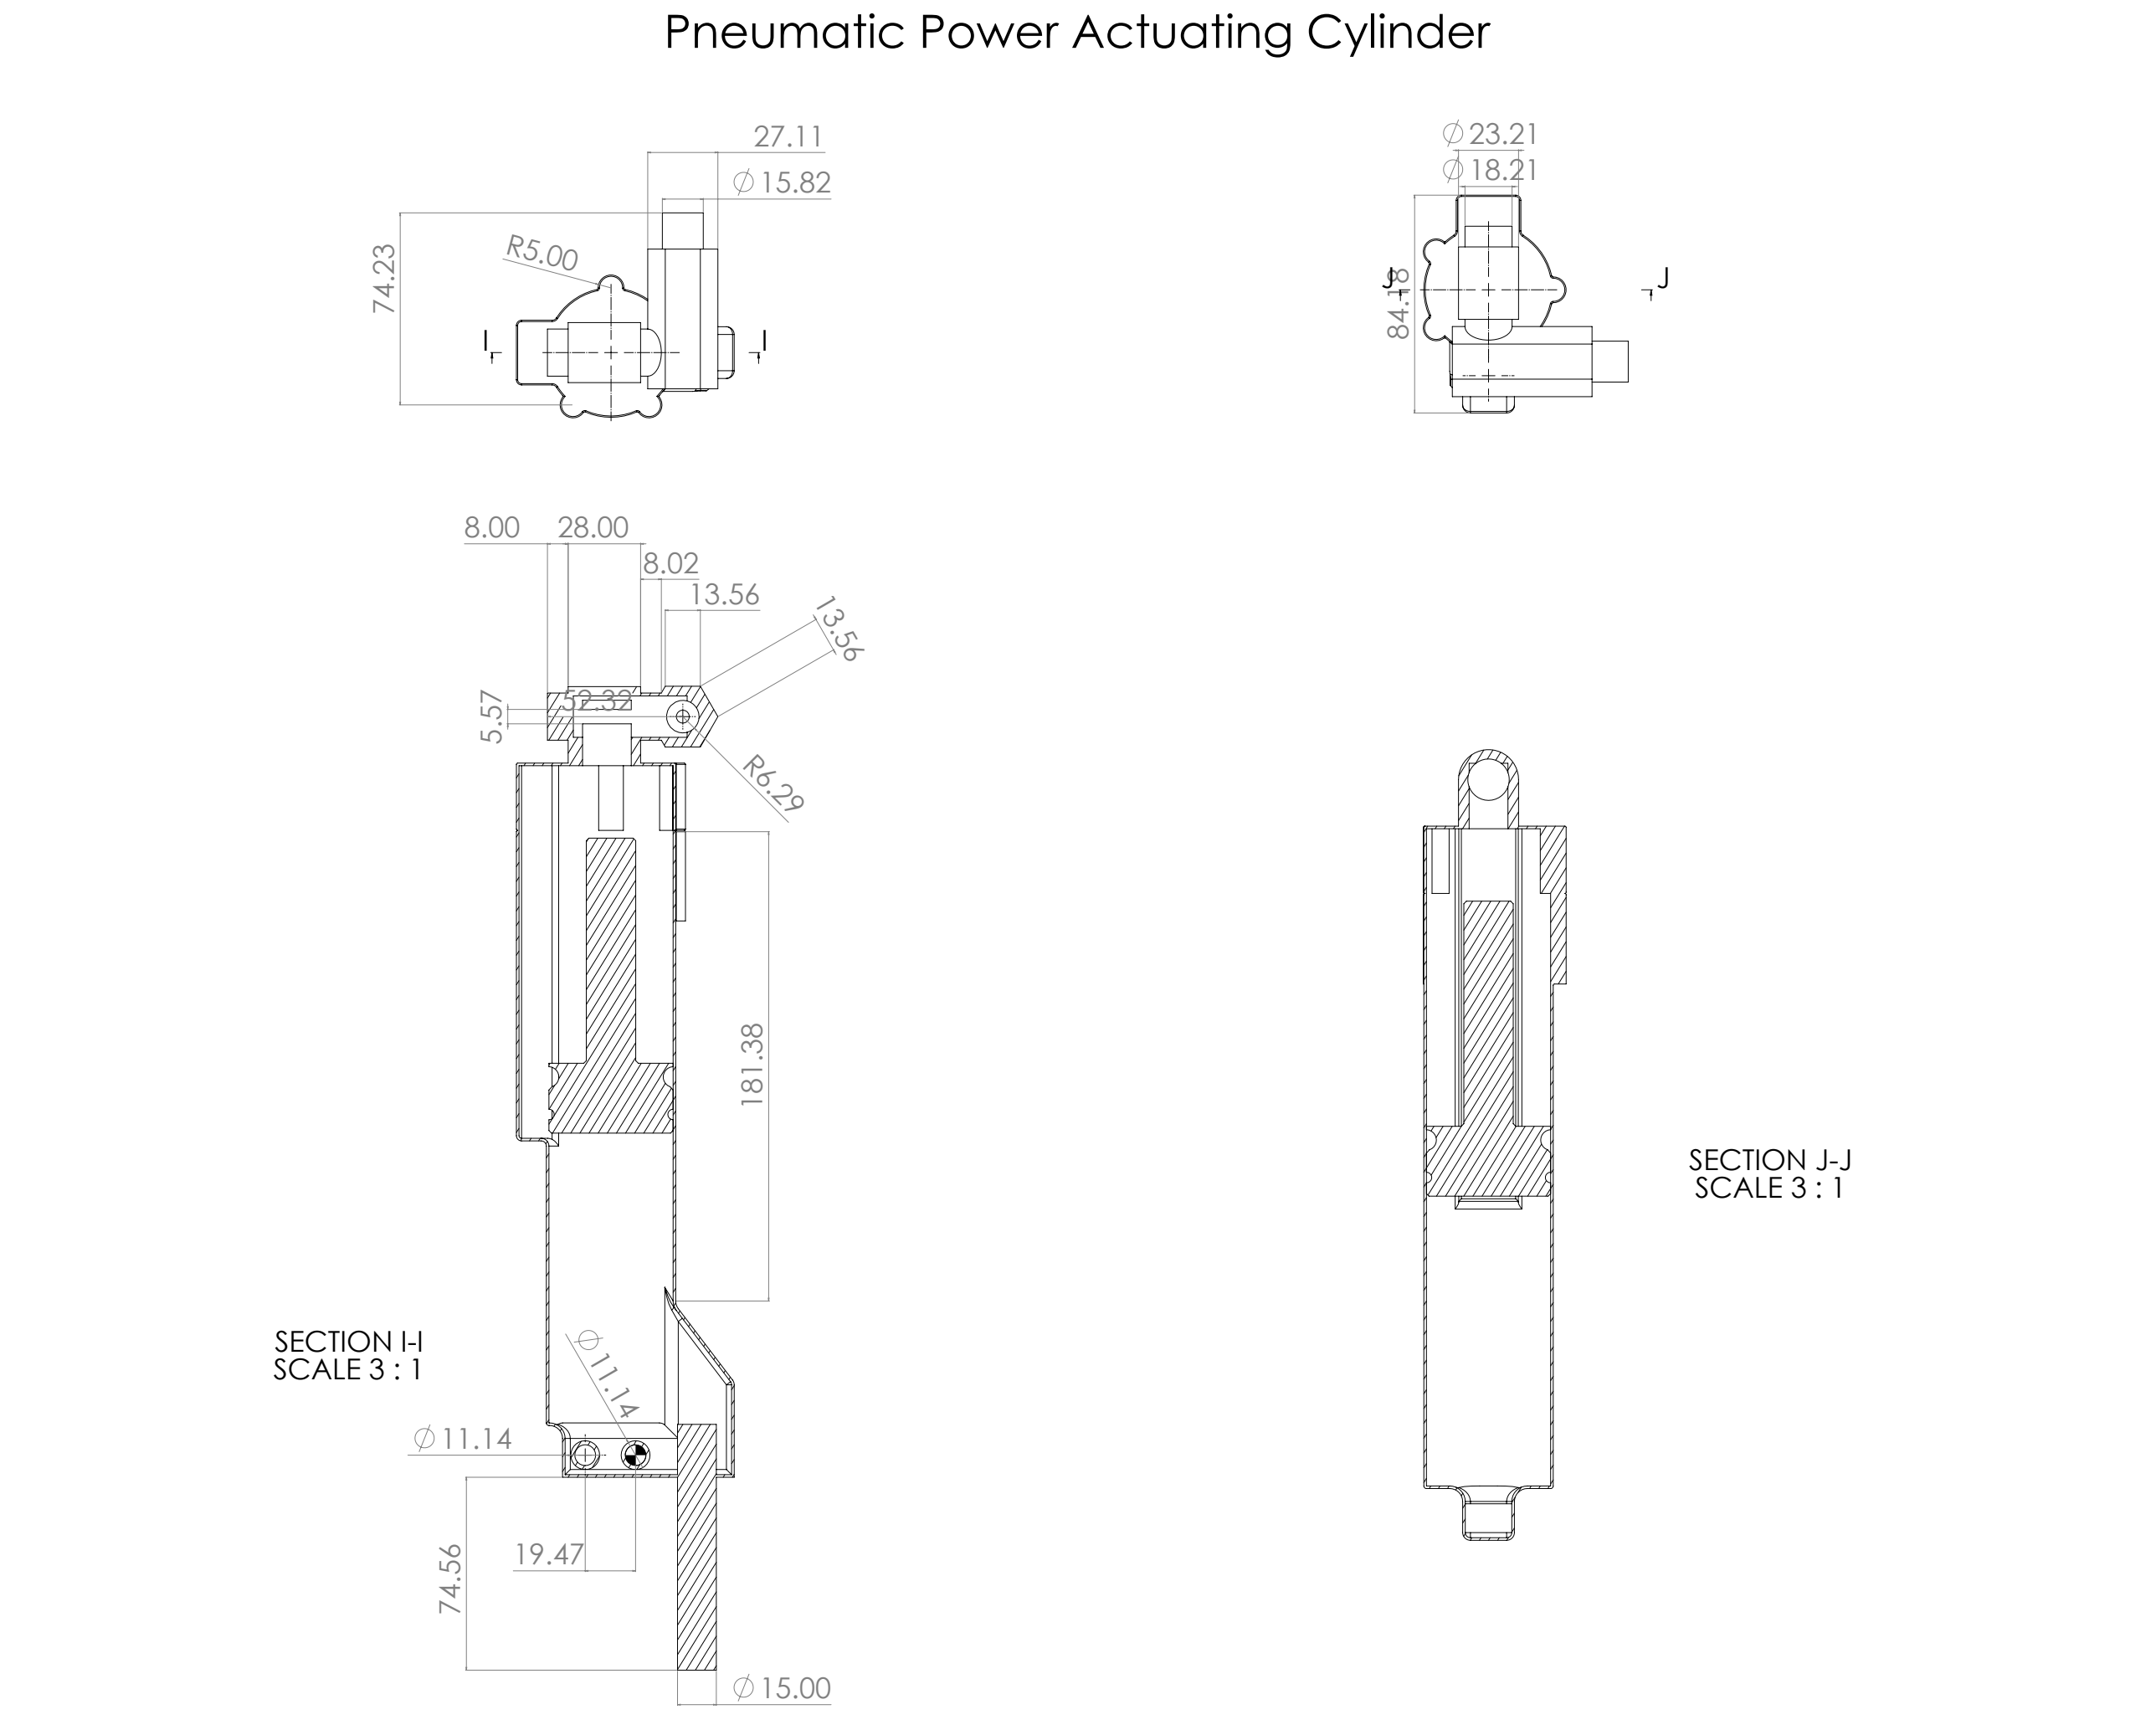
ISO-10303-21;
HEADER;
FILE_DESCRIPTION (('STEP AP214'),
    '1' );
FILE_NAME ('Pneumatic Power Actuating Cylinder.step',
    '2026-10-25T20:52:49',
    ( '' ),
    ( '' ),
    'SwSTEP 2.0',
    'SolidWorks 2025',
    '' );
FILE_SCHEMA (( 'AUTOMOTIVE_DESIGN' ));
ENDSEC;

DATA;
#13=CONICAL_SURFACE ( 'NONE', #77116, 24.00000000000001066, 0.7446590313522313265 ) ;
#19=LINE ( 'NONE', #14705, #54462 ) ;
#22=DIRECTION ( 'NONE',  ( -0.7957555401921980742, -0.6056179655966482667, 0.000000000000000000 ) ) ;
#31=VERTEX_POINT ( 'NONE', #14545 ) ;
#46=DIRECTION ( 'NONE',  ( -0.4999999999999952260, -0.8660254037844413721, 0.000000000000000000 ) ) ;
#47=FACE_OUTER_BOUND ( 'NONE', #78112, .T. ) ;
#48=EDGE_CURVE ( 'NONE', #2640, #65773, #51617, .T. ) ;
#70=VERTEX_POINT ( 'NONE', #796 ) ;
#88=EDGE_LOOP ( 'NONE', ( #36300, #74959 ) ) ;
#89=DIRECTION ( 'NONE',  ( 0.000000000000000000, -0.000000000000000000, 1.000000000000000000 ) ) ;
#92=EDGE_CURVE ( 'NONE', #64177, #39404, #21633, .T. ) ;
#124=CARTESIAN_POINT ( 'NONE',  ( 175.2296996224750103, 275.0000000000000568, 0.000000000000000000 ) ) ;
#125=CARTESIAN_POINT ( 'NONE',  ( 208.4306832106271088, 20.44233620800389772, 0.000000000000000000 ) ) ;
#133=EDGE_CURVE ( 'NONE', #3915, #71428, #47386, .T. ) ;
#135=VERTEX_POINT ( 'NONE', #13608 ) ;
#137=AXIS2_PLACEMENT_3D ( 'NONE', #66421, #57925, #65055 ) ;
#142=ORIENTED_EDGE ( 'NONE', *, *, #90775, .T. ) ;
#150=ORIENTED_EDGE ( 'NONE', *, *, #26082, .T. ) ;
#154=DIRECTION ( 'NONE',  ( 0.000000000000000000, 1.000000000000000000, 0.000000000000000000 ) ) ;
#157=CYLINDRICAL_SURFACE ( 'NONE', #21355, 0.5000000000000004441 ) ;
#172=ORIENTED_EDGE ( 'NONE', *, *, #18686, .T. ) ;
#175=ORIENTED_EDGE ( 'NONE', *, *, #24191, .T. ) ;
#200=VERTEX_POINT ( 'NONE', #71848 ) ;
#203=EDGE_CURVE ( 'NONE', #23354, #33474, #15867, .T. ) ;
#215=DIRECTION ( 'NONE',  ( 0.000000000000000000, 1.000000000000000000, 0.000000000000000000 ) ) ;
#220=CARTESIAN_POINT ( 'NONE',  ( 211.4629471475955427, 32.98517505407394168, 10.00000000000000000 ) ) ;
#226=CARTESIAN_POINT ( 'NONE',  ( 219.8344101925596021, 35.72494958537217968, 7.000000000000000000 ) ) ;
#230=CARTESIAN_POINT ( 'NONE',  ( 201.2509219215139922, 65.09645894978946501, 0.000000000000000000 ) ) ;
#233=DIRECTION ( 'NONE',  ( -0.000000000000000000, 0.000000000000000000, -1.000000000000000000 ) ) ;
#237=CARTESIAN_POINT ( 'NONE',  ( 196.8803347170859865, 73.40565171261609123, -12.49999999999998579 ) ) ;
#250=EDGE_CURVE ( 'NONE', #25460, #78927, #7415, .T. ) ;
#252=ADVANCED_FACE ( 'NONE', ( #16740 ), #65214, .F. ) ;
#266=EDGE_CURVE ( 'NONE', #10377, #27540, #29202, .T. ) ;
#272=AXIS2_PLACEMENT_3D ( 'NONE', #89516, #54022, #33648 ) ;
#291=EDGE_CURVE ( 'NONE', #59112, #73985, #48974, .T. ) ;
#307=VERTEX_POINT ( 'NONE', #19143 ) ;
#308=DIRECTION ( 'NONE',  ( 0.000000000000000000, 0.000000000000000000, -1.000000000000000000 ) ) ;
#309=CARTESIAN_POINT ( 'NONE',  ( 196.7084708347797459, 24.79057925319257194, 12.79847700770043950 ) ) ;
#315=CARTESIAN_POINT ( 'NONE',  ( 209.2565306692229683, 27.88187848093107846, 12.07105558346639462 ) ) ;
#318=DIRECTION ( 'NONE',  ( -0.000000000000000000, -1.000000000000000000, -0.000000000000000000 ) ) ;
#321=ORIENTED_EDGE ( 'NONE', *, *, #79781, .T. ) ;
#322=LINE ( 'NONE', #6506, #611 ) ;
#330=AXIS2_PLACEMENT_3D ( 'NONE', #82535, #75438, #88694 ) ;
#336=CARTESIAN_POINT ( 'NONE',  ( 197.2699694956033341, 291.3106288012165805, -7.550674042187431212 ) ) ;
#337=DIRECTION ( 'NONE',  ( -0.000000000000000000, -1.000000000000000000, -0.000000000000000000 ) ) ;
#339=AXIS2_PLACEMENT_3D ( 'NONE', #18506, #54487, #77693 ) ;
#351=CARTESIAN_POINT ( 'NONE',  ( 152.0879868122481184, 129.8824796955493355, -12.50000000000000178 ) ) ;
#359=CARTESIAN_POINT ( 'NONE',  ( 196.0143093133015384, 42.36571313990103960, 11.99999999999998934 ) ) ;
#376=ORIENTED_EDGE ( 'NONE', *, *, #4713, .F. ) ;
#377=CARTESIAN_POINT ( 'NONE',  ( 0.000000000000000000, 131.0000000000000568, -11.50000000000000000 ) ) ;
#379=CARTESIAN_POINT ( 'NONE',  ( 207.5838500149071706, 29.29481134328564451, 13.58522159759120740 ) ) ;
#390=CARTESIAN_POINT ( 'NONE',  ( 195.6182592083429768, 42.27466702580179714, 12.66657019004900953 ) ) ;
#400=CIRCLE ( 'NONE', #83570, 2.500000000000007550 ) ;
#402=CARTESIAN_POINT ( 'NONE',  ( 210.1640492649794396, 37.84931640281016030, 10.50000000000000000 ) ) ;
#403=AXIS2_PLACEMENT_3D ( 'NONE', #74243, #31178, #30232 ) ;
#404=DIRECTION ( 'NONE',  ( 0.000000000000000000, -1.000000000000000000, 0.000000000000000000 ) ) ;
#409=AXIS2_PLACEMENT_3D ( 'NONE', #74640, #9280, #38163 ) ;
#427=DIRECTION ( 'NONE',  ( -0.000000000000000000, 1.000000000000000000, -0.000000000000000000 ) ) ;
#438=( BOUNDED_SURFACE ( )  B_SPLINE_SURFACE ( 3, 2, ( 
 ( #50320, #50797, #35669 ),
 ( #87224, #29020, #21923 ),
 ( #65495, #15274, #20984 ),
 ( #42745, #29497, #79681 ) ),
 .UNSPECIFIED., .F., .F., .F. ) 
 B_SPLINE_SURFACE_WITH_KNOTS ( ( 4, 4 ),
 ( 3, 3 ),
 ( 0.000000000000000000, 0.0009274969146595095750 ),
 ( 0.000000000000000000, 1.000000000000000000 ),
 .UNSPECIFIED. ) 
 GEOMETRIC_REPRESENTATION_ITEM ( )  RATIONAL_B_SPLINE_SURFACE ( (
 ( 1.000000000000000000, 0.7691239371209215303, 1.000000000000000000),
 ( 1.000000000000000000, 0.7869877059350417481, 1.000000000000000000),
 ( 1.000000000000000000, 0.8014280003973071054, 1.000000000000000000),
 ( 1.000000000000000000, 0.8108476219622873238, 1.000000000000000000) ) ) 
 REPRESENTATION_ITEM ( '' )  SURFACE ( )  );
#443=VERTEX_POINT ( 'NONE', #78317 ) ;
#444=CARTESIAN_POINT ( 'NONE',  ( 156.6537229343953754, 214.8829733828359849, 16.96953521546817001 ) ) ;
#446=( BOUNDED_SURFACE ( )  B_SPLINE_SURFACE ( 3, 2, ( 
 ( #46429, #52604, #66380 ),
 ( #81486, #45029, #45487 ),
 ( #9515, #38403, #9987 ),
 ( #68231, #32242, #60670 ) ),
 .UNSPECIFIED., .F., .F., .F. ) 
 B_SPLINE_SURFACE_WITH_KNOTS ( ( 4, 4 ),
 ( 3, 3 ),
 ( 0.000000000000000000, 0.0009274969146595095750 ),
 ( 0.000000000000000000, 1.000000000000000000 ),
 .UNSPECIFIED. ) 
 GEOMETRIC_REPRESENTATION_ITEM ( )  RATIONAL_B_SPLINE_SURFACE ( (
 ( 1.000000000000000000, 0.7691239371209221964, 1.000000000000000000),
 ( 1.000000000000000000, 0.7869877059350496307, 1.000000000000000000),
 ( 1.000000000000000000, 0.8014280003973005551, 1.000000000000000000),
 ( 1.000000000000000000, 0.8108476219622871017, 1.000000000000000000) ) ) 
 REPRESENTATION_ITEM ( '' )  SURFACE ( )  );
#459=CARTESIAN_POINT ( 'NONE',  ( 219.8344101925596021, 0.000000000000000000, 7.000000000000000000 ) ) ;
#460=DIRECTION ( 'NONE',  ( -0.000000000000000000, -1.000000000000000000, -0.000000000000000000 ) ) ;
#470=EDGE_CURVE ( 'NONE', #443, #38673, #70143, .T. ) ;
#474=AXIS2_PLACEMENT_3D ( 'NONE', #24792, #83000, #69744 ) ;
#477=VECTOR ( 'NONE', #77768, 1000.000000000000000 ) ;
#481=AXIS2_PLACEMENT_3D ( 'NONE', #69178, #53570, #82445 ) ;
#484=VECTOR ( 'NONE', #66979, 1000.000000000000000 ) ;
#485=DIRECTION ( 'NONE',  ( 0.000000000000000000, 0.000000000000000000, -1.000000000000000000 ) ) ;
#488=DIRECTION ( 'NONE',  ( 0.000000000000000000, 1.000000000000000000, 0.000000000000000000 ) ) ;
#495=VECTOR ( 'NONE', #32367, 1000.000000000000000 ) ;
#509=AXIS2_PLACEMENT_3D ( 'NONE', #63054, #5739, #91883 ) ;
#516=CARTESIAN_POINT ( 'NONE',  ( 159.4851178187871312, 15.00000000000000000, 9.000000000000000000 ) ) ;
#527=EDGE_LOOP ( 'NONE', ( #23564, #43969, #29055, #47901 ) ) ;
#533=( NAMED_UNIT ( * ) SI_UNIT ( $, .STERADIAN. ) SOLID_ANGLE_UNIT ( ) );
#536=EDGE_LOOP ( 'NONE', ( #40735, #1250, #34787, #36151 ) ) ;
#539=VECTOR ( 'NONE', #13268, 1000.000000000000000 ) ;
#544=CARTESIAN_POINT ( 'NONE',  ( 186.6539576904058890, 276.0000000000000568, 11.60392986742922616 ) ) ;
#557=VERTEX_POINT ( 'NONE', #91558 ) ;
#558=CARTESIAN_POINT ( 'NONE',  ( 195.4431342809958210, 25.62282010151562162, 12.94565045871722653 ) ) ;
#569=DIRECTION ( 'NONE',  ( -0.7957555401921984073, -0.6056179655966479336, 0.000000000000000000 ) ) ;
#573=DIRECTION ( 'NONE',  ( -1.000000000000000000, 0.000000000000000000, 0.000000000000000000 ) ) ;
#584=EDGE_CURVE ( 'NONE', #89341, #28861, #72351, .T. ) ;
#596=DIRECTION ( 'NONE',  ( 0.000000000000000000, 0.000000000000000000, 1.000000000000000000 ) ) ;
#599=CARTESIAN_POINT ( 'NONE',  ( 195.7618616733231249, 25.17790309710478880, 14.26375052247069597 ) ) ;
#600=DIRECTION ( 'NONE',  ( 0.000000000000000000, 0.000000000000000000, -1.000000000000000000 ) ) ;
#608=EDGE_CURVE ( 'NONE', #87677, #6373, #68742, .T. ) ;
#610=VERTEX_POINT ( 'NONE', #13456 ) ;
#611=VECTOR ( 'NONE', #22104, 1000.000000000000000 ) ;
#617=AXIS2_PLACEMENT_3D ( 'NONE', #50183, #27969, #71997 ) ;
#626=AXIS2_PLACEMENT_3D ( 'NONE', #69064, #4653, #32616 ) ;
#628=VECTOR ( 'NONE', #56195, 1000.000000000000000 ) ;
#629=CARTESIAN_POINT ( 'NONE',  ( 196.6877655503061817, 294.2166337988281839, -7.999911143031724237 ) ) ;
#632=DIRECTION ( 'NONE',  ( 0.000000000000000000, 0.000000000000000000, -1.000000000000000000 ) ) ;
#634=AXIS2_PLACEMENT_3D ( 'NONE', #54460, #69150, #62530 ) ;
#645=TOROIDAL_SURFACE ( 'NONE', #5171, 1.000000000000000000, 0.5000000000000000000 ) ;
#648=ORIENTED_EDGE ( 'NONE', *, *, #78193, .T. ) ;
#676=ORIENTED_EDGE ( 'NONE', *, *, #7722, .F. ) ;
#680=ORIENTED_EDGE ( 'NONE', *, *, #88813, .T. ) ;
#684=AXIS2_PLACEMENT_3D ( 'NONE', #53670, #32361, #85228 ) ;
#690=DIRECTION ( 'NONE',  ( 1.000000000000000000, 0.000000000000000000, -0.000000000000000000 ) ) ;
#693=CIRCLE ( 'NONE', #79306, 1.999999999999988454 ) ;
#696=CARTESIAN_POINT ( 'NONE',  ( 193.9646936176702070, 20.00000000000000000, -15.00000000000000000 ) ) ;
#698=AXIS2_PLACEMENT_3D ( 'NONE', #32787, #46964, #39859 ) ;
#703=CARTESIAN_POINT ( 'NONE',  ( 154.5739546116847407, 19.95362051968588801, 14.09237539257051530 ) ) ;
#706=CARTESIAN_POINT ( 'NONE',  ( 151.2975037349263800, 130.0000000000000568, 12.50000000000000000 ) ) ;
#709=CIRCLE ( 'NONE', #58172, 7.500000000000012434 ) ;
#733=ADVANCED_FACE ( 'NONE', ( #49428 ), #55131, .T. ) ;
#742=EDGE_CURVE ( 'NONE', #34447, #93704, #90736, .T. ) ;
#760=AXIS2_PLACEMENT_3D ( 'NONE', #30344, #9477, #21860 ) ;
#784=CARTESIAN_POINT ( 'NONE',  ( 165.2494399300530290, 8.542400036368780647, 9.000000000000001776 ) ) ;
#793=EDGE_CURVE ( 'NONE', #79410, #22214, #70290, .T. ) ;
#794=DIRECTION ( 'NONE',  ( 0.000000000000000000, 0.000000000000000000, 1.000000000000000000 ) ) ;
#796=CARTESIAN_POINT ( 'NONE',  ( 196.8702642586143270, 40.96915988761478644, 12.42857142857141994 ) ) ;
#800=CARTESIAN_POINT ( 'NONE',  ( 197.0850307134193713, 40.94976125279444545, 10.55987713565813024 ) ) ;
#813=LINE ( 'NONE', #31437, #58161 ) ;
#814=CARTESIAN_POINT ( 'NONE',  ( 201.2104617360081704, 25.32700003806615996, 9.000000000000001776 ) ) ;
#822=DIRECTION ( 'NONE',  ( 0.000000000000000000, 0.000000000000000000, 1.000000000000000000 ) ) ;
#823=DIRECTION ( 'NONE',  ( 1.000000000000000000, 0.000000000000000000, 0.000000000000000000 ) ) ;
#830=DIRECTION ( 'NONE',  ( -0.000000000000000000, -1.000000000000000000, -0.000000000000000000 ) ) ;
#839=PLANE ( 'NONE',  #10916 ) ;
#841=AXIS2_PLACEMENT_3D ( 'NONE', #42069, #7056, #77614 ) ;
#854=CARTESIAN_POINT ( 'NONE',  ( 199.7111327665421072, 66.88064514420912587, 10.01633191836423364 ) ) ;
#856=FACE_OUTER_BOUND ( 'NONE', #12534, .T. ) ;
#867=EDGE_LOOP ( 'NONE', ( #63453, #67407, #86830, #3763 ) ) ;
#878=DIRECTION ( 'NONE',  ( 0.000000000000000000, 0.000000000000000000, -1.000000000000000000 ) ) ;
#882=ORIENTED_EDGE ( 'NONE', *, *, #83721, .T. ) ;
#899=EDGE_CURVE ( 'NONE', #67369, #66900, #57022, .T. ) ;
#900=CARTESIAN_POINT ( 'NONE',  ( 210.2448042458983366, 0.01303144969186963500, -7.291618491801075130 ) ) ;
#907=EDGE_CURVE ( 'NONE', #12419, #67382, #86299, .T. ) ;
#909=EDGE_CURVE ( 'NONE', #57029, #39232, #24135, .T. ) ;
#915=ORIENTED_EDGE ( 'NONE', *, *, #72851, .F. ) ;
#916=CARTESIAN_POINT ( 'NONE',  ( 197.9834613664963001, 18.87240044341482914, -11.15593255764641967 ) ) ;
#930=DIRECTION ( 'NONE',  ( 0.000000000000000000, 1.000000000000000000, 0.000000000000000000 ) ) ;
#938=CARTESIAN_POINT ( 'NONE',  ( 140.6539576904058606, 249.5000000000000568, 12.50000000000000000 ) ) ;
#942=DIRECTION ( 'NONE',  ( 0.000000000000000000, 0.000000000000000000, 1.000000000000000000 ) ) ;
#964=ORIENTED_EDGE ( 'NONE', *, *, #41918, .T. ) ;
#965=PLANE ( 'NONE',  #3028 ) ;
#967=CARTESIAN_POINT ( 'NONE',  ( 175.2296996224750103, 214.5000000000000568, 0.000000000000000000 ) ) ;
#979=CARTESIAN_POINT ( 'NONE',  ( 201.8074164582889125, 62.71404347880360319, -8.782170572880787063 ) ) ;
#980=CARTESIAN_POINT ( 'NONE',  ( 160.5350683151633291, 250.5000000000000568, 20.22542485937379908 ) ) ;
#983=CARTESIAN_POINT ( 'NONE',  ( 193.9153122143737562, 214.9910457053126720, 17.21343741151142481 ) ) ;
#999=EDGE_CURVE ( 'NONE', #46709, #71428, #37410, .T. ) ;
#1003=ORIENTED_EDGE ( 'NONE', *, *, #5970, .F. ) ;
#1009=CARTESIAN_POINT ( 'NONE',  ( 165.0704140682094589, 2.965303559109564890, 10.00000000000000000 ) ) ;
#1014=ADVANCED_FACE ( 'NONE', ( #2837 ), #75763, .T. ) ;
#1017=B_SPLINE_CURVE_WITH_KNOTS ( 'NONE', 3,
 ( #237, #56627, #85477, #93503, #42373, #57546, #29117, #35287 ),
 .UNSPECIFIED., .F., .F.,
 ( 4, 2, 2, 4 ),
 ( -1.794524598959325299E-05, 0.004652435581272471032, 0.006987625994903502377, 0.009322816408534533722 ),
 .UNSPECIFIED. ) ;
#1023=VERTEX_POINT ( 'NONE', #983 ) ;
#1024=CARTESIAN_POINT ( 'NONE',  ( 195.7077576554793836, 26.39544325298913918, 13.66612345222623404 ) ) ;
#1047=DIRECTION ( 'NONE',  ( -1.000000000000000000, 0.000000000000000000, 0.000000000000000000 ) ) ;
#1055=CARTESIAN_POINT ( 'NONE',  ( 198.6746746775679355, 25.20017525016920246, 11.14960445189099225 ) ) ;
#1058=CARTESIAN_POINT ( 'NONE',  ( 195.0811277904325323, 27.27788670632333989, 15.19607843137264602 ) ) ;
#1059=CARTESIAN_POINT ( 'NONE',  ( 156.4851178187871312, 0.000000000000000000, -7.000000000000000888 ) ) ;
#1068=EDGE_LOOP ( 'NONE', ( #54068, #62858, #68288, #37860 ) ) ;
#1069=CARTESIAN_POINT ( 'NONE',  ( 175.2296996224749250, 276.0000000000000568, -24.99999999999999289 ) ) ;
#1072=DIRECTION ( 'NONE',  ( 0.000000000000000000, 1.000000000000000000, 0.000000000000000000 ) ) ;
#1084=CARTESIAN_POINT ( 'NONE',  ( 201.9208557708175249, 300.1658636863270431, -5.053462443409009630 ) ) ;
#1087=CARTESIAN_POINT ( 'NONE',  ( 175.2296996224750103, 250.5000000000000568, 0.000000000000000000 ) ) ;
#1101=ORIENTED_EDGE ( 'NONE', *, *, #12784, .T. ) ;
#1104=EDGE_LOOP ( 'NONE', ( #42911, #32160, #59830, #16502 ) ) ;
#1109=EDGE_CURVE ( 'NONE', #44168, #80534, #22737, .T. ) ;
#1131=ORIENTED_EDGE ( 'NONE', *, *, #65065, .F. ) ;
#1134=ADVANCED_FACE ( 'NONE', ( #58749 ), #55660, .T. ) ;
#1135=VERTEX_POINT ( 'NONE', #59209 ) ;
#1146=DIRECTION ( 'NONE',  ( 0.000000000000000000, 1.000000000000000000, 0.000000000000000000 ) ) ;
#1151=CARTESIAN_POINT ( 'NONE',  ( 140.6539576904058606, 275.0000000000000568, -10.49999999999999822 ) ) ;
#1157=DIRECTION ( 'NONE',  ( -0.000000000000000000, -0.000000000000000000, -1.000000000000000000 ) ) ;
#1160=CARTESIAN_POINT ( 'NONE',  ( 194.7173632872394649, 19.95192844427760193, 14.18452691302933033 ) ) ;
#1162=LINE ( 'NONE', #80229, #54661 ) ;
#1168=CARTESIAN_POINT ( 'NONE',  ( 180.2288731078812702, 214.9910457053126720, -24.90909090909092782 ) ) ;
#1176=VERTEX_POINT ( 'NONE', #23212 ) ;
#1180=CARTESIAN_POINT ( 'NONE',  ( 169.8384340989974532, 214.5000000000000568, -24.41176470588233727 ) ) ;
#1197=ADVANCED_FACE ( 'NONE', ( #88535 ), #31719, .T. ) ;
#1219=EDGE_CURVE ( 'NONE', #20475, #31737, #23684, .T. ) ;
#1237=ORIENTED_EDGE ( 'NONE', *, *, #74557, .F. ) ;
#1244=CARTESIAN_POINT ( 'NONE',  ( 209.0514133012270861, 29.56734752687822620, 14.78224109794551033 ) ) ;
#1250=ORIENTED_EDGE ( 'NONE', *, *, #18442, .F. ) ;
#1251=CARTESIAN_POINT ( 'NONE',  ( 152.4536156746142410, 250.0000000000000568, -11.99999999999999112 ) ) ;
#1264=CARTESIAN_POINT ( 'NONE',  ( 196.7806748523260012, 250.5000000000000568, -12.67104836398113399 ) ) ;
#1272=CARTESIAN_POINT ( 'NONE',  ( 193.9646936176702070, 21.00000000000000000, -15.00000000000000000 ) ) ;
#1273=CARTESIAN_POINT ( 'NONE',  ( 175.2296996224749250, 250.5000000000000568, -24.99999999999999289 ) ) ;
#1280=LINE ( 'NONE', #2221, #36777 ) ;
#1287=CARTESIAN_POINT ( 'NONE',  ( 196.5738014817347050, 41.11195847892590649, 11.18394375856346556 ) ) ;
#1290=FACE_OUTER_BOUND ( 'NONE', #52683, .T. ) ;
#1303=ORIENTED_EDGE ( 'NONE', *, *, #24438, .F. ) ;
#1306=DIRECTION ( 'NONE',  ( 0.000000000000000000, 0.000000000000000000, 1.000000000000000000 ) ) ;
#1326=CARTESIAN_POINT ( 'NONE',  ( 152.4536156746142410, 275.0000000000000568, -11.50000000000000355 ) ) ;
#1331=EDGE_LOOP ( 'NONE', ( #25766, #6601, #5992, #88463 ) ) ;
#1347=DIRECTION ( 'NONE',  ( 0.000000000000000000, 1.000000000000000000, 0.000000000000000000 ) ) ;
#1349=DIRECTION ( 'NONE',  ( 0.000000000000000000, 0.000000000000000000, -1.000000000000000000 ) ) ;
#1361=ORIENTED_EDGE ( 'NONE', *, *, #30936, .F. ) ;
#1367=EDGE_CURVE ( 'NONE', #81908, #50747, #52092, .T. ) ;
#1378=CARTESIAN_POINT ( 'NONE',  ( 156.4947056272798136, 19.99999999999999645, -15.00000000000000711 ) ) ;
#1386=CARTESIAN_POINT ( 'NONE',  ( 204.7786681169002350, 32.98517505407394168, 10.00000000000000000 ) ) ;
#1403=CARTESIAN_POINT ( 'NONE',  ( 197.8477145984406889, 64.61450673763175701, -7.741079165001063522 ) ) ;
#1410=VECTOR ( 'NONE', #49510, 1000.000000000000000 ) ;
#1413=ORIENTED_EDGE ( 'NONE', *, *, #64946, .T. ) ;
#1414=DIRECTION ( 'NONE',  ( 0.000000000000000000, 0.000000000000000000, 1.000000000000000000 ) ) ;
#1417=DIRECTION ( 'NONE',  ( 0.000000000000000000, 1.000000000000000000, 0.000000000000000000 ) ) ;
#1421=ADVANCED_FACE ( 'NONE', ( #16119 ), #24606, .F. ) ;
#1431=DIRECTION ( 'NONE',  ( 0.000000000000000000, 0.000000000000000000, 1.000000000000000000 ) ) ;
#1443=VERTEX_POINT ( 'NONE', #82370 ) ;
#1450=ORIENTED_EDGE ( 'NONE', *, *, #68389, .T. ) ;
#1451=VERTEX_POINT ( 'NONE', #73871 ) ;
#1470=VERTEX_POINT ( 'NONE', #17520 ) ;
#1476=AXIS2_PLACEMENT_3D ( 'NONE', #8968, #1414, #22268 ) ;
#1482=B_SPLINE_CURVE_WITH_KNOTS ( 'NONE', 3,
 ( #10660, #39516, #23489, #52356, #74608, #10190, #31066, #9737, #82632, #82167 ),
 .UNSPECIFIED., .F., .F.,
 ( 4, 2, 2, 2, 4 ),
 ( -1.872485596898890801E-05, 0.002374103250644057396, 0.004766931357257103534, 0.007159759463870149672, 0.009552587570483194943 ),
 .UNSPECIFIED. ) ;
#1496=CARTESIAN_POINT ( 'NONE',  ( 194.3475392320528385, 26.68743749201679805, 14.50895590765962240 ) ) ;
#1502=DIRECTION ( 'NONE',  ( -0.000000000000000000, 0.000000000000000000, -1.000000000000000000 ) ) ;
#1508=LINE ( 'NONE', #59764, #45796 ) ;
#1518=CARTESIAN_POINT ( 'NONE',  ( 200.4551663813218170, 64.49084098419280053, 0.000000000000000000 ) ) ;
#1524=EDGE_CURVE ( 'NONE', #92711, #90042, #92671, .T. ) ;
#1533=( BOUNDED_CURVE ( )  B_SPLINE_CURVE ( 3, ( #22098, #93125, #56710, #43398 ),
 .UNSPECIFIED., .F., .F. ) 
 B_SPLINE_CURVE_WITH_KNOTS ( ( 4, 4 ),
 ( 1.570796326794895004, 2.004620063563923082 ),
 .UNSPECIFIED. ) 
 CURVE ( )  GEOMETRIC_REPRESENTATION_ITEM ( )  RATIONAL_B_SPLINE_CURVE ( ( 1.000000000000000000, 0.9843778111405747655, 0.9843778111405747655, 1.000000000000000000 ) ) 
 REPRESENTATION_ITEM ( '' )  );
#1535=CARTESIAN_POINT ( 'NONE',  ( 155.8055003384388897, 17.52828139914081618, 8.087387968559804463 ) ) ;
#1536=DIRECTION ( 'NONE',  ( -1.000000000000000000, 0.000000000000000000, 0.000000000000000000 ) ) ;
#1537=AXIS2_PLACEMENT_3D ( 'NONE', #11772, #17497, #68618 ) ;
#1542=AXIS2_PLACEMENT_3D ( 'NONE', #35545, #85251, #20398 ) ;
#1554=ORIENTED_EDGE ( 'NONE', *, *, #13930, .F. ) ;
#1557=EDGE_LOOP ( 'NONE', ( #41598, #34259, #35254, #4428 ) ) ;
#1567=VERTEX_POINT ( 'NONE', #67252 ) ;
#1585=VERTEX_POINT ( 'NONE', #11336 ) ;
#1586=CARTESIAN_POINT ( 'NONE',  ( 158.3977298502311157, 18.03393767897202693, 9.815540976419818264 ) ) ;
#1609=CIRCLE ( 'NONE', #49999, 0.5000000000000004441 ) ;
#1612=CYLINDRICAL_SURFACE ( 'NONE', #21692, 24.00000000000000355 ) ;
#1616=CARTESIAN_POINT ( 'NONE',  ( 195.3965999132940397, 19.72393862741004611, 13.34571198792791868 ) ) ;
#1618=DIRECTION ( 'NONE',  ( -0.000000000000000000, -1.000000000000000000, 0.000000000000000000 ) ) ;
#1620=DIRECTION ( 'NONE',  ( -1.000000000000000000, 0.000000000000000000, -0.000000000000000000 ) ) ;
#1624=CARTESIAN_POINT ( 'NONE',  ( 188.2019740231993410, 44.81720372851549428, 10.50000000000000000 ) ) ;
#1631=ADVANCED_FACE ( 'NONE', ( #76207 ), #91321, .T. ) ;
#1634=ORIENTED_EDGE ( 'NONE', *, *, #50049, .T. ) ;
#1638=DIRECTION ( 'NONE',  ( -1.000000000000000000, 0.000000000000000000, 0.000000000000000000 ) ) ;
#1641=CARTESIAN_POINT ( 'NONE',  ( 208.6470931340251695, 37.28147638844021117, 12.02381566707520300 ) ) ;
#1670=EDGE_LOOP ( 'NONE', ( #9116, #72630, #35817, #56102 ) ) ;
#1671=EDGE_CURVE ( 'NONE', #70513, #36421, #78434, .T. ) ;
#1682=CIRCLE ( 'NONE', #34945, 24.50000000000000355 ) ;
#1695=CARTESIAN_POINT ( 'NONE',  ( 196.8803347170859865, 20.19615242270661426, 12.49999999999999289 ) ) ;
#1700=CYLINDRICAL_SURFACE ( 'NONE', #14009, 2.000000000000000888 ) ;
#1701=DIRECTION ( 'NONE',  ( -0.000000000000000000, -1.000000000000000000, -0.000000000000000000 ) ) ;
#1707=CARTESIAN_POINT ( 'NONE',  ( 208.6208076322478746, 32.98517505407394168, 10.00000000000000000 ) ) ;
#1730=CARTESIAN_POINT ( 'NONE',  ( 209.7513585654923816, 282.2246705312486483, -40.00000000000000711 ) ) ;
#1735=CARTESIAN_POINT ( 'NONE',  ( 199.0061125298537377, 250.5000000000000568, -7.725424859374024678 ) ) ;
#1737=EDGE_CURVE ( 'NONE', #23799, #17402, #5377, .T. ) ;
#1739=FACE_OUTER_BOUND ( 'NONE', #32338, .T. ) ;
#1746=CARTESIAN_POINT ( 'NONE',  ( 197.3748232817348764, 249.5000000000000568, -12.45182892472558756 ) ) ;
#1749=DIRECTION ( 'NONE',  ( 0.000000000000000000, 0.000000000000000000, 1.000000000000000000 ) ) ;
#1751=AXIS2_PLACEMENT_3D ( 'NONE', #1735, #81729, #16877 ) ;
#1761=EDGE_CURVE ( 'NONE', #65093, #10127, #91797, .T. ) ;
#1762=EDGE_CURVE ( 'NONE', #5855, #73562, #18431, .T. ) ;
#1763=B_SPLINE_CURVE_WITH_KNOTS ( 'NONE', 3,
 ( #706, #29590, #44697, #7785, #81151, #43765 ),
 .UNSPECIFIED., .F., .F.,
 ( 4, 2, 4 ),
 ( 0.000000000000000000, 0.0005961816168538936920, 0.001192363233707787384 ),
 .UNSPECIFIED. ) ;
#1769=DIRECTION ( 'NONE',  ( 0.000000000000000000, 0.000000000000000000, 1.000000000000000000 ) ) ;
#1778=ORIENTED_EDGE ( 'NONE', *, *, #19590, .F. ) ;
#1783=EDGE_CURVE ( 'NONE', #27568, #44950, #62480, .T. ) ;
#1790=DIRECTION ( 'NONE',  ( -0.000000000000000000, -0.000000000000000000, -1.000000000000000000 ) ) ;
#1791=DIRECTION ( 'NONE',  ( 0.000000000000000000, 0.000000000000000000, -1.000000000000000000 ) ) ;
#1795=ORIENTED_EDGE ( 'NONE', *, *, #45672, .T. ) ;
#1809=DIRECTION ( 'NONE',  ( -0.7453559924999200170, 0.000000000000000000, -0.6666666666666777319 ) ) ;
#1812=FACE_OUTER_BOUND ( 'NONE', #17774, .T. ) ;
#1813=CIRCLE ( 'NONE', #47133, 7.999911143031724237 ) ;
#1814=CARTESIAN_POINT ( 'NONE',  ( 210.6911334572095598, 1.334076891925523281E-16, -7.166221634559009956 ) ) ;
#1815=VECTOR ( 'NONE', #7572, 1000.000000000000000 ) ;
#1823=CARTESIAN_POINT ( 'NONE',  ( 201.2104617360081704, 15.00000000000000000, 10.00000000000000000 ) ) ;
#1827=ORIENTED_EDGE ( 'NONE', *, *, #52934, .F. ) ;
#1828=VERTEX_POINT ( 'NONE', #68169 ) ;
#1829=CARTESIAN_POINT ( 'NONE',  ( 196.8803347170860150, 20.19615242270657163, -12.49999999999990941 ) ) ;
#1831=ADVANCED_FACE ( 'NONE', ( #40648 ), #55492, .T. ) ;
#1844=CARTESIAN_POINT ( 'NONE',  ( 197.1123855246549113, 19.09807621135331601, -10.09807621135331246 ) ) ;
#1879=FACE_OUTER_BOUND ( 'NONE', #84407, .T. ) ;
#1883=CARTESIAN_POINT ( 'NONE',  ( 175.2296996224750103, 275.0000000000000568, 0.000000000000000000 ) ) ;
#1886=MECHANICAL_DESIGN_GEOMETRIC_PRESENTATION_REPRESENTATION('',(#88040),#32101);
#1889=AXIS2_PLACEMENT_3D ( 'NONE', #75536, #46175, #8792 ) ;
#1892=ADVANCED_FACE ( 'NONE', ( #39254 ), #63083, .T. ) ;
#1895=ORIENTED_EDGE ( 'NONE', *, *, #3875, .T. ) ;
#1899=EDGE_CURVE ( 'NONE', #23580, #14315, #57008, .T. ) ;
#1903=DIRECTION ( 'NONE',  ( 0.000000000000000000, 0.000000000000000000, 1.000000000000000000 ) ) ;
#1937=DIRECTION ( 'NONE',  ( -1.000000000000000000, 0.000000000000000000, 0.000000000000000000 ) ) ;
#1944=AXIS2_PLACEMENT_3D ( 'NONE', #34809, #13512, #28646 ) ;
#1952=EDGE_CURVE ( 'NONE', #64179, #15573, #34061, .T. ) ;
#1954=EDGE_CURVE ( 'NONE', #44950, #76130, #84195, .T. ) ;
#1955=AXIS2_PLACEMENT_3D ( 'NONE', #93178, #10133, #31007 ) ;
#1966=DIRECTION ( 'NONE',  ( -0.000000000000000000, -1.000000000000000000, -0.000000000000000000 ) ) ;
#1972=CARTESIAN_POINT ( 'NONE',  ( 165.2494399300530290, 8.542400036368780647, 10.00000000000000000 ) ) ;
#1978=CARTESIAN_POINT ( 'NONE',  ( 158.6539576904058606, 276.0000000000000568, -11.60392986742922439 ) ) ;
#1979=CARTESIAN_POINT ( 'NONE',  ( 219.8344101925596021, 3.000000000000000000, -9.000000000000001776 ) ) ;
#1988=VERTEX_POINT ( 'NONE', #39717 ) ;
#1992=DIRECTION ( 'NONE',  ( -0.000000000000000000, -1.000000000000000000, -0.000000000000000000 ) ) ;
#2003=AXIS2_PLACEMENT_3D ( 'NONE', #71866, #337, #86031 ) ;
#2005=CARTESIAN_POINT ( 'NONE',  ( 156.3466120839441089, 16.19322481500840993, 7.221609175748572973 ) ) ;
#2009=VECTOR ( 'NONE', #39902, 1000.000000000000000 ) ;
#2023=EDGE_CURVE ( 'NONE', #3915, #44324, #61085, .T. ) ;
#2040=ORIENTED_EDGE ( 'NONE', *, *, #56462, .T. ) ;
#2051=ORIENTED_EDGE ( 'NONE', *, *, #5681, .F. ) ;
#2055=VECTOR ( 'NONE', #50209, 1000.000000000000000 ) ;
#2059=ORIENTED_EDGE ( 'NONE', *, *, #38620, .T. ) ;
#2060=CARTESIAN_POINT ( 'NONE',  ( 157.4471379844591752, 15.78783268421836183, 9.037979834337678042 ) ) ;
#2063=VERTEX_POINT ( 'NONE', #61546 ) ;
#2080=CARTESIAN_POINT ( 'NONE',  ( 207.8229135343381131, 36.37371623600424186, 14.86900317285956064 ) ) ;
#2088=DIRECTION ( 'NONE',  ( 0.000000000000000000, 1.000000000000000000, 0.000000000000000000 ) ) ;
#2090=AXIS2_PLACEMENT_3D ( 'NONE', #30133, #58563, #59492 ) ;
#2094=DIRECTION ( 'NONE',  ( 0.000000000000000000, 0.000000000000000000, 1.000000000000000000 ) ) ;
#2110=AXIS2_PLACEMENT_3D ( 'NONE', #15492, #87900, #51930 ) ;
#2114=CYLINDRICAL_SURFACE ( 'NONE', #34879, 3.000000000000000888 ) ;
#2117=CARTESIAN_POINT ( 'NONE',  ( 170.4537599243631405, 250.0000000000000568, -23.51999999999999602 ) ) ;
#2121=VECTOR ( 'NONE', #87459, 1000.000000000000000 ) ;
#2135=DIRECTION ( 'NONE',  ( 0.000000000000000000, 1.000000000000000000, -0.000000000000000000 ) ) ;
#2147=ORIENTED_EDGE ( 'NONE', *, *, #33369, .F. ) ;
#2155=DIRECTION ( 'NONE',  ( 0.000000000000000000, 0.000000000000000000, 1.000000000000000000 ) ) ;
#2156=CIRCLE ( 'NONE', #21833, 25.50000000000000355 ) ;
#2164=CIRCLE ( 'NONE', #17308, 0.4999999999999922839 ) ;
#2170=VERTEX_POINT ( 'NONE', #46370 ) ;
#2180=DIRECTION ( 'NONE',  ( 0.000000000000000000, 1.000000000000000000, 0.000000000000000000 ) ) ;
#2181=CARTESIAN_POINT ( 'NONE',  ( 155.7140808774800007, 21.00000000000000000, 15.62500000000000000 ) ) ;
#2184=AXIS2_PLACEMENT_3D ( 'NONE', #63537, #78191, #92363 ) ;
#2188=CARTESIAN_POINT ( 'NONE',  ( 200.1258905644044432, 39.98499045671346153, 10.50000000000114753 ) ) ;
#2203=FACE_OUTER_BOUND ( 'NONE', #28399, .T. ) ;
#2212=CARTESIAN_POINT ( 'NONE',  ( 175.2296996224750103, 142.2541816238762920, 0.000000000000000000 ) ) ;
#2213=DIRECTION ( 'NONE',  ( 0.000000000000000000, 1.000000000000000000, 0.000000000000000000 ) ) ;
#2221=CARTESIAN_POINT ( 'NONE',  ( 201.2104617360081704, 0.000000000000000000, 10.00000000000000000 ) ) ;
#2232=CARTESIAN_POINT ( 'NONE',  ( 200.6103193995254230, 275.5000000000000568, -2.464576988612312114 ) ) ;
#2242=CIRCLE ( 'NONE', #50642, 2.999999999999999556 ) ;
#2247=CARTESIAN_POINT ( 'NONE',  ( 198.0748556046041244, 67.35408903922716206, 11.09505092893674139 ) ) ;
#2259=AXIS2_PLACEMENT_3D ( 'NONE', #79399, #14535, #43390 ) ;
#2261=ORIENTED_EDGE ( 'NONE', *, *, #4649, .T. ) ;
#2262=DIRECTION ( 'NONE',  ( -0.000000000000000000, -1.000000000000000000, -0.000000000000000000 ) ) ;
#2294=CARTESIAN_POINT ( 'NONE',  ( 180.2262870919856823, 214.9642003054772488, -24.76688354601323283 ) ) ;
#2303=CARTESIAN_POINT ( 'NONE',  ( 207.3561592308186334, 36.17070937851315193, 14.95737379494689456 ) ) ;
#2308=VERTEX_POINT ( 'NONE', #13233 ) ;
#2309=CARTESIAN_POINT ( 'NONE',  ( 199.1517898866434848, 16.71555987447352720, -10.28330198088200120 ) ) ;
#2312=ADVANCED_FACE ( 'NONE', ( #65297 ), #79334, .T. ) ;
#2313=ADVANCED_FACE ( 'NONE', ( #57710 ), #13689, .T. ) ;
#2345=B_SPLINE_CURVE_WITH_KNOTS ( 'NONE', 3,
 ( #61003, #39638, #53881, #91241, #19759, #70446, #11261, #68563, #40573, #69029, #83679, #25010, #91717, #55294, #18841, #47698, #11719, #89848 ),
 .UNSPECIFIED., .F., .F.,
 ( 4, 2, 2, 2, 2, 2, 2, 2, 4 ),
 ( 0.000000000000000000, 0.0005979543124017953383, 0.001195908624803590677, 0.001793862937205386015, 0.002391817249607181353, 0.002989771562008976691, 0.003587725874410772030, 0.004185680186812567802, 0.004783634499214362706 ),
 .UNSPECIFIED. ) ;
#2363=ORIENTED_EDGE ( 'NONE', *, *, #88613, .F. ) ;
#2364=CARTESIAN_POINT ( 'NONE',  ( 200.2349812190172713, 66.43136063442170780, -7.741079165001061746 ) ) ;
#2367=DIRECTION ( 'NONE',  ( 0.000000000000000000, 0.000000000000000000, 1.000000000000000000 ) ) ;
#2375=ORIENTED_EDGE ( 'NONE', *, *, #74127, .F. ) ;
#2378=CARTESIAN_POINT ( 'NONE',  ( 214.2238915819278589, 32.98517505407394168, 9.000000000000001776 ) ) ;
#2380=CARTESIAN_POINT ( 'NONE',  ( 196.0742305401642511, 73.02742819586271139, 11.89621339062204264 ) ) ;
#2383=CARTESIAN_POINT ( 'NONE',  ( 175.2296996224750103, 247.0000000000001137, -8.550761578869359170 ) ) ;
#2384=PRODUCT_DEFINITION_FORMATION_WITH_SPECIFIED_SOURCE ( 'ANY', '', #44255, .NOT_KNOWN. ) ;
#2407=CARTESIAN_POINT ( 'NONE',  ( 189.9243309297870610, 215.0000000000000568, 25.22542485937348644 ) ) ;
#2418=ORIENTED_EDGE ( 'NONE', *, *, #35543, .T. ) ;
#2419=CARTESIAN_POINT ( 'NONE',  ( 175.2296996224750103, 133.0000000000000000, 0.000000000000000000 ) ) ;
#2428=CARTESIAN_POINT ( 'NONE',  ( 208.0521033162707738, 35.78478885999048487, 14.36581762243483773 ) ) ;
#2434=ADVANCED_FACE ( 'NONE', ( #42541 ), #63901, .T. ) ;
#2438=ADVANCED_FACE ( 'NONE', ( #27420 ), #34527, .T. ) ;
#2442=CYLINDRICAL_SURFACE ( 'NONE', #62544, 2.842139515347646750 ) ;
#2449=CYLINDRICAL_SURFACE ( 'NONE', #86484, 4.000000000000003553 ) ;
#2453=CARTESIAN_POINT ( 'NONE',  ( 200.4566814582243808, 25.65177970828076681, 10.50000000000112799 ) ) ;
#2456=CARTESIAN_POINT ( 'NONE',  ( 200.3284360491938116, 214.9642003054772488, -2.901350841306745476 ) ) ;
#2466=VERTEX_POINT ( 'NONE', #402 ) ;
#2467=CARTESIAN_POINT ( 'NONE',  ( 200.4551663813218170, 64.49084098419280053, 2.617322427804800622 ) ) ;
#2482=CARTESIAN_POINT ( 'NONE',  ( 0.000000000000000000, 0.000000000000000000, 10.00000000000000000 ) ) ;
#2485=DIRECTION ( 'NONE',  ( -0.6056179655966483777, 0.7957555401921979632, -0.000000000000000000 ) ) ;
#2498=EDGE_LOOP ( 'NONE', ( #7623, #46944, #48481, #11345, #33708, #19609, #82707 ) ) ;
#2501=ORIENTED_EDGE ( 'NONE', *, *, #85025, .T. ) ;
#2508=ADVANCED_FACE ( 'NONE', ( #7499 ), #66273, .F. ) ;
#2512=EDGE_LOOP ( 'NONE', ( #77006, #1795, #22729, #21511 ) ) ;
#2523=ORIENTED_EDGE ( 'NONE', *, *, #63231, .F. ) ;
#2530=ORIENTED_EDGE ( 'NONE', *, *, #24991, .T. ) ;
#2531=FACE_OUTER_BOUND ( 'NONE', #25162, .T. ) ;
#2535=VERTEX_POINT ( 'NONE', #9822 ) ;
#2547=CYLINDRICAL_SURFACE ( 'NONE', #81948, 2.000000000000010658 ) ;
#2558=CARTESIAN_POINT ( 'NONE',  ( 204.6539576904058606, 287.9062406767683910, -59.00000000000003553 ) ) ;
#2563=CARTESIAN_POINT ( 'NONE',  ( 155.0786878258419392, 18.48484813926942749, -9.250287988715951926 ) ) ;
#2573=AXIS2_PLACEMENT_3D ( 'NONE', #3290, #26948, #69567 ) ;
#2585=CARTESIAN_POINT ( 'NONE',  ( 175.2296996224750103, 133.0000000000000000, 24.00000000000001066 ) ) ;
#2603=DIRECTION ( 'NONE',  ( 0.000000000000000000, 0.000000000000000000, -1.000000000000000000 ) ) ;
#2609=ADVANCED_FACE ( 'NONE', ( #60040, #80389 ), #58637, .T. ) ;
#2612=EDGE_CURVE ( 'NONE', #10377, #82490, #8425, .T. ) ;
#2634=ORIENTED_EDGE ( 'NONE', *, *, #56503, .T. ) ;
#2640=VERTEX_POINT ( 'NONE', #51973 ) ;
#2641=CARTESIAN_POINT ( 'NONE',  ( 197.1402318696357270, 70.11481179788400198, -10.20567219414501992 ) ) ;
#2647=CARTESIAN_POINT ( 'NONE',  ( 150.7110049404234644, 21.00000000139189638, -5.101169899787367790 ) ) ;
#2652=CARTESIAN_POINT ( 'NONE',  ( 197.4027394742815886, 40.84896208771629489, 12.00000000000000711 ) ) ;
#2720=EDGE_LOOP ( 'NONE', ( #34758, #77144, #38820, #57265 ) ) ;
#2735=ORIENTED_EDGE ( 'NONE', *, *, #52504, .T. ) ;
#2751=DIRECTION ( 'NONE',  ( 0.9531768234071978929, -0.3024135303179465994, 1.424463645888277034E-13 ) ) ;
#2752=CARTESIAN_POINT ( 'NONE',  ( 200.4551663813218170, 64.49084098419280053, 0.000000000000000000 ) ) ;
#2760=CARTESIAN_POINT ( 'NONE',  ( 206.7809450508160865, 35.77530089738195329, 15.00000000000000178 ) ) ;
#2763=ORIENTED_EDGE ( 'NONE', *, *, #44799, .F. ) ;
#2770=VECTOR ( 'NONE', #13795, 1000.000000000000000 ) ;
#2779=CARTESIAN_POINT ( 'NONE',  ( 156.4851178187871312, 1.000000000000000000, -7.000000000000000888 ) ) ;
#2791=CARTESIAN_POINT ( 'NONE',  ( 138.6539576904058606, 250.5000000000000568, -10.49999999999999822 ) ) ;
#2793=DIRECTION ( 'NONE',  ( 0.000000000000000000, 0.000000000000000000, -1.000000000000000000 ) ) ;
#2803=DIRECTION ( 'NONE',  ( 0.9764705882352960886, 0.000000000000000000, -0.2156506209390900708 ) ) ;
#2808=EDGE_CURVE ( 'NONE', #31000, #20790, #31154, .T. ) ;
#2812=ADVANCED_FACE ( 'NONE', ( #59099 ), #42773, .T. ) ;
#2815=ORIENTED_EDGE ( 'NONE', *, *, #63406, .F. ) ;
#2816=DIRECTION ( 'NONE',  ( 0.000000000000000000, 1.000000000000000000, 0.000000000000000000 ) ) ;
#2819=LINE ( 'NONE', #65859, #32252 ) ;
#2830=CARTESIAN_POINT ( 'NONE',  ( 209.7827226070571385, 36.64741339240061535, 13.08022668053247983 ) ) ;
#2833=CARTESIAN_POINT ( 'NONE',  ( 209.7513585654923816, 282.2246705312486483, -40.00000000000000711 ) ) ;
#2835=AXIS2_PLACEMENT_3D ( 'NONE', #93040, #42369, #58009 ) ;
#2837=FACE_OUTER_BOUND ( 'NONE', #66330, .T. ) ;
#2838=CARTESIAN_POINT ( 'NONE',  ( 196.1862243335229721, 25.40468116510840701, 14.05651170788187443 ) ) ;
#2855=ORIENTED_EDGE ( 'NONE', *, *, #52014, .F. ) ;
#2870=VERTEX_POINT ( 'NONE', #43934 ) ;
#2880=CARTESIAN_POINT ( 'NONE',  ( 208.4207707293412852, 35.83328680606452821, 15.07795544555653855 ) ) ;
#2889=EDGE_CURVE ( 'NONE', #67382, #91332, #11583, .T. ) ;
#2891=DIRECTION ( 'NONE',  ( 0.000000000000000000, 0.000000000000000000, 1.000000000000000000 ) ) ;
#2900=DIRECTION ( 'NONE',  ( 0.000000000000000000, 1.000000000000000000, 0.000000000000000000 ) ) ;
#2902=CARTESIAN_POINT ( 'NONE',  ( 197.4375396935993479, 24.88665474053333071, 11.71825508031674445 ) ) ;
#2905=DIRECTION ( 'NONE',  ( -0.000000000000000000, -1.000000000000000000, -9.656854691831248164E-17 ) ) ;
#2915=ORIENTED_EDGE ( 'NONE', *, *, #28070, .F. ) ;
#2916=DIRECTION ( 'NONE',  ( 0.000000000000000000, 0.000000000000000000, 1.000000000000000000 ) ) ;
#2919=CARTESIAN_POINT ( 'NONE',  ( 196.7904975038847795, 24.97768796420434256, 13.23503237509909880 ) ) ;
#2930=LINE ( 'NONE', #60708, #86796 ) ;
#2931=EDGE_CURVE ( 'NONE', #4825, #86359, #52442, .T. ) ;
#2934=DIRECTION ( 'NONE',  ( 0.7957555401921969640, 0.6056179655966498210, 0.000000000000000000 ) ) ;
#2949=ORIENTED_EDGE ( 'NONE', *, *, #86598, .T. ) ;
#2955=EDGE_CURVE ( 'NONE', #15079, #77887, #79661, .T. ) ;
#2965=VECTOR ( 'NONE', #11518, 1000.000000000000000 ) ;
#2969=DIRECTION ( 'NONE',  ( 0.000000000000000000, 0.000000000000000000, 1.000000000000000000 ) ) ;
#2982=CARTESIAN_POINT ( 'NONE',  ( 157.0521749816618069, 17.25638377771152676, 7.577257116167345430 ) ) ;
#2986=ORIENTED_EDGE ( 'NONE', *, *, #75967, .T. ) ;
#3008=DIRECTION ( 'NONE',  ( 0.000000000000000000, 0.000000000000000000, -1.000000000000000000 ) ) ;
#3009=DIRECTION ( 'NONE',  ( -1.000000000000000000, 0.000000000000000000, 0.000000000000000000 ) ) ;
#3012=DIRECTION ( 'NONE',  ( -1.000000000000000000, 0.000000000000000000, 0.000000000000000000 ) ) ;
#3016=CARTESIAN_POINT ( 'NONE',  ( 208.0212563688061209, 27.56882951438707607, 12.00000000000000000 ) ) ;
#3028=AXIS2_PLACEMENT_3D ( 'NONE', #31242, #65388, #22716 ) ;
#3030=ORIENTED_EDGE ( 'NONE', *, *, #89041, .T. ) ;
#3032=VECTOR ( 'NONE', #46391, 1000.000000000000000 ) ;
#3034=DIRECTION ( 'NONE',  ( 0.000000000000000000, 0.000000000000000000, -1.000000000000000000 ) ) ;
#3069=VERTEX_POINT ( 'NONE', #87028 ) ;
#3085=ORIENTED_EDGE ( 'NONE', *, *, #11508, .F. ) ;
#3090=EDGE_LOOP ( 'NONE', ( #20220, #50138, #1554, #40636 ) ) ;
#3098=LINE ( 'NONE', #67517, #66901 ) ;
#3104=CARTESIAN_POINT ( 'NONE',  ( 165.2424497756046549, 275.5000000000000568, 22.91843887563435800 ) ) ;
#3134=CARTESIAN_POINT ( 'NONE',  ( 189.4188515237862589, 293.9636489450775798, -9.103929867429222611 ) ) ;
#3137=DIRECTION ( 'NONE',  ( 0.000000000000000000, 1.000000000000000000, 0.000000000000000000 ) ) ;
#3145=DIRECTION ( 'NONE',  ( 0.000000000000000000, 1.000000000000000000, 0.000000000000000000 ) ) ;
#3168=AXIS2_PLACEMENT_3D ( 'NONE', #78776, #38339, #60149 ) ;
#3174=ORIENTED_EDGE ( 'NONE', *, *, #53671, .T. ) ;
#3175=CARTESIAN_POINT ( 'NONE',  ( 222.8344101925596306, 36.73669859915801794, 7.000000000000000000 ) ) ;
#3184=CARTESIAN_POINT ( 'NONE',  ( 175.2296996224750103, 214.5000000000000568, 0.000000000000000000 ) ) ;
#3198=ORIENTED_EDGE ( 'NONE', *, *, #88532, .F. ) ;
#3206=DIRECTION ( 'NONE',  ( 1.000000000000000000, 0.000000000000000000, 0.000000000000000000 ) ) ;
#3215=DIRECTION ( 'NONE',  ( 0.000000000000000000, 1.000000000000000000, 0.000000000000000000 ) ) ;
#3219=ORIENTED_EDGE ( 'NONE', *, *, #24991, .F. ) ;
#3234=CARTESIAN_POINT ( 'NONE',  ( 189.9243309297870610, 215.0000000000000568, 25.22542485937348644 ) ) ;
#3236=CARTESIAN_POINT ( 'NONE',  ( 155.0193286407019002, 19.71512530817393127, -13.29403319965122066 ) ) ;
#3247=DIRECTION ( 'NONE',  ( 1.000000000000000000, 0.000000000000000000, 0.000000000000000000 ) ) ;
#3249=EDGE_CURVE ( 'NONE', #71226, #4269, #76566, .T. ) ;
#3259=CARTESIAN_POINT ( 'NONE',  ( 139.1539576904058606, 250.0000000000000568, 10.50000000000000000 ) ) ;
#3269=ORIENTED_EDGE ( 'NONE', *, *, #11007, .T. ) ;
#3284=DIRECTION ( 'NONE',  ( -0.000000000000000000, -1.000000000000000000, -0.000000000000000000 ) ) ;
#3286=DIRECTION ( 'NONE',  ( 0.000000000000000000, 0.000000000000000000, 1.000000000000000000 ) ) ;
#3290=CARTESIAN_POINT ( 'NONE',  ( 165.0427047786672290, 275.5000000000000568, 23.37680765314704701 ) ) ;
#3297=AXIS2_PLACEMENT_3D ( 'NONE', #86504, #22132, #85589 ) ;
#3303=EDGE_CURVE ( 'NONE', #24040, #7041, #77458, .T. ) ;
#3310=ORIENTED_EDGE ( 'NONE', *, *, #24948, .F. ) ;
#3311=EDGE_LOOP ( 'NONE', ( #33346, #66788, #7493 ) ) ;
#3312=CARTESIAN_POINT ( 'NONE',  ( 194.3144103428324172, 215.0000000000000568, 16.91223866672520515 ) ) ;
#3328=ORIENTED_EDGE ( 'NONE', *, *, #46568, .F. ) ;
#3338=DIRECTION ( 'NONE',  ( 0.000000000000000000, 0.000000000000000000, 1.000000000000000000 ) ) ;
#3347=EDGE_CURVE ( 'NONE', #29030, #26503, #47183, .T. ) ;
#3351=FACE_OUTER_BOUND ( 'NONE', #71825, .T. ) ;
#3352=VECTOR ( 'NONE', #12074, 1000.000000000000000 ) ;
#3359=CIRCLE ( 'NONE', #409, 4.999999999999986677 ) ;
#3361=CARTESIAN_POINT ( 'NONE',  ( 200.6103193995254230, 275.0000000000000568, -2.464576988612312114 ) ) ;
#3364=LINE ( 'NONE', #90445, #82186 ) ;
#3368=DIRECTION ( 'NONE',  ( -0.000000000000000000, 1.000000000000000000, -0.000000000000000000 ) ) ;
#3377=ORIENTED_EDGE ( 'NONE', *, *, #93547, .F. ) ;
#3381=CARTESIAN_POINT ( 'NONE',  ( 156.4851178187871312, 3.000000000000000000, -7.000000000000000888 ) ) ;
#3392=CARTESIAN_POINT ( 'NONE',  ( 140.6539576904058606, 131.0000000000000568, -11.50000000000000000 ) ) ;
#3395=CARTESIAN_POINT ( 'NONE',  ( 202.9738562182569694, 293.9636489450776367, -54.00000000000000000 ) ) ;
#3411=ORIENTED_EDGE ( 'NONE', *, *, #84671, .F. ) ;
#3421=ORIENTED_EDGE ( 'NONE', *, *, #30621, .F. ) ;
#3422=AXIS2_PLACEMENT_3D ( 'NONE', #9639, #81603, #51330 ) ;
#3435=ORIENTED_EDGE ( 'NONE', *, *, #9771, .T. ) ;
#3437=VECTOR ( 'NONE', #19295, 1000.000000000000000 ) ;
#3443=VERTEX_POINT ( 'NONE', #18807 ) ;
#3444=DIRECTION ( 'NONE',  ( 0.000000000000000000, 0.000000000000000000, 1.000000000000000000 ) ) ;
#3449=ORIENTED_EDGE ( 'NONE', *, *, #50173, .T. ) ;
#3450=EDGE_CURVE ( 'NONE', #61449, #47327, #29358, .T. ) ;
#3467=VECTOR ( 'NONE', #39809, 1000.000000000000114 ) ;
#3468=CYLINDRICAL_SURFACE ( 'NONE', #29402, 25.00000000000000355 ) ;
#3469=( BOUNDED_SURFACE ( )  B_SPLINE_SURFACE ( 3, 2, ( 
 ( #14695, #57777, #86622 ),
 ( #63964, #43550, #87097 ),
 ( #72446, #22247, #51117 ),
 ( #7565, #36450, #65365 ) ),
 .UNSPECIFIED., .F., .F., .F. ) 
 B_SPLINE_SURFACE_WITH_KNOTS ( ( 4, 4 ),
 ( 3, 3 ),
 ( 4.278565243615663150, 4.712388980384689674 ),
 ( 0.000000000000000000, 1.000000000000000000 ),
 .UNSPECIFIED. ) 
 GEOMETRIC_REPRESENTATION_ITEM ( )  RATIONAL_B_SPLINE_SURFACE ( (
 ( 1.000000000000000000, 0.8168508380123955526, 1.000000000000000000),
 ( 1.000000000000000000, 0.7849082635113585615, 1.000000000000000000),
 ( 1.000000000000000000, 0.7478056585118741939, 1.000000000000000000),
 ( 1.000000000000000000, 0.7071067811865482389, 1.000000000000000000) ) ) 
 REPRESENTATION_ITEM ( '' )  SURFACE ( )  );
#3475=LINE ( 'NONE', #40825, #76092 ) ;
#3476=CARTESIAN_POINT ( 'NONE',  ( 194.7453183674696220, 20.99999999999999645, 15.62500000000048850 ) ) ;
#3481=FACE_OUTER_BOUND ( 'NONE', #83950, .T. ) ;
#3483=LINE ( 'NONE', #60333, #78480 ) ;
#3492=AXIS2_PLACEMENT_3D ( 'NONE', #26890, #3717, #69980 ) ;
#3499=CIRCLE ( 'NONE', #56446, 24.00000000000000355 ) ;
#3502=CARTESIAN_POINT ( 'NONE',  ( 159.4851178187871312, 69.18068689461284748, -7.000000000000000888 ) ) ;
#3504=ORIENTED_EDGE ( 'NONE', *, *, #8722, .F. ) ;
#3519=AXIS2_PLACEMENT_3D ( 'NONE', #17433, #18349, #3206 ) ;
#3522=CARTESIAN_POINT ( 'NONE',  ( 175.2296996224750103, 250.5000000000000568, 0.000000000000000000 ) ) ;
#3524=AXIS2_PLACEMENT_3D ( 'NONE', #39095, #830, #45739 ) ;
#3543=EDGE_CURVE ( 'NONE', #52528, #80622, #55017, .T. ) ;
#3561=ORIENTED_EDGE ( 'NONE', *, *, #29697, .T. ) ;
#3565=AXIS2_PLACEMENT_3D ( 'NONE', #71851, #6971, #36301 ) ;
#3576=CARTESIAN_POINT ( 'NONE',  ( 175.2296996224750103, 161.0000000000000853, 9.550761578869391144 ) ) ;
#3577=AXIS2_PLACEMENT_3D ( 'NONE', #90895, #39781, #41669 ) ;
#3579=AXIS2_PLACEMENT_3D ( 'NONE', #3184, #17412, #40540 ) ;
#3586=DIRECTION ( 'NONE',  ( 0.000000000000000000, 1.000000000000000000, 0.000000000000000000 ) ) ;
#3589=AXIS2_PLACEMENT_3D ( 'NONE', #35399, #72314, #92668 ) ;
#3596=EDGE_CURVE ( 'NONE', #45087, #74899, #45950, .T. ) ;
#3603=CARTESIAN_POINT ( 'NONE',  ( 140.6539576904058606, 250.5000000000000568, -12.50000000000000000 ) ) ;
#3608=ADVANCED_FACE ( 'NONE', ( #11689 ), #80700, .F. ) ;
#3622=FACE_OUTER_BOUND ( 'NONE', #33584, .T. ) ;
#3639=CARTESIAN_POINT ( 'NONE',  ( 165.0427047786672290, 249.5000000000000568, 23.37680765314704701 ) ) ;
#3647=TOROIDAL_SURFACE ( 'NONE', #65662, 24.50000000000000000, 0.5000000000000000000 ) ;
#3651=ORIENTED_EDGE ( 'NONE', *, *, #46092, .F. ) ;
#3652=DIRECTION ( 'NONE',  ( 0.5729786897769825194, 1.137382224641321619E-14, 0.8195702660915978877 ) ) ;
#3663=CARTESIAN_POINT ( 'NONE',  ( 169.9462594094670180, 250.5000000000000568, -23.92352941176469727 ) ) ;
#3664=CIRCLE ( 'NONE', #23325, 2.500000000000000444 ) ;
#3669=VERTEX_POINT ( 'NONE', #40082 ) ;
#3670=ADVANCED_FACE ( 'NONE', ( #26373 ), #69455, .F. ) ;
#3675=ADVANCED_FACE ( 'NONE', ( #53851 ), #61445, .T. ) ;
#3679=AXIS2_PLACEMENT_3D ( 'NONE', #24712, #10485, #68270 ) ;
#3681=ORIENTED_EDGE ( 'NONE', *, *, #203, .T. ) ;
#3686=CARTESIAN_POINT ( 'NONE',  ( 207.4345711710209343, 35.56792554197559042, 11.99999999999999822 ) ) ;
#3689=CARTESIAN_POINT ( 'NONE',  ( 209.2568086740244837, 34.98978593258890868, 12.09245862095592727 ) ) ;
#3690=CARTESIAN_POINT ( 'NONE',  ( 199.2296996224750103, 68.12454877777268791, 0.000000000000000000 ) ) ;
#3698=CARTESIAN_POINT ( 'NONE',  ( 196.8803347170859865, 73.40565171261609123, -12.49999999999998579 ) ) ;
#3702=CARTESIAN_POINT ( 'NONE',  ( 197.7570118961457695, 17.87787486654938363, 10.88803913700007975 ) ) ;
#3717=DIRECTION ( 'NONE',  ( -0.000000000000000000, -0.000000000000000000, -1.000000000000000000 ) ) ;
#3730=CARTESIAN_POINT ( 'NONE',  ( 201.2104617360081704, 60.19600395700749829, 7.000000000000000000 ) ) ;
#3732=FACE_OUTER_BOUND ( 'NONE', #62620, .T. ) ;
#3738=DIRECTION ( 'NONE',  ( -0.3024135303179394940, -0.9531768234072001134, 0.000000000000000000 ) ) ;
#3741=EDGE_CURVE ( 'NONE', #25512, #71850, #23283, .T. ) ;
#3752=VERTEX_POINT ( 'NONE', #70871 ) ;
#3753=FACE_OUTER_BOUND ( 'NONE', #58377, .T. ) ;
#3755=DIRECTION ( 'NONE',  ( -0.000000000000000000, -1.000000000000000000, -0.000000000000000000 ) ) ;
#3763=ORIENTED_EDGE ( 'NONE', *, *, #45526, .T. ) ;
#3773=DIRECTION ( 'NONE',  ( 0.000000000000000000, 0.000000000000000000, -1.000000000000000000 ) ) ;
#3774=CARTESIAN_POINT ( 'NONE',  ( 195.0811277904325038, 27.48493576247232539, 15.19607843137263892 ) ) ;
#3777=EDGE_CURVE ( 'NONE', #73850, #20929, #71819, .T. ) ;
#3784=VERTEX_POINT ( 'NONE', #64271 ) ;
#3788=CIRCLE ( 'NONE', #23462, 0.5000000000000128786 ) ;
#3794=ORIENTED_EDGE ( 'NONE', *, *, #21048, .T. ) ;
#3795=EDGE_LOOP ( 'NONE', ( #20981, #915 ) ) ;
#3814=ORIENTED_EDGE ( 'NONE', *, *, #88682, .F. ) ;
#3833=CARTESIAN_POINT ( 'NONE',  ( 200.1126601882107252, 249.5000000000000568, -2.416251949619908856 ) ) ;
#3835=LINE ( 'NONE', #27483, #38313 ) ;
#3842=CARTESIAN_POINT ( 'NONE',  ( 221.8344101925596306, 0.000000000000000000, 10.00000000000000000 ) ) ;
#3846=DIRECTION ( 'NONE',  ( -0.000000000000000000, -1.000000000000000000, -0.000000000000000000 ) ) ;
#3847=LINE ( 'NONE', #47845, #14071 ) ;
#3857=ORIENTED_EDGE ( 'NONE', *, *, #61840, .F. ) ;
#3861=CARTESIAN_POINT ( 'NONE',  ( 175.2296996224750103, 276.0000000000000568, 0.000000000000000000 ) ) ;
#3867=AXIS2_PLACEMENT_3D ( 'NONE', #30577, #37217, #59003 ) ;
#3874=CARTESIAN_POINT ( 'NONE',  ( 156.8934089303672295, 249.5000000000000568, 16.24901362097164537 ) ) ;
#3875=EDGE_CURVE ( 'NONE', #87519, #52231, #11143, .T. ) ;
#3876=FACE_OUTER_BOUND ( 'NONE', #88544, .T. ) ;
#3883=ADVANCED_FACE ( 'NONE', ( #48596 ), #13578, .F. ) ;
#3893=VERTEX_POINT ( 'NONE', #34414 ) ;
#3903=ORIENTED_EDGE ( 'NONE', *, *, #12254, .T. ) ;
#3915=VERTEX_POINT ( 'NONE', #33948 ) ;
#3922=ORIENTED_EDGE ( 'NONE', *, *, #92370, .F. ) ;
#3927=ORIENTED_EDGE ( 'NONE', *, *, #91947, .F. ) ;
#3940=CARTESIAN_POINT ( 'NONE',  ( 209.8616357346614905, 36.89613957940296274, 10.50000000000000000 ) ) ;
#3941=ADVANCED_FACE ( 'NONE', ( #41958 ), #17245, .T. ) ;
#3945=TOROIDAL_SURFACE ( 'NONE', #55384, 24.00000000000000355, 1.000000000000000000 ) ;
#3954=CARTESIAN_POINT ( 'NONE',  ( 195.4113456599614551, 19.73462695515988230, 13.33559673734781015 ) ) ;
#3959=CARTESIAN_POINT ( 'NONE',  ( 156.4851178187871312, 15.24064981607392255, -6.999999999998999023 ) ) ;
#3961=CARTESIAN_POINT ( 'NONE',  ( 155.8658096505380684, 20.95954935106544426, 14.18771993490441830 ) ) ;
#3964=CARTESIAN_POINT ( 'NONE',  ( 156.8097460172999149, 17.78059845260639804, -7.900495735315244517 ) ) ;
#3976=CARTESIAN_POINT ( 'NONE',  ( 157.4851178187871596, 1.000000000000001554, -8.171572875253810153 ) ) ;
#3978=ORIENTED_EDGE ( 'NONE', *, *, #89850, .T. ) ;
#3980=DIRECTION ( 'NONE',  ( 0.000000000000000000, 0.000000000000000000, -1.000000000000000000 ) ) ;
#3996=DIRECTION ( 'NONE',  ( 0.000000000000000000, 1.000000000000000000, 0.000000000000000000 ) ) ;
#4012=ORIENTED_EDGE ( 'NONE', *, *, #33617, .F. ) ;
#4023=EDGE_CURVE ( 'NONE', #83547, #2308, #67130, .T. ) ;
#4031=ORIENTED_EDGE ( 'NONE', *, *, #31052, .T. ) ;
#4033=( BOUNDED_SURFACE ( )  B_SPLINE_SURFACE ( 3, 2, ( 
 ( #63343, #28274, #49106 ),
 ( #50023, #91708, #78916 ),
 ( #14064, #55748, #71839 ),
 ( #57616, #86459, #48618 ),
 ( #28732, #77518, #12670 ),
 ( #41513, #82972, #1586 ),
 ( #89597, #24286, #53161 ),
 ( #2982, #37557, #31409 ),
 ( #68320, #46061, #60298 ),
 ( #16720, #66469, #67403 ),
 ( #38498, #2060, #52691 ),
 ( #30468, #89135, #45115 ),
 ( #82043, #54100, #30950 ),
 ( #10079, #88216, #38011 ) ),
 .UNSPECIFIED., .F., .F., .F. ) 
 B_SPLINE_SURFACE_WITH_KNOTS ( ( 4, 2, 2, 2, 2, 2, 4 ),
 ( 3, 3 ),
 ( 5.128070023563283009, 5.416848844467358148, 5.705627665371434176, 5.850017075823472190, 5.994406486275510204, 6.138795896727548218, 6.283185307179586232 ),
 ( 0.000000000000000000, 1.000000000000000000 ),
 .UNSPECIFIED. ) 
 GEOMETRIC_REPRESENTATION_ITEM ( )  RATIONAL_B_SPLINE_SURFACE ( (
 ( 1.000000000000000000, 0.9583671019092238064, 1.000000000000000000),
 ( 1.000000000000000000, 0.9398658125638107430, 1.000000000000000000),
 ( 1.000000000000000000, 0.9157002655843566874, 1.000000000000000000),
 ( 1.000000000000000000, 0.8622678315323227816, 1.000000000000000000),
 ( 1.000000000000000000, 0.8329613673159231846, 1.000000000000000000),
 ( 1.000000000000000000, 0.7919708659745474666, 1.000000000000000000),
 ( 1.000000000000000000, 0.7788285231915077489, 1.000000000000000000),
 ( 1.000000000000000000, 0.7549177526733943377, 1.000000000000000000),
 ( 1.000000000000000000, 0.7441566529437989574, 1.000000000000000000),
 ( 1.000000000000000000, 0.7262859251462961963, 1.000000000000000000),
 ( 1.000000000000000000, 0.7191857644035900554, 1.000000000000000000),
 ( 1.000000000000000000, 0.7095926089624357003, 1.000000000000000000),
 ( 1.000000000000000000, 0.7070960980132859897, 1.000000000000000000),
 ( 1.000000000000000000, 0.7071067811865473507, 1.000000000000000000) ) ) 
 REPRESENTATION_ITEM ( '' )  SURFACE ( )  );
#4038=VERTEX_POINT ( 'NONE', #78896 ) ;
#4040=ORIENTED_EDGE ( 'NONE', *, *, #67853, .F. ) ;
#4048=DIRECTION ( 'NONE',  ( 0.000000000000000000, 0.000000000000000000, 1.000000000000000000 ) ) ;
#4052=DIRECTION ( 'NONE',  ( -0.000000000000000000, -1.000000000000000000, -0.000000000000000000 ) ) ;
#4060=CARTESIAN_POINT ( 'NONE',  ( 153.2628468892384603, 20.37991841447901820, 11.93555113919330424 ) ) ;
#4065=CARTESIAN_POINT ( 'NONE',  ( 199.0350682890975236, 66.35678781651726865, 8.036454959886293992 ) ) ;
#4073=CARTESIAN_POINT ( 'NONE',  ( 189.4188515237862589, 293.9636489450775798, -40.00000000000000711 ) ) ;
#4088=CARTESIAN_POINT ( 'NONE',  ( 161.2494399300530290, 8.542400036368780647, 9.000000000000001776 ) ) ;
#4105=ORIENTED_EDGE ( 'NONE', *, *, #42456, .T. ) ;
#4108=FACE_OUTER_BOUND ( 'NONE', #54869, .T. ) ;
#4119=ORIENTED_EDGE ( 'NONE', *, *, #18958, .F. ) ;
#4120=DIRECTION ( 'NONE',  ( -0.000000000000000000, -0.000000000000000000, -1.000000000000000000 ) ) ;
#4124=EDGE_CURVE ( 'NONE', #29329, #86133, #42429, .T. ) ;
#4130=CARTESIAN_POINT ( 'NONE',  ( 196.8934835002044395, 70.76361186333477349, 10.57047112608304928 ) ) ;
#4131=DIRECTION ( 'NONE',  ( 0.000000000000000000, 0.000000000000000000, 1.000000000000000000 ) ) ;
#4135=ORIENTED_EDGE ( 'NONE', *, *, #16496, .F. ) ;
#4144=EDGE_LOOP ( 'NONE', ( #46379, #25207, #12148, #83850 ) ) ;
#4149=FACE_OUTER_BOUND ( 'NONE', #63894, .T. ) ;
#4152=CARTESIAN_POINT ( 'NONE',  ( 219.8344101925596021, 0.000000000000000000, 7.000000000000000000 ) ) ;
#4153=CARTESIAN_POINT ( 'NONE',  ( 198.9506515269346210, 68.58287003104832991, 4.213754548330891581 ) ) ;
#4164=CARTESIAN_POINT ( 'NONE',  ( 200.6868442215911728, 15.43634792868212635, 10.00000000000000178 ) ) ;
#4178=DIRECTION ( 'NONE',  ( -0.000000000000000000, -1.000000000000000000, -0.000000000000000000 ) ) ;
#4191=CARTESIAN_POINT ( 'NONE',  ( 157.4851178187871312, 15.00000000000000000, -7.000000000000000888 ) ) ;
#4199=CARTESIAN_POINT ( 'NONE',  ( 164.6329196456214277, 275.5000000000000568, 23.09031830825856346 ) ) ;
#4210=VERTEX_POINT ( 'NONE', #41488 ) ;
#4213=CARTESIAN_POINT ( 'NONE',  ( 207.5109667085373246, 0.03340139000135432246, -7.446935725088736469 ) ) ;
#4223=VERTEX_POINT ( 'NONE', #28254 ) ;
#4233=FACE_OUTER_BOUND ( 'NONE', #78998, .T. ) ;
#4248=EDGE_CURVE ( 'NONE', #38673, #23012, #57142, .T. ) ;
#4252=ORIENTED_EDGE ( 'NONE', *, *, #90122, .F. ) ;
#4253=VECTOR ( 'NONE', #13080, 1000.000000000000000 ) ;
#4254=DIRECTION ( 'NONE',  ( 0.000000000000000000, 0.000000000000000000, 1.000000000000000000 ) ) ;
#4259=CARTESIAN_POINT ( 'NONE',  ( 197.1195687025391976, 25.83768540896262778, 10.52967080450865822 ) ) ;
#4269=VERTEX_POINT ( 'NONE', #6939 ) ;
#4290=CARTESIAN_POINT ( 'NONE',  ( 199.9390245229544405, 68.58287003104832991, 4.389327654508852206 ) ) ;
#4292=CARTESIAN_POINT ( 'NONE',  ( 197.2116943569230330, 276.0000000000000568, -11.92446933126074882 ) ) ;
#4299=ADVANCED_FACE ( 'NONE', ( #57596 ), #86440, .F. ) ;
#4304=CARTESIAN_POINT ( 'NONE',  ( 204.6539576904058606, 287.9062406767683910, -5.225551010890931103 ) ) ;
#4318=ORIENTED_EDGE ( 'NONE', *, *, #34465, .T. ) ;
#4322=DIRECTION ( 'NONE',  ( -0.8195702660915913373, 0.000000000000000000, 0.5729786897769918452 ) ) ;
#4334=CARTESIAN_POINT ( 'NONE',  ( 175.2296996224750103, 214.5000000000000568, 0.000000000000000000 ) ) ;
#4355=CARTESIAN_POINT ( 'NONE',  ( 196.8803347170859865, 73.40565171261609123, -12.49999999999998579 ) ) ;
#4360=ORIENTED_EDGE ( 'NONE', *, *, #66323, .T. ) ;
#4367=CARTESIAN_POINT ( 'NONE',  ( 170.2305261370685798, 250.5000000000000568, -24.90909090909090295 ) ) ;
#4372=ORIENTED_EDGE ( 'NONE', *, *, #31927, .F. ) ;
#4379=ORIENTED_EDGE ( 'NONE', *, *, #41255, .F. ) ;
#4386=CIRCLE ( 'NONE', #64928, 5.603083949679982467 ) ;
#4392=DIRECTION ( 'NONE',  ( 0.000000000000000000, 1.000000000000000000, 0.000000000000000000 ) ) ;
#4397=CARTESIAN_POINT ( 'NONE',  ( 207.4724402404596333, 29.73442829110635444, 14.90057469441955362 ) ) ;
#4408=FACE_OUTER_BOUND ( 'NONE', #57371, .T. ) ;
#4411=EDGE_CURVE ( 'NONE', #22214, #89903, #24812, .T. ) ;
#4412=DIRECTION ( 'NONE',  ( 0.000000000000000000, 1.000000000000000000, 0.000000000000000000 ) ) ;
#4414=CARTESIAN_POINT ( 'NONE',  ( 156.4892692376084256, 15.19211566834932192, -9.995848581181771664 ) ) ;
#4416=CARTESIAN_POINT ( 'NONE',  ( 207.3051956367744424, 29.36351352329048581, 13.69055975427936289 ) ) ;
#4428=ORIENTED_EDGE ( 'NONE', *, *, #46324, .T. ) ;
#4448=VECTOR ( 'NONE', #56643, 1000.000000000000000 ) ;
#4450=CARTESIAN_POINT ( 'NONE',  ( 154.7659666677267865, 20.47222690886501439, -12.53936336329526391 ) ) ;
#4466=EDGE_LOOP ( 'NONE', ( #42447, #92408, #69125, #53684, #20238, #13242 ) ) ;
#4469=VERTEX_POINT ( 'NONE', #80752 ) ;
#4490=VERTEX_POINT ( 'NONE', #73200 ) ;
#4500=CARTESIAN_POINT ( 'NONE',  ( 152.0139507567511998, 20.82771571514204467, -9.304222368685264755 ) ) ;
#4504=CARTESIAN_POINT ( 'NONE',  ( 208.6208076322478746, 32.98517505407394168, 10.00000000000000000 ) ) ;
#4507=EDGE_CURVE ( 'NONE', #50747, #1828, #77739, .T. ) ;
#4514=CARTESIAN_POINT ( 'NONE',  ( 154.5829541210975151, 19.45714094959671314, -12.72029999255603450 ) ) ;
#4517=AXIS2_PLACEMENT_3D ( 'NONE', #5375, #12457, #71640 ) ;
#4520=CARTESIAN_POINT ( 'NONE',  ( 197.4836817735085219, 24.47698789593438917, 11.66666666666666785 ) ) ;
#4525=LINE ( 'NONE', #41426, #82904 ) ;
#4528=CARTESIAN_POINT ( 'NONE',  ( 197.2564953664965515, 42.34359863175593119, 11.92066879148802272 ) ) ;
#4543=CARTESIAN_POINT ( 'NONE',  ( 209.8616357346614905, 36.89613957940296274, 15.00000000000000000 ) ) ;
#4565=DIRECTION ( 'NONE',  ( 0.000000000000000000, -0.000000000000000000, 1.000000000000000000 ) ) ;
#4576=VERTEX_POINT ( 'NONE', #16358 ) ;
#4586=CARTESIAN_POINT ( 'NONE',  ( 184.8920641257441844, 2.973978534295031118, 8.999830714574057922 ) ) ;
#4587=CARTESIAN_POINT ( 'NONE',  ( 175.2296996224750103, 20.99999999999998934, 0.000000000000000000 ) ) ;
#4589=AXIS2_PLACEMENT_3D ( 'NONE', #91344, #62022, #39737 ) ;
#4601=ORIENTED_EDGE ( 'NONE', *, *, #8722, .T. ) ;
#4606=PLANE ( 'NONE',  #73366 ) ;
#4608=CARTESIAN_POINT ( 'NONE',  ( 175.2296996224750103, 276.0000000000000568, 0.000000000000000000 ) ) ;
#4609=CARTESIAN_POINT ( 'NONE',  ( 196.7383257810085979, 42.27872732282705925, 11.00000000000000000 ) ) ;
#4616=DIRECTION ( 'NONE',  ( -0.000000000000000000, -1.000000000000000000, -0.000000000000000000 ) ) ;
#4620=VERTEX_POINT ( 'NONE', #31045 ) ;
#4621=ORIENTED_EDGE ( 'NONE', *, *, #37438, .F. ) ;
#4622=DIRECTION ( 'NONE',  ( -0.000000000000000000, -1.000000000000000000, -0.000000000000000000 ) ) ;
#4626=EDGE_CURVE ( 'NONE', #41151, #90952, #49009, .T. ) ;
#4637=LINE ( 'NONE', #33511, #61063 ) ;
#4638=CARTESIAN_POINT ( 'NONE',  ( 195.4412442344684848, 39.86655514736339967, 13.94770545599002354 ) ) ;
#4649=EDGE_CURVE ( 'NONE', #11243, #34447, #37650, .T. ) ;
#4651=DIRECTION ( 'NONE',  ( 0.8620390091940283162, 0.000000000000000000, -0.5068419345592647396 ) ) ;
#4653=DIRECTION ( 'NONE',  ( 0.000000000000000000, 1.000000000000000000, 0.000000000000000000 ) ) ;
#4664=CARTESIAN_POINT ( 'NONE',  ( 195.0811277904324470, 39.36132622696000283, 15.19607843137254832 ) ) ;
#4674=CARTESIAN_POINT ( 'NONE',  ( 207.9682738430187214, 0.04008605884692675175, -7.489252814170929362 ) ) ;
#4684=ORIENTED_EDGE ( 'NONE', *, *, #1783, .F. ) ;
#4691=ORIENTED_EDGE ( 'NONE', *, *, #85740, .T. ) ;
#4706=ORIENTED_EDGE ( 'NONE', *, *, #999, .T. ) ;
#4713=EDGE_CURVE ( 'NONE', #49742, #87677, #73147, .T. ) ;
#4717=CARTESIAN_POINT ( 'NONE',  ( 165.7865175155837676, 3.000000000000000000, 9.000000000000001776 ) ) ;
#4718=AXIS2_PLACEMENT_3D ( 'NONE', #30902, #45071, #24716 ) ;
#4756=FACE_OUTER_BOUND ( 'NONE', #53050, .T. ) ;
#4758=CARTESIAN_POINT ( 'NONE',  ( 196.1963538710216994, 282.2246705312485915, -40.00000000000000711 ) ) ;
#4766=DIRECTION ( 'NONE',  ( 0.000000000000000000, 0.000000000000000000, 1.000000000000000000 ) ) ;
#4768=FACE_OUTER_BOUND ( 'NONE', #90044, .T. ) ;
#4771=DIRECTION ( 'NONE',  ( 1.000000000000000000, 0.000000000000000000, 0.000000000000000000 ) ) ;
#4781=AXIS2_PLACEMENT_3D ( 'NONE', #7869, #18135, #67044 ) ;
#4786=DIRECTION ( 'NONE',  ( -0.000000000000000000, -1.000000000000000000, -0.000000000000000000 ) ) ;
#4801=DIRECTION ( 'NONE',  ( 0.000000000000000000, 1.000000000000000000, 0.000000000000000000 ) ) ;
#4814=VERTEX_POINT ( 'NONE', #75409 ) ;
#4816=EDGE_LOOP ( 'NONE', ( #42290, #11420, #12767, #2855, #7733 ) ) ;
#4825=VERTEX_POINT ( 'NONE', #46506 ) ;
#4832=CARTESIAN_POINT ( 'NONE',  ( 165.4421947725420523, 276.0000000000000568, 22.46007009812166544 ) ) ;
#4837=ADVANCED_FACE ( 'NONE', ( #90061 ), #74766, .T. ) ;
#4851=ORIENTED_EDGE ( 'NONE', *, *, #36821, .T. ) ;
#4856=VECTOR ( 'NONE', #8693, 1000.000000000000000 ) ;
#4859=CARTESIAN_POINT ( 'NONE',  ( 202.9738562182569694, 293.9636489450776367, -44.00000000000000000 ) ) ;
#4868=CIRCLE ( 'NONE', #339, 4.999999999999993783 ) ;
#4876=CYLINDRICAL_SURFACE ( 'NONE', #71586, 4.999999999999984013 ) ;
#4877=DIRECTION ( 'NONE',  ( 0.000000000000000000, 1.000000000000000000, 0.000000000000000000 ) ) ;
#4881=LINE ( 'NONE', #62677, #78619 ) ;
#4883=VERTEX_POINT ( 'NONE', #4367 ) ;
#4884=DIRECTION ( 'NONE',  ( -1.000000000000000000, 0.000000000000000000, 0.000000000000000000 ) ) ;
#4889=CARTESIAN_POINT ( 'NONE',  ( 155.4202272374187714, 20.25578850494577665, -12.04866793599389396 ) ) ;
#4899=ORIENTED_EDGE ( 'NONE', *, *, #27543, .F. ) ;
#4902=DIRECTION ( 'NONE',  ( 0.3024135303176525569, 0.9531768234072912627, 0.000000000000000000 ) ) ;
#4921=CARTESIAN_POINT ( 'NONE',  ( 222.8344101925596306, 36.73669859915801794, -7.000000000000000888 ) ) ;
#4924=CIRCLE ( 'NONE', #92569, 4.999999999999986677 ) ;
#4931=DIRECTION ( 'NONE',  ( 0.000000000000000000, 1.000000000000000000, 0.000000000000000000 ) ) ;
#4934=EDGE_CURVE ( 'NONE', #64042, #74853, #40323, .T. ) ;
#4944=ORIENTED_EDGE ( 'NONE', *, *, #75080, .F. ) ;
#4958=ADVANCED_FACE ( 'NONE', ( #82957 ), #83417, .T. ) ;
#4961=ORIENTED_EDGE ( 'NONE', *, *, #30594, .F. ) ;
#4968=ORIENTED_EDGE ( 'NONE', *, *, #8073, .T. ) ;
#4976=CARTESIAN_POINT ( 'NONE',  ( 209.7513585654922679, 305.7026273589066818, 13.99999999999999112 ) ) ;
#4981=DIRECTION ( 'NONE',  ( 0.000000000000000000, 1.000000000000000000, 0.000000000000000000 ) ) ;
#4989=CARTESIAN_POINT ( 'NONE',  ( 153.4740190581475474, 20.31595717416274738, -12.31823986473498245 ) ) ;
#4993=AXIS2_PLACEMENT_3D ( 'NONE', #83914, #61688, #84371 ) ;
#4996=VECTOR ( 'NONE', #54963, 1000.000000000000000 ) ;
#4997=CARTESIAN_POINT ( 'NONE',  ( 197.1849154220910236, 70.00167207606656916, 10.14165260477480146 ) ) ;
#4999=AXIS2_PLACEMENT_3D ( 'NONE', #62706, #24823, #39459 ) ;
#5002=DIRECTION ( 'NONE',  ( -1.000000000000000000, 0.000000000000000000, 0.000000000000000000 ) ) ;
#5006=CYLINDRICAL_SURFACE ( 'NONE', #17159, 7.910944475430059519 ) ;
#5010=AXIS2_PLACEMENT_3D ( 'NONE', #36406, #29781, #44884 ) ;
#5022=CARTESIAN_POINT ( 'NONE',  ( 164.2231345125756263, 291.1800221208779931, 7.500000000000000000 ) ) ;
#5025=LINE ( 'NONE', #55224, #27169 ) ;
#5029=AXIS2_PLACEMENT_3D ( 'NONE', #20873, #6206, #93302 ) ;
#5043=CARTESIAN_POINT ( 'NONE',  ( 169.7306087885279169, 215.0000000000000568, -24.89999999999998792 ) ) ;
#5054=ORIENTED_EDGE ( 'NONE', *, *, #48, .T. ) ;
#5064=CIRCLE ( 'NONE', #57926, 24.00000000000001066 ) ;
#5066=DIRECTION ( 'NONE',  ( 0.000000000000000000, 0.000000000000000000, -1.000000000000000000 ) ) ;
#5072=EDGE_LOOP ( 'NONE', ( #48504, #81925, #52420, #87146, #87917, #35825, #76451, #55613, #54390, #82572, #65555 ) ) ;
#5079=AXIS2_PLACEMENT_3D ( 'NONE', #33405, #68468, #26311 ) ;
#5082=ORIENTED_EDGE ( 'NONE', *, *, #793, .T. ) ;
#5087=CARTESIAN_POINT ( 'NONE',  ( 216.5288609127277084, 293.9636489450776935, 13.99999999999999112 ) ) ;
#5091=CARTESIAN_POINT ( 'NONE',  ( 194.3144103428324172, 249.5000000000000568, 16.91223866672520515 ) ) ;
#5098=CARTESIAN_POINT ( 'NONE',  ( 207.4652116465272798, 29.76295193202772538, 14.90818566952114921 ) ) ;
#5100=CARTESIAN_POINT ( 'NONE',  ( 175.2296996224750103, 275.0000000000000568, 0.000000000000000000 ) ) ;
#5104=VERTEX_POINT ( 'NONE', #62140 ) ;
#5117=AXIS2_PLACEMENT_3D ( 'NONE', #36297, #318, #35383 ) ;
#5120=CARTESIAN_POINT ( 'NONE',  ( 175.2296996224750103, 249.5000000000000568, 0.000000000000000000 ) ) ;
#5121=PLANE ( 'NONE',  #20122 ) ;
#5133=CYLINDRICAL_SURFACE ( 'NONE', #58146, 0.5000000000000004441 ) ;
#5139=AXIS2_PLACEMENT_3D ( 'NONE', #60418, #89258, #40927 ) ;
#5144=CARTESIAN_POINT ( 'NONE',  ( 175.2296996224750103, 131.0000000000000568, 0.000000000000000000 ) ) ;
#5146=AXIS2_PLACEMENT_3D ( 'NONE', #20387, #56372, #64447 ) ;
#5153=CIRCLE ( 'NONE', #88260, 24.00000000000000355 ) ;
#5155=AXIS2_PLACEMENT_3D ( 'NONE', #54767, #68527, #54304 ) ;
#5159=CARTESIAN_POINT ( 'NONE',  ( 219.8344101925596021, 35.72494958537217968, 7.000000000000000000 ) ) ;
#5160=AXIS2_PLACEMENT_3D ( 'NONE', #32703, #88102, #23728 ) ;
#5171=AXIS2_PLACEMENT_3D ( 'NONE', #44618, #154, #77957 ) ;
#5174=CARTESIAN_POINT ( 'NONE',  ( 185.8264795993290477, 249.5000000000000568, 23.09031830825835385 ) ) ;
#5180=EDGE_CURVE ( 'NONE', #14315, #57029, #44470, .T. ) ;
#5181=ORIENTED_EDGE ( 'NONE', *, *, #50089, .T. ) ;
#5187=DIRECTION ( 'NONE',  ( 0.000000000000000000, 0.000000000000000000, 1.000000000000000000 ) ) ;
#5189=CARTESIAN_POINT ( 'NONE',  ( 208.6208076322478746, 32.98517505407394168, 12.09245862095555601 ) ) ;
#5192=ORIENTED_EDGE ( 'NONE', *, *, #21097, .F. ) ;
#5200=ORIENTED_EDGE ( 'NONE', *, *, #90748, .T. ) ;
#5221=AXIS2_PLACEMENT_3D ( 'NONE', #77564, #25040, #32138 ) ;
#5228=DIRECTION ( 'NONE',  ( 1.000000000000000000, 0.000000000000000000, 0.000000000000000000 ) ) ;
#5237=CARTESIAN_POINT ( 'NONE',  ( 196.1227023549103592, 275.0000000000000568, -11.81026827902096876 ) ) ;
#5238=AXIS2_PLACEMENT_3D ( 'NONE', #91230, #26396, #3009 ) ;
#5252=CARTESIAN_POINT ( 'NONE',  ( 140.6539576904058606, 249.5000000000000568, 12.00000000000000000 ) ) ;
#5254=PLANE ( 'NONE',  #58017 ) ;
#5264=DIRECTION ( 'NONE',  ( 0.000000000000000000, 0.000000000000000000, 1.000000000000000000 ) ) ;
#5266=CARTESIAN_POINT ( 'NONE',  ( 196.4642207764701141, 42.34395110402748941, 11.30645871156049687 ) ) ;
#5277=ORIENTED_EDGE ( 'NONE', *, *, #5180, .T. ) ;
#5280=CARTESIAN_POINT ( 'NONE',  ( 164.2231345125756263, 275.0000000000000568, 7.500000000000000000 ) ) ;
#5294=DIRECTION ( 'NONE',  ( 0.000000000000000000, 0.000000000000000000, 1.000000000000000000 ) ) ;
#5311=VERTEX_POINT ( 'NONE', #19052 ) ;
#5338=EDGE_CURVE ( 'NONE', #44839, #52563, #47502, .T. ) ;
#5341=VERTEX_POINT ( 'NONE', #4832 ) ;
#5342=CARTESIAN_POINT ( 'NONE',  ( 221.8344101925596306, 35.72494958537217968, -7.000000000000000888 ) ) ;
#5359=CARTESIAN_POINT ( 'NONE',  ( 175.2296996224750103, 142.2541816238762920, 0.000000000000000000 ) ) ;
#5375=CARTESIAN_POINT ( 'NONE',  ( 175.2296996224750103, 133.0000000000000000, 0.000000000000000000 ) ) ;
#5377=B_SPLINE_CURVE_WITH_KNOTS ( 'NONE', 3,
 ( #82823, #54881, #69107, #18916 ),
 .UNSPECIFIED., .F., .F.,
 ( 4, 4 ),
 ( 0.000000000000000000, 0.0006906318969024608651 ),
 .UNSPECIFIED. ) ;
#5380=CIRCLE ( 'NONE', #59782, 2.999999999999999112 ) ;
#5381=CARTESIAN_POINT ( 'NONE',  ( 206.2573329513795670, 29.95202539821489296, 13.98713712351915994 ) ) ;
#5397=CARTESIAN_POINT ( 'NONE',  ( 206.7023069086528722, 36.31764626557887965, 13.94198228246500904 ) ) ;
#5399=ORIENTED_EDGE ( 'NONE', *, *, #80495, .F. ) ;
#5401=CARTESIAN_POINT ( 'NONE',  ( 196.9298236971690415, 73.03079864117960085, 12.41428257208146668 ) ) ;
#5430=ORIENTED_EDGE ( 'NONE', *, *, #44800, .T. ) ;
#5448=ORIENTED_EDGE ( 'NONE', *, *, #53477, .T. ) ;
#5450=AXIS2_PLACEMENT_3D ( 'NONE', #84225, #35468, #92738 ) ;
#5468=CARTESIAN_POINT ( 'NONE',  ( 197.2116943569230045, 249.5000000000000568, -12.92446933126075592 ) ) ;
#5475=LINE ( 'NONE', #32930, #77517 ) ;
#5480=FACE_OUTER_BOUND ( 'NONE', #18708, .T. ) ;
#5486=CARTESIAN_POINT ( 'NONE',  ( 196.3627624770896034, 41.61148439004283262, 13.79125661931971969 ) ) ;
#5500=CARTESIAN_POINT ( 'NONE',  ( 210.8848006936870263, 293.9636489450776367, -40.00000000000000711 ) ) ;
#5502=ADVANCED_FACE ( 'NONE', ( #48375 ), #36974, .T. ) ;
#5504=EDGE_CURVE ( 'NONE', #50614, #65076, #6717, .T. ) ;
#5505=CARTESIAN_POINT ( 'NONE',  ( 152.4536156746142410, 275.0000000000000568, 14.50000000000000000 ) ) ;
#5508=AXIS2_PLACEMENT_3D ( 'NONE', #74702, #17413, #53373 ) ;
#5523=CARTESIAN_POINT ( 'NONE',  ( 155.7883889513938698, 17.75303870060442790, 10.69672886740308648 ) ) ;
#5542=EDGE_CURVE ( 'NONE', #10842, #84959, #82323, .T. ) ;
#5544=CARTESIAN_POINT ( 'NONE',  ( 199.0034008648431154, 66.39839742806377387, 8.059598887640509801 ) ) ;
#5549=ORIENTED_EDGE ( 'NONE', *, *, #15094, .T. ) ;
#5565=FACE_OUTER_BOUND ( 'NONE', #867, .T. ) ;
#5572=CARTESIAN_POINT ( 'NONE',  ( 156.4217629211117355, 119.0463968525363327, -10.00000000000000000 ) ) ;
#5573=FACE_OUTER_BOUND ( 'NONE', #17555, .T. ) ;
#5576=ORIENTED_EDGE ( 'NONE', *, *, #18516, .T. ) ;
#5577=CARTESIAN_POINT ( 'NONE',  ( 209.8744251295252354, 28.03846817292548366, 12.09245862095555601 ) ) ;
#5615=EDGE_CURVE ( 'NONE', #39404, #68312, #44530, .T. ) ;
#5619=CARTESIAN_POINT ( 'NONE',  ( 196.4677825244212102, 42.27466702580179714, 13.19434394796706655 ) ) ;
#5627=ORIENTED_EDGE ( 'NONE', *, *, #81728, .T. ) ;
#5628=DIRECTION ( 'NONE',  ( 0.000000000000000000, 1.000000000000000000, 0.000000000000000000 ) ) ;
#5630=LINE ( 'NONE', #56775, #9676 ) ;
#5644=CARTESIAN_POINT ( 'NONE',  ( 198.7350614680270269, 66.75098366856256860, -10.35296668938369180 ) ) ;
#5646=EDGE_LOOP ( 'NONE', ( #23340, #29843, #86455, #72923, #41393 ) ) ;
#5670=ORIENTED_EDGE ( 'NONE', *, *, #89476, .T. ) ;
#5681=EDGE_CURVE ( 'NONE', #15573, #76413, #49075, .T. ) ;
#5688=CARTESIAN_POINT ( 'NONE',  ( 195.4101840090182236, 19.73533033507746381, -13.33719194813488507 ) ) ;
#5702=CARTESIAN_POINT ( 'NONE',  ( 207.9682065434784022, 1.060642095945600216, -7.489249145872056701 ) ) ;
#5711=EDGE_CURVE ( 'NONE', #10872, #26346, #46011, .T. ) ;
#5712=FACE_OUTER_BOUND ( 'NONE', #15203, .T. ) ;
#5714=CARTESIAN_POINT ( 'NONE',  ( 200.4644824113734387, 214.9910457053126720, -2.942835885954282471 ) ) ;
#5723=CARTESIAN_POINT ( 'NONE',  ( 153.0292788520804663, 130.2722548028652625, 11.54371207238994934 ) ) ;
#5736=ORIENTED_EDGE ( 'NONE', *, *, #24919, .T. ) ;
#5739=DIRECTION ( 'NONE',  ( 0.000000000000000000, 1.000000000000000000, 0.000000000000000000 ) ) ;
#5751=PLANE ( 'NONE',  #9740 ) ;
#5782=CARTESIAN_POINT ( 'NONE',  ( 175.2296996224750103, 249.5000000000000568, 0.000000000000000000 ) ) ;
#5788=ORIENTED_EDGE ( 'NONE', *, *, #250, .F. ) ;
#5795=ORIENTED_EDGE ( 'NONE', *, *, #50231, .T. ) ;
#5800=ORIENTED_EDGE ( 'NONE', *, *, #20540, .T. ) ;
#5807=CARTESIAN_POINT ( 'NONE',  ( 152.4536156746142410, 250.0000000000000568, -14.50000000000000000 ) ) ;
#5821=EDGE_CURVE ( 'NONE', #78077, #60755, #80771, .T. ) ;
#5824=CARTESIAN_POINT ( 'NONE',  ( 213.7238915819278589, 32.98517505407394168, 10.50000000000000000 ) ) ;
#5826=CARTESIAN_POINT ( 'NONE',  ( 170.2305261370685798, 275.5000000000000568, -24.90909090909090295 ) ) ;
#5832=DIRECTION ( 'NONE',  ( 0.000000000000000000, 9.656854691831248164E-17, -1.000000000000000000 ) ) ;
#5836=CARTESIAN_POINT ( 'NONE',  ( 175.2296996224750103, 154.6894116713782807, 24.16304133878946558 ) ) ;
#5839=DIRECTION ( 'NONE',  ( 3.794040663998540091E-16, -1.000000000000000000, -4.956352788505168198E-16 ) ) ;
#5848=ADVANCED_FACE ( 'NONE', ( #13362 ), #64197, .T. ) ;
#5850=ORIENTED_EDGE ( 'NONE', *, *, #39899, .T. ) ;
#5855=VERTEX_POINT ( 'NONE', #93342 ) ;
#5869=EDGE_CURVE ( 'NONE', #11817, #84307, #30898, .T. ) ;
#5872=CARTESIAN_POINT ( 'NONE',  ( 154.1415209985679269, 20.37991841447901820, -11.45812909362559040 ) ) ;
#5888=ORIENTED_EDGE ( 'NONE', *, *, #89138, .T. ) ;
#5891=ORIENTED_EDGE ( 'NONE', *, *, #8888, .F. ) ;
#5897=AXIS2_PLACEMENT_3D ( 'NONE', #26191, #47014, #11523 ) ;
#5909=ORIENTED_EDGE ( 'NONE', *, *, #27071, .F. ) ;
#5917=EDGE_CURVE ( 'NONE', #86306, #83027, #68684, .T. ) ;
#5918=ORIENTED_EDGE ( 'NONE', *, *, #33819, .F. ) ;
#5937=DIRECTION ( 'NONE',  ( 0.000000000000000000, 0.000000000000000000, 1.000000000000000000 ) ) ;
#5942=CARTESIAN_POINT ( 'NONE',  ( 154.5625123364532101, 250.5000000000000568, -13.15740740740742254 ) ) ;
#5945=CARTESIAN_POINT ( 'NONE',  ( 208.3180124865313587, 30.15554586770298329, 14.31509665898690287 ) ) ;
#5964=CARTESIAN_POINT ( 'NONE',  ( 211.1232656141943949, 1.000000000000000888, 7.000000000000000000 ) ) ;
#5970=EDGE_CURVE ( 'NONE', #54214, #85888, #50249, .T. ) ;
#5978=ADVANCED_FACE ( 'NONE', ( #85767 ), #32451, .T. ) ;
#5992=ORIENTED_EDGE ( 'NONE', *, *, #89368, .F. ) ;
#6002=DIRECTION ( 'NONE',  ( 0.000000000000000000, 0.000000000000000000, 1.000000000000000000 ) ) ;
#6020=VERTEX_POINT ( 'NONE', #49786 ) ;
#6021=CARTESIAN_POINT ( 'NONE',  ( 200.8419735307467420, 26.78103457774642138, 10.49999999999999822 ) ) ;
#6022=DIRECTION ( 'NONE',  ( 1.000000000000000000, 0.000000000000000000, 0.000000000000000000 ) ) ;
#6023=CONICAL_SURFACE ( 'NONE', #34740, 24.00000000000001066, 0.7446590313522313265 ) ;
#6031=CARTESIAN_POINT ( 'NONE',  ( 154.1415209985679269, 20.37991841447902175, 11.45812909362559040 ) ) ;
#6035=EDGE_LOOP ( 'NONE', ( #27895, #41391, #35244, #60184, #63409, #9138, #53254, #34317, #76879, #47970, #45596, #27943, #60385, #84376, #89602, #36500, #49848, #71353, #50593, #74484, #24603, #56583 ) ) ;
#6051=CARTESIAN_POINT ( 'NONE',  ( 196.6877655503061533, 293.9636489450775230, -7.999911143031724237 ) ) ;
#6065=DIRECTION ( 'NONE',  ( 0.5877852522924681411, 0.000000000000000000, -0.8090169943749512260 ) ) ;
#6067=DIRECTION ( 'NONE',  ( -0.000000000000000000, -1.000000000000000000, -0.000000000000000000 ) ) ;
#6076=DIRECTION ( 'NONE',  ( -1.000000000000000000, 0.000000000000000000, 0.000000000000000000 ) ) ;
#6080=CARTESIAN_POINT ( 'NONE',  ( 195.2884072777227686, 40.74925082751602190, 14.92164996664659427 ) ) ;
#6086=TOROIDAL_SURFACE ( 'NONE', #68125, 1.000000000000000000, 0.5000000000000000000 ) ;
#6090=CARTESIAN_POINT ( 'NONE',  ( 150.7110049404237770, 21.00000000139189638, 5.101169899789431916 ) ) ;
#6093=CIRCLE ( 'NONE', #13669, 5.000000000000004441 ) ;
#6101=EDGE_CURVE ( 'NONE', #78927, #88979, #86695, .T. ) ;
#6103=ORIENTED_EDGE ( 'NONE', *, *, #8199, .F. ) ;
#6104=DIRECTION ( 'NONE',  ( 0.000000000000000000, -1.000000000000000000, 0.000000000000000000 ) ) ;
#6109=EDGE_LOOP ( 'NONE', ( #76397, #25919, #56935, #9258 ) ) ;
#6115=DIRECTION ( 'NONE',  ( 0.000000000000000000, 0.000000000000000000, 1.000000000000000000 ) ) ;
#6116=PLANE ( 'NONE',  #93147 ) ;
#6120=VERTEX_POINT ( 'NONE', #23707 ) ;
#6143=ADVANCED_FACE ( 'NONE', ( #29889 ), #55095, .T. ) ;
#6150=EDGE_LOOP ( 'NONE', ( #6583, #24016, #50242, #18562, #3814, #73236 ) ) ;
#6152=CARTESIAN_POINT ( 'NONE',  ( 156.6308165671946142, 214.7033826592484900, 16.75079304138620273 ) ) ;
#6158=EDGE_CURVE ( 'NONE', #17753, #50862, #48627, .T. ) ;
#6162=CARTESIAN_POINT ( 'NONE',  ( 199.4392256788250677, 65.82574266882504332, -7.741079165001071516 ) ) ;
#6165=AXIS2_PLACEMENT_3D ( 'NONE', #26689, #76877, #12478 ) ;
#6169=CARTESIAN_POINT ( 'NONE',  ( 198.5086862847412306, 68.69963673584575758, -12.80442219784223923 ) ) ;
#6170=AXIS2_PLACEMENT_3D ( 'NONE', #6343, #77369, #64142 ) ;
#6171=CARTESIAN_POINT ( 'NONE',  ( 153.3662726500193116, 20.33089334036130680, -12.12590166673910907 ) ) ;
#6179=CARTESIAN_POINT ( 'NONE',  ( 192.9623460957494956, 250.0000000000000568, 16.90571646082667812 ) ) ;
#6181=FACE_OUTER_BOUND ( 'NONE', #9022, .T. ) ;
#6192=CARTESIAN_POINT ( 'NONE',  ( 140.6539576904058606, 275.0000000000000568, 12.50000000000000000 ) ) ;
#6203=ORIENTED_EDGE ( 'NONE', *, *, #55527, .T. ) ;
#6204=CARTESIAN_POINT ( 'NONE',  ( 188.3531807883583440, 45.29379214021909661, 10.50000000000000000 ) ) ;
#6206=DIRECTION ( 'NONE',  ( -0.000000000000000000, 1.000000000000000000, -0.000000000000000000 ) ) ;
#6219=FACE_OUTER_BOUND ( 'NONE', #40685, .T. ) ;
#6231=ORIENTED_EDGE ( 'NONE', *, *, #93048, .F. ) ;
#6233=EDGE_LOOP ( 'NONE', ( #29746, #4621, #92950, #76082, #91360 ) ) ;
#6237=EDGE_CURVE ( 'NONE', #42461, #78803, #9730, .T. ) ;
#6247=DIRECTION ( 'NONE',  ( -0.000000000000000000, -0.000000000000000000, -1.000000000000000000 ) ) ;
#6263=EDGE_CURVE ( 'NONE', #88883, #86547, #65618, .T. ) ;
#6281=ORIENTED_EDGE ( 'NONE', *, *, #9083, .F. ) ;
#6288=CARTESIAN_POINT ( 'NONE',  ( 185.0172044724083946, 250.0000000000000568, 22.46007009812148425 ) ) ;
#6289=CARTESIAN_POINT ( 'NONE',  ( 154.5625123364532101, 250.0000000000000568, 13.15740740740740655 ) ) ;
#6296=CARTESIAN_POINT ( 'NONE',  ( 193.4805245855986584, 250.1588552167598039, 16.89623126087845861 ) ) ;
#6298=LINE ( 'NONE', #48902, #80414 ) ;
#6301=DIRECTION ( 'NONE',  ( 0.000000000000000000, 0.000000000000000000, 1.000000000000000000 ) ) ;
#6329=ORIENTED_EDGE ( 'NONE', *, *, #19750, .F. ) ;
#6335=CARTESIAN_POINT ( 'NONE',  ( 175.2296996224750103, 149.6461846693799487, 24.00000000000001066 ) ) ;
#6343=CARTESIAN_POINT ( 'NONE',  ( 140.6539576904058606, 250.5000000000000568, 10.50000000000000000 ) ) ;
#6353=VERTEX_POINT ( 'NONE', #87161 ) ;
#6358=ADVANCED_FACE ( 'NONE', ( #87615 ), #52116, .F. ) ;
#6362=TOROIDAL_SURFACE ( 'NONE', #4781, 24.50000000000001066, 0.5000000000000000000 ) ;
#6365=CIRCLE ( 'NONE', #32022, 3.589950628481164419 ) ;
#6373=VERTEX_POINT ( 'NONE', #81450 ) ;
#6375=AXIS2_PLACEMENT_3D ( 'NONE', #50306, #36106, #87209 ) ;
#6382=EDGE_CURVE ( 'NONE', #74598, #307, #2242, .T. ) ;
#6383=ORIENTED_EDGE ( 'NONE', *, *, #23960, .T. ) ;
#6395=DIRECTION ( 'NONE',  ( -0.000000000000000000, -1.000000000000000000, -0.000000000000000000 ) ) ;
#6405=CARTESIAN_POINT ( 'NONE',  ( 208.4306832106271088, -74.55766379199613425, 7.500000000000013323 ) ) ;
#6420=VECTOR ( 'NONE', #13501, 1000.000000000000000 ) ;
#6422=AXIS2_PLACEMENT_3D ( 'NONE', #32622, #90344, #54377 ) ;
#6426=CARTESIAN_POINT ( 'NONE',  ( 152.4536156746142410, 249.5000000000000568, 14.50000000000000000 ) ) ;
#6428=CIRCLE ( 'NONE', #20006, 0.5000000000000004441 ) ;
#6430=CARTESIAN_POINT ( 'NONE',  ( 219.8344101925596021, 35.72494958537217968, -7.000000000000000888 ) ) ;
#6444=EDGE_CURVE ( 'NONE', #79467, #85305, #12868, .T. ) ;
#6459=ORIENTED_EDGE ( 'NONE', *, *, #12627, .T. ) ;
#6460=VERTEX_POINT ( 'NONE', #28955 ) ;
#6484=EDGE_LOOP ( 'NONE', ( #33767, #26856, #40529, #61563, #76682, #33936, #28025, #52477 ) ) ;
#6491=CARTESIAN_POINT ( 'NONE',  ( 208.6208076322478746, 32.98517505407394168, 10.00000000000000000 ) ) ;
#6498=AXIS2_PLACEMENT_3D ( 'NONE', #25153, #17593, #46443 ) ;
#6499=CARTESIAN_POINT ( 'NONE',  ( 209.6851631783452490, 27.99050452776153008, 13.95111757441321920 ) ) ;
#6504=CARTESIAN_POINT ( 'NONE',  ( 209.7513585654923816, 282.2246705312486483, -40.00000000000000711 ) ) ;
#6506=CARTESIAN_POINT ( 'NONE',  ( 183.0442525570908288, 275.0000000000000568, 20.22542485937379908 ) ) ;
#6509=EDGE_CURVE ( 'NONE', #13368, #48695, #44542, .T. ) ;
#6521=CARTESIAN_POINT ( 'NONE',  ( 196.9274440531671360, 292.2264140707667366, -7.812896314794627983 ) ) ;
#6524=AXIS2_PLACEMENT_3D ( 'NONE', #29864, #87591, #80499 ) ;
#6551=CARTESIAN_POINT ( 'NONE',  ( 196.0677363144156402, 41.33745432255098251, 14.18591286744891633 ) ) ;
#6556=VECTOR ( 'NONE', #54357, 1000.000000000000000 ) ;
#6562=ORIENTED_EDGE ( 'NONE', *, *, #85946, .T. ) ;
#6563=CARTESIAN_POINT ( 'NONE',  ( 140.6539576904058606, 275.0000000000000568, -10.49999999999999822 ) ) ;
#6566=DIRECTION ( 'NONE',  ( -0.000000000000000000, 1.000000000000000000, -0.000000000000000000 ) ) ;
#6569=EDGE_CURVE ( 'NONE', #13227, #55526, #85443, .T. ) ;
#6577=ORIENTED_EDGE ( 'NONE', *, *, #73794, .F. ) ;
#6583=ORIENTED_EDGE ( 'NONE', *, *, #91723, .T. ) ;
#6589=CARTESIAN_POINT ( 'NONE',  ( 198.7877904355241014, 66.56388957926334626, -9.416941149845250436 ) ) ;
#6591=FACE_OUTER_BOUND ( 'NONE', #50586, .T. ) ;
#6601=ORIENTED_EDGE ( 'NONE', *, *, #65063, .F. ) ;
#6624=ORIENTED_EDGE ( 'NONE', *, *, #34302, .F. ) ;
#6636=TOROIDAL_SURFACE ( 'NONE', #30813, 24.00000000000000355, 1.000000000000000000 ) ;
#6642=CARTESIAN_POINT ( 'NONE',  ( 197.9445473535714939, 71.72765703697457695, -10.67027600767165652 ) ) ;
#6643=CARTESIAN_POINT ( 'NONE',  ( 154.5625123364532101, 276.0000000000000568, -13.15740740740742254 ) ) ;
#6660=AXIS2_PLACEMENT_3D ( 'NONE', #61021, #83697, #41053 ) ;
#6670=CARTESIAN_POINT ( 'NONE',  ( 198.7989590516236547, 65.26577858576978031, -10.60668493626651454 ) ) ;
#6681=ORIENTED_EDGE ( 'NONE', *, *, #40020, .F. ) ;
#6687=EDGE_CURVE ( 'NONE', #77289, #81908, #71811, .T. ) ;
#6702=CIRCLE ( 'NONE', #39905, 0.5000000000000004441 ) ;
#6717=CIRCLE ( 'NONE', #52044, 9.103929867429224387 ) ;
#6722=ORIENTED_EDGE ( 'NONE', *, *, #93228, .F. ) ;
#6724=AXIS2_PLACEMENT_3D ( 'NONE', #80545, #43186, #79641 ) ;
#6733=ORIENTED_EDGE ( 'NONE', *, *, #30878, .F. ) ;
#6737=AXIS2_PLACEMENT_3D ( 'NONE', #49061, #37508, #44146 ) ;
#6741=ORIENTED_EDGE ( 'NONE', *, *, #39378, .T. ) ;
#6742=CARTESIAN_POINT ( 'NONE',  ( 195.0233977251112947, 26.09208739110615838, 13.58423960365109195 ) ) ;
#6767=CARTESIAN_POINT ( 'NONE',  ( 175.2296996224750103, 134.0000000000000284, 0.000000000000000000 ) ) ;
#6773=DIRECTION ( 'NONE',  ( 0.000000000000000000, 0.000000000000000000, 1.000000000000000000 ) ) ;
#6775=CARTESIAN_POINT ( 'NONE',  ( 151.4851178187871312, 20.00000000000000000, 3.492110388858666870 ) ) ;
#6778=CARTESIAN_POINT ( 'NONE',  ( 140.6539576904058606, 276.0000000000000568, -10.49999999999999822 ) ) ;
#6779=DIRECTION ( 'NONE',  ( 0.000000000000000000, 0.000000000000000000, 1.000000000000000000 ) ) ;
#6786=VECTOR ( 'NONE', #15157, 1000.000000000000000 ) ;
#6789=EDGE_CURVE ( 'NONE', #59928, #48925, #82513, .T. ) ;
#6813=CARTESIAN_POINT ( 'NONE',  ( 160.6539576904058606, 293.9636489450775230, -7.999911143031724237 ) ) ;
#6830=ORIENTED_EDGE ( 'NONE', *, *, #48291, .F. ) ;
#6854=VERTEX_POINT ( 'NONE', #46855 ) ;
#6866=DIRECTION ( 'NONE',  ( -1.000000000000000000, 0.000000000000000000, 0.000000000000000000 ) ) ;
#6879=CARTESIAN_POINT ( 'NONE',  ( 185.2519943799831879, 3.000000000000000000, 9.000000000000001776 ) ) ;
#6883=DIRECTION ( 'NONE',  ( 1.000000000000000000, 0.000000000000000000, 0.000000000000000000 ) ) ;
#6889=CARTESIAN_POINT ( 'NONE',  ( 208.4306832106271088, -74.55766379199613425, -7.500000000000013323 ) ) ;
#6894=EDGE_CURVE ( 'NONE', #36590, #74948, #25979, .T. ) ;
#6914=EDGE_CURVE ( 'NONE', #36583, #39232, #31706, .T. ) ;
#6927=AXIS2_PLACEMENT_3D ( 'NONE', #73676, #65670, #8787 ) ;
#6939=CARTESIAN_POINT ( 'NONE',  ( 140.6539576904058606, 131.0000000000000568, 11.50000000000000000 ) ) ;
#6944=ORIENTED_EDGE ( 'NONE', *, *, #25879, .F. ) ;
#6952=ORIENTED_EDGE ( 'NONE', *, *, #82203, .F. ) ;
#6957=DIRECTION ( 'NONE',  ( 0.000000000000000000, 0.000000000000000000, 1.000000000000000000 ) ) ;
#6958=CARTESIAN_POINT ( 'NONE',  ( 175.2296996224750103, 250.5000000000000568, 0.000000000000000000 ) ) ;
#6966=DIRECTION ( 'NONE',  ( -1.000000000000000000, 0.000000000000000000, 0.000000000000000000 ) ) ;
#6971=DIRECTION ( 'NONE',  ( -0.000000000000000000, -0.000000000000000000, 1.000000000000000000 ) ) ;
#6973=ADVANCED_FACE ( 'NONE', ( #39742 ), #38826, .T. ) ;
#6986=CARTESIAN_POINT ( 'NONE',  ( 195.4638858641033892, 26.97464251841893201, 13.94285838819634549 ) ) ;
#7004=CARTESIAN_POINT ( 'NONE',  ( 193.9402003287077605, 214.5000000000000568, 16.58062614384823874 ) ) ;
#7026=EDGE_CURVE ( 'NONE', #41724, #52563, #74841, .T. ) ;
#7029=ORIENTED_EDGE ( 'NONE', *, *, #73031, .F. ) ;
#7030=DIRECTION ( 'NONE',  ( -0.000000000000000000, -1.000000000000000000, -0.000000000000000000 ) ) ;
#7041=VERTEX_POINT ( 'NONE', #40215 ) ;
#7042=DIRECTION ( 'NONE',  ( 0.000000000000000000, 0.000000000000000000, -1.000000000000000000 ) ) ;
#7049=VERTEX_POINT ( 'NONE', #75296 ) ;
#7055=CARTESIAN_POINT ( 'NONE',  ( 160.5350683151633291, 215.0000000000000568, 20.22542485937379908 ) ) ;
#7056=DIRECTION ( 'NONE',  ( 0.9167375550253613614, -2.772018683170089088E-15, -0.3994899938748440738 ) ) ;
#7065=ORIENTED_EDGE ( 'NONE', *, *, #76588, .F. ) ;
#7073=DIRECTION ( 'NONE',  ( -1.000000000000000000, 0.000000000000000000, 0.000000000000000000 ) ) ;
#7087=VERTEX_POINT ( 'NONE', #9954 ) ;
#7089=PLANE ( 'NONE',  #45867 ) ;
#7091=( BOUNDED_SURFACE ( )  B_SPLINE_SURFACE ( 3, 2, ( 
 ( #90402, #31287, #54439 ),
 ( #60635, #47316, #54908 ),
 ( #11363, #89472, #69131 ),
 ( #24633, #82396, #10415 ),
 ( #83787, #4259, #47796 ),
 ( #39279, #76698, #11824 ) ),
 .UNSPECIFIED., .F., .F., .F. ) 
 B_SPLINE_SURFACE_WITH_KNOTS ( ( 4, 2, 4 ),
 ( 3, 3 ),
 ( 4.712388980384689674, 5.132923315668655562, 5.553457650952620561 ),
 ( 0.000000000000000000, 1.000000000000000000 ),
 .UNSPECIFIED. ) 
 GEOMETRIC_REPRESENTATION_ITEM ( )  RATIONAL_B_SPLINE_SURFACE ( (
 ( 1.000000000000000000, 0.7071067811865479058, 1.000000000000000000),
 ( 1.000000000000000000, 0.7192895461630171017, 1.000000000000000000),
 ( 1.000000000000000000, 0.7311219824197653372, 1.000000000000000000),
 ( 1.000000000000000000, 0.7523130761988451320, 1.000000000000000000),
 ( 1.000000000000000000, 0.7616706333094609427, 1.000000000000000000),
 ( 1.000000000000000000, 0.7691239371209227516, 1.000000000000000000) ) ) 
 REPRESENTATION_ITEM ( '' )  SURFACE ( )  );
#7104=CARTESIAN_POINT ( 'NONE',  ( 198.7962788613944554, 70.38469146215045669, -8.627472241147954080 ) ) ;
#7105=CARTESIAN_POINT ( 'NONE',  ( 164.5772123382336360, 215.0000000000000568, 23.16839473634451352 ) ) ;
#7116=DIRECTION ( 'NONE',  ( -1.000000000000000000, 2.528396334038674078E-14, 0.000000000000000000 ) ) ;
#7118=PLANE ( 'NONE',  #76246 ) ;
#7129=LINE ( 'NONE', #6192, #45722 ) ;
#7140=DIRECTION ( 'NONE',  ( -0.9531768234071980039, 0.3024135303179465994, 0.000000000000000000 ) ) ;
#7153=CARTESIAN_POINT ( 'NONE',  ( 195.4781563537916043, 39.36132622696000283, 15.00000000000000000 ) ) ;
#7155=FACE_OUTER_BOUND ( 'NONE', #28486, .T. ) ;
#7167=ORIENTED_EDGE ( 'NONE', *, *, #41597, .T. ) ;
#7175=ORIENTED_EDGE ( 'NONE', *, *, #89946, .F. ) ;
#7181=CARTESIAN_POINT ( 'NONE',  ( 196.3496553477289979, 275.5000000000000568, -12.41762739670151028 ) ) ;
#7193=ORIENTED_EDGE ( 'NONE', *, *, #48633, .T. ) ;
#7194=CARTESIAN_POINT ( 'NONE',  ( 196.2721731643909493, 25.96757666558882249, 13.11199317982073964 ) ) ;
#7209=ADVANCED_FACE ( 'NONE', ( #67733 ), #7091, .T. ) ;
#7211=ADVANCED_FACE ( 'NONE', ( #21807 ), #80467, .F. ) ;
#7220=DIRECTION ( 'NONE',  ( -1.000000000000000000, 0.000000000000000000, 0.000000000000000000 ) ) ;
#7226=CARTESIAN_POINT ( 'NONE',  ( 210.0121166852535453, 37.89751991204045822, 12.09245862092500445 ) ) ;
#7231=DIRECTION ( 'NONE',  ( 0.000000000000000000, 0.000000000000000000, 1.000000000000000000 ) ) ;
#7232=DIRECTION ( 'NONE',  ( 0.5729786897769378884, 0.000000000000000000, -0.8195702660916291959 ) ) ;
#7244=CARTESIAN_POINT ( 'NONE',  ( 197.1656530321902494, 41.90019538913895758, 12.64285714285713169 ) ) ;
#7246=EDGE_LOOP ( 'NONE', ( #80302, #26116, #84583, #21763 ) ) ;
#7260=DIRECTION ( 'NONE',  ( 0.000000000000000000, 1.000000000000000000, 0.000000000000000000 ) ) ;
#7314=DIRECTION ( 'NONE',  ( -1.000000000000000000, -0.000000000000000000, 0.000000000000000000 ) ) ;
#7320=CARTESIAN_POINT ( 'NONE',  ( 185.2169494693457921, 214.5000000000000568, 22.91843887563416615 ) ) ;
#7329=DIRECTION ( 'NONE',  ( -0.5000000000000046629, 0.8660254037844359321, 0.000000000000000000 ) ) ;
#7332=LINE ( 'NONE', #78839, #67864 ) ;
#7363=AXIS2_PLACEMENT_3D ( 'NONE', #2833, #53490, #82366 ) ;
#7403=ORIENTED_EDGE ( 'NONE', *, *, #70232, .T. ) ;
#7405=CARTESIAN_POINT ( 'NONE',  ( 196.1604930303647052, 24.75642484911453067, 13.67253731732742494 ) ) ;
#7413=CARTESIAN_POINT ( 'NONE',  ( 209.7199135963037406, 27.99931114053373804, 12.09245862092541657 ) ) ;
#7415=LINE ( 'NONE', #23845, #64300 ) ;
#7419=FACE_OUTER_BOUND ( 'NONE', #2512, .T. ) ;
#7435=CARTESIAN_POINT ( 'NONE',  ( 196.5940483389518647, 25.86285152137379839, 12.79436563626940249 ) ) ;
#7449=LINE ( 'NONE', #78043, #39566 ) ;
#7457=CARTESIAN_POINT ( 'NONE',  ( 197.4027394742815886, 40.84896208771627357, 12.00000000000000533 ) ) ;
#7474=CARTESIAN_POINT ( 'NONE',  ( 152.6878565075764413, 20.88255170682893080, 8.268021619243398845 ) ) ;
#7476=LINE ( 'NONE', #27885, #65620 ) ;
#7486=ORIENTED_EDGE ( 'NONE', *, *, #38083, .T. ) ;
#7487=CARTESIAN_POINT ( 'NONE',  ( 195.9399694403358012, 40.74223533523908714, 13.37580287366501075 ) ) ;
#7493=ORIENTED_EDGE ( 'NONE', *, *, #10209, .F. ) ;
#7499=FACE_OUTER_BOUND ( 'NONE', #65338, .T. ) ;
#7500=DIRECTION ( 'NONE',  ( 0.000000000000000000, 0.000000000000000000, 1.000000000000000000 ) ) ;
#7504=ORIENTED_EDGE ( 'NONE', *, *, #55943, .T. ) ;
#7511=EDGE_LOOP ( 'NONE', ( #17720, #57229, #12802, #9857, #45994, #67486, #38928 ) ) ;
#7520=EDGE_CURVE ( 'NONE', #26188, #92859, #17383, .T. ) ;
#7521=CYLINDRICAL_SURFACE ( 'NONE', #5010, 24.00000000000001066 ) ;
#7535=ORIENTED_EDGE ( 'NONE', *, *, #79046, .F. ) ;
#7562=CARTESIAN_POINT ( 'NONE',  ( 185.2169494693457921, 275.5000000000000568, 22.91843887563416615 ) ) ;
#7565=CARTESIAN_POINT ( 'NONE',  ( 201.2104617360081704, 60.19600395700751250, 9.000000000000000000 ) ) ;
#7572=DIRECTION ( 'NONE',  ( -0.000000000000000000, -0.000000000000000000, 1.000000000000000000 ) ) ;
#7573=CARTESIAN_POINT ( 'NONE',  ( 152.4536156746142410, 275.0000000000000568, -12.49999999999999289 ) ) ;
#7576=CARTESIAN_POINT ( 'NONE',  ( 197.3617861379907481, 72.09200933227452879, -11.67137979308930973 ) ) ;
#7586=FACE_OUTER_BOUND ( 'NONE', #37527, .T. ) ;
#7599=CARTESIAN_POINT ( 'NONE',  ( 209.2599468862078140, 293.9636489450776367, -44.00000000000000000 ) ) ;
#7600=EDGE_CURVE ( 'NONE', #26503, #27314, #50680, .T. ) ;
#7601=CARTESIAN_POINT ( 'NONE',  ( 159.4851178187871312, 17.43233815881133708, 9.000000000000000000 ) ) ;
#7613=ORIENTED_EDGE ( 'NONE', *, *, #55070, .T. ) ;
#7616=( BOUNDED_CURVE ( )  B_SPLINE_CURVE ( 3, ( #9043, #88590, #34121, #69628 ),
 .UNSPECIFIED., .F., .F. ) 
 B_SPLINE_CURVE_WITH_KNOTS ( ( 4, 4 ),
 ( 1.570796326794896780, 3.141592653589793116 ),
 .UNSPECIFIED. ) 
 CURVE ( )  GEOMETRIC_REPRESENTATION_ITEM ( )  RATIONAL_B_SPLINE_CURVE ( ( 1.000000000000000000, 0.8047378541243650485, 0.8047378541243650485, 1.000000000000000000 ) ) 
 REPRESENTATION_ITEM ( '' )  );
#7621=AXIS2_PLACEMENT_3D ( 'NONE', #46135, #2135, #82591 ) ;
#7623=ORIENTED_EDGE ( 'NONE', *, *, #24310, .F. ) ;
#7642=ORIENTED_EDGE ( 'NONE', *, *, #18737, .T. ) ;
#7643=CARTESIAN_POINT ( 'NONE',  ( 195.8183634747502708, 24.45209547744994438, 12.33938814790248628 ) ) ;
#7661=VERTEX_POINT ( 'NONE', #44940 ) ;
#7668=ADVANCED_FACE ( 'NONE', ( #79099 ), #15616, .T. ) ;
#7671=DIRECTION ( 'NONE',  ( 0.000000000000000000, 0.000000000000000000, 1.000000000000000000 ) ) ;
#7679=FACE_OUTER_BOUND ( 'NONE', #18341, .T. ) ;
#7682=CARTESIAN_POINT ( 'NONE',  ( 199.9311642430739653, 275.7557892102190067, 9.103929867429336298 ) ) ;
#7683=DIRECTION ( 'NONE',  ( -0.000000000000000000, -1.000000000000000000, -0.000000000000000000 ) ) ;
#7696=CARTESIAN_POINT ( 'NONE',  ( 186.6539576904058890, 276.0000000000000568, 11.60392986742922616 ) ) ;
#7698=ORIENTED_EDGE ( 'NONE', *, *, #75701, .F. ) ;
#7710=CARTESIAN_POINT ( 'NONE',  ( 154.0561329571324904, 19.33057573605696788, 12.42898486165470118 ) ) ;
#7713=DIRECTION ( 'NONE',  ( -0.000000000000000000, -1.000000000000000000, -0.000000000000000000 ) ) ;
#7720=EDGE_CURVE ( 'NONE', #89141, #24992, #59661, .T. ) ;
#7722=EDGE_CURVE ( 'NONE', #39851, #49577, #67264, .T. ) ;
#7733=ORIENTED_EDGE ( 'NONE', *, *, #35766, .T. ) ;
#7750=ORIENTED_EDGE ( 'NONE', *, *, #72944, .F. ) ;
#7757=ORIENTED_EDGE ( 'NONE', *, *, #60013, .T. ) ;
#7760=ORIENTED_EDGE ( 'NONE', *, *, #8954, .F. ) ;
#7771=FACE_BOUND ( 'NONE', #46629, .T. ) ;
#7782=CARTESIAN_POINT ( 'NONE',  ( 175.2296996224749250, 215.0000000000000568, -24.99999999999999289 ) ) ;
#7785=CARTESIAN_POINT ( 'NONE',  ( 152.0840361487231860, 129.8837617311558290, 12.49999999999999822 ) ) ;
#7788=ADVANCED_FACE ( 'NONE', ( #36462 ), #44488, .T. ) ;
#7789=DIRECTION ( 'NONE',  ( -1.000000000000000000, 0.000000000000000000, -0.000000000000000000 ) ) ;
#7793=CARTESIAN_POINT ( 'NONE',  ( 201.2104617360081704, 15.00000000000000000, -10.00000000000000000 ) ) ;
#7835=AXIS2_PLACEMENT_3D ( 'NONE', #60451, #30161, #66613 ) ;
#7860=ORIENTED_EDGE ( 'NONE', *, *, #59380, .T. ) ;
#7861=DIRECTION ( 'NONE',  ( -0.000000000000000000, -1.000000000000000000, -0.000000000000000000 ) ) ;
#7862=ADVANCED_FACE ( 'NONE', ( #88504 ), #81436, .T. ) ;
#7868=DIRECTION ( 'NONE',  ( 0.000000000000000000, 0.000000000000000000, 1.000000000000000000 ) ) ;
#7869=CARTESIAN_POINT ( 'NONE',  ( 175.2296996224750103, 275.5000000000000568, 0.000000000000000000 ) ) ;
#7871=ORIENTED_EDGE ( 'NONE', *, *, #31927, .T. ) ;
#7874=ORIENTED_EDGE ( 'NONE', *, *, #47697, .T. ) ;
#7884=AXIS2_PLACEMENT_3D ( 'NONE', #25803, #76484, #69842 ) ;
#7887=AXIS2_PLACEMENT_3D ( 'NONE', #8841, #66625, #1749 ) ;
#7890=CARTESIAN_POINT ( 'NONE',  ( 196.5838024899613856, 20.48082335702326873, 13.01360888346138367 ) ) ;
#7891=AXIS2_PLACEMENT_3D ( 'NONE', #79436, #65710, #822 ) ;
#7892=LINE ( 'NONE', #92669, #77655 ) ;
#7894=VECTOR ( 'NONE', #56981, 1000.000000000000000 ) ;
#7908=CARTESIAN_POINT ( 'NONE',  ( 161.2244399300530233, 8.542400036368780647, 25.74970488511327815 ) ) ;
#7914=CARTESIAN_POINT ( 'NONE',  ( 209.5027106082920056, 29.50523358103493621, 14.69807322781335479 ) ) ;
#7917=CARTESIAN_POINT ( 'NONE',  ( 156.1449889021179160, 215.0000000000000568, 16.91223866672558529 ) ) ;
#7928=EDGE_CURVE ( 'NONE', #75392, #14315, #38307, .T. ) ;
#7931=ORIENTED_EDGE ( 'NONE', *, *, #29868, .F. ) ;
#7932=CARTESIAN_POINT ( 'NONE',  ( 197.1016235222741670, 72.78816326493900135, 12.11671654626785433 ) ) ;
#7945=CARTESIAN_POINT ( 'NONE',  ( 195.7340404941960514, 41.37717207137899322, 12.47808917857981470 ) ) ;
#7949=ADVANCED_FACE ( 'NONE', ( #46795 ), #81393, .F. ) ;
#7955=CIRCLE ( 'NONE', #60888, 7.999911143031724237 ) ;
#7957=DIRECTION ( 'NONE',  ( 1.000000000000000000, 0.000000000000000000, 0.000000000000000000 ) ) ;
#7958=CARTESIAN_POINT ( 'NONE',  ( 139.1539576904058606, 249.5000000000000568, 10.50000000000000000 ) ) ;
#7963=CIRCLE ( 'NONE', #481, 25.50000000000000355 ) ;
#7967=CIRCLE ( 'NONE', #68461, 5.568361562975243650 ) ;
#7989=AXIS2_PLACEMENT_3D ( 'NONE', #83286, #83760, #3773 ) ;
#8003=B_SPLINE_CURVE_WITH_KNOTS ( 'NONE', 3,
 ( #24027, #10747, #33002, #60041, #39148, #61893, #40083, #68528 ),
 .UNSPECIFIED., .F., .F.,
 ( 4, 2, 2, 4 ),
 ( 0.000000000000000000, 0.0004662050538968414977, 0.0009324101077936829953, 0.001864820215587370978 ),
 .UNSPECIFIED. ) ;
#8011=CARTESIAN_POINT ( 'NONE',  ( 153.2628468892384603, 20.37991841447902175, -11.93555113919331134 ) ) ;
#8019=DIRECTION ( 'NONE',  ( 0.000000000000000000, 0.000000000000000000, -1.000000000000000000 ) ) ;
#8025=FACE_OUTER_BOUND ( 'NONE', #2498, .T. ) ;
#8050=VERTEX_POINT ( 'NONE', #33077 ) ;
#8051=DIRECTION ( 'NONE',  ( 0.000000000000000000, 1.000000000000000000, 0.000000000000000000 ) ) ;
#8054=DIRECTION ( 'NONE',  ( 0.000000000000000000, 1.000000000000000000, 0.000000000000000000 ) ) ;
#8067=CARTESIAN_POINT ( 'NONE',  ( 159.4851178187871312, 0.000000000000000000, -10.00000000000000000 ) ) ;
#8068=ADVANCED_FACE ( 'NONE', ( #17486 ), #64264, .T. ) ;
#8072=CARTESIAN_POINT ( 'NONE',  ( 0.000000000000000000, 3.000000000000000000, -9.000000000000001776 ) ) ;
#8073=EDGE_CURVE ( 'NONE', #14859, #53738, #38773, .T. ) ;
#8082=VERTEX_POINT ( 'NONE', #3259 ) ;
#8093=AXIS2_PLACEMENT_3D ( 'NONE', #41524, #78014, #78473 ) ;
#8105=AXIS2_PLACEMENT_3D ( 'NONE', #49950, #85929, #42850 ) ;
#8111=ORIENTED_EDGE ( 'NONE', *, *, #51306, .T. ) ;
#8112=CARTESIAN_POINT ( 'NONE',  ( 195.0876680567968720, 25.98883653703275343, 13.48929546537064716 ) ) ;
#8114=CIRCLE ( 'NONE', #54944, 1.000000000000000888 ) ;
#8124=CIRCLE ( 'NONE', #3589, 0.5000000000000001110 ) ;
#8131=TOROIDAL_SURFACE ( 'NONE', #58033, 1.000000000000000000, 0.5000000000000000000 ) ;
#8139=CARTESIAN_POINT ( 'NONE',  ( 195.8126787625682539, 24.45293242576443049, 12.34923435822822491 ) ) ;
#8147=CYLINDRICAL_SURFACE ( 'NONE', #60424, 7.999911143031724237 ) ;
#8150=LINE ( 'NONE', #35655, #7894 ) ;
#8151=CARTESIAN_POINT ( 'NONE',  ( 221.0059830678134460, 1.828427124746190069, -9.000000000000001776 ) ) ;
#8160=EDGE_CURVE ( 'NONE', #2170, #72022, #58227, .T. ) ;
#8161=ORIENTED_EDGE ( 'NONE', *, *, #86265, .T. ) ;
#8162=CIRCLE ( 'NONE', #41395, 24.49999999999999645 ) ;
#8170=CIRCLE ( 'NONE', #85287, 1.500000000000001332 ) ;
#8179=AXIS2_PLACEMENT_3D ( 'NONE', #70479, #40148, #83246 ) ;
#8185=DIRECTION ( 'NONE',  ( 0.000000000000000000, 0.000000000000000000, 1.000000000000000000 ) ) ;
#8187=VECTOR ( 'NONE', #47932, 1000.000000000000000 ) ;
#8198=VECTOR ( 'NONE', #46, 1000.000000000000114 ) ;
#8199=EDGE_CURVE ( 'NONE', #69835, #6120, #61050, .T. ) ;
#8205=ORIENTED_EDGE ( 'NONE', *, *, #46440, .T. ) ;
#8208=EDGE_CURVE ( 'NONE', #13153, #31, #3788, .T. ) ;
#8232=ORIENTED_EDGE ( 'NONE', *, *, #29223, .T. ) ;
#8244=DIRECTION ( 'NONE',  ( 0.000000000000000000, 0.000000000000000000, 1.000000000000000000 ) ) ;
#8256=DIRECTION ( 'NONE',  ( 0.000000000000000000, 0.000000000000000000, 1.000000000000000000 ) ) ;
#8259=CARTESIAN_POINT ( 'NONE',  ( 197.7335303680046650, 24.96166607582781083, 12.00000000000000000 ) ) ;
#8261=CARTESIAN_POINT ( 'NONE',  ( 155.5427215445352260, 17.93151222991595262, -8.507834038805324184 ) ) ;
#8299=CARTESIAN_POINT ( 'NONE',  ( 204.6539576904058606, 291.1800221208779931, 7.500000000000000000 ) ) ;
#8314=ADVANCED_FACE ( 'NONE', ( #68606 ), #28007, .T. ) ;
#8329=CIRCLE ( 'NONE', #61276, 24.00000000000001066 ) ;
#8335=ORIENTED_EDGE ( 'NONE', *, *, #50291, .T. ) ;
#8336=CARTESIAN_POINT ( 'NONE',  ( 196.0143093133015384, 250.0000000000000568, -11.99999999999998579 ) ) ;
#8341=DIRECTION ( 'NONE',  ( 0.000000000000000000, 1.000000000000000000, 0.000000000000000000 ) ) ;
#8342=CARTESIAN_POINT ( 'NONE',  ( 204.6539576904058606, 293.9636489450775230, 0.000000000000000000 ) ) ;
#8347=ORIENTED_EDGE ( 'NONE', *, *, #81598, .F. ) ;
#8348=CARTESIAN_POINT ( 'NONE',  ( 140.6539576904058606, 276.0000000000000568, 12.00000000000000000 ) ) ;
#8361=EDGE_CURVE ( 'NONE', #36764, #61449, #64332, .T. ) ;
#8362=ADVANCED_FACE ( 'NONE', ( #11305 ), #62694, .F. ) ;
#8371=CARTESIAN_POINT ( 'NONE',  ( 158.6539576904058606, 293.9636489450775230, -11.60392986742922261 ) ) ;
#8372=CARTESIAN_POINT ( 'NONE',  ( 219.8344101925596021, 35.72494958537217968, 7.000000000000000000 ) ) ;
#8386=DIRECTION ( 'NONE',  ( -1.000000000000000000, 0.000000000000000000, 0.000000000000000000 ) ) ;
#8391=AXIS2_PLACEMENT_3D ( 'NONE', #85547, #6957, #19286 ) ;
#8403=CARTESIAN_POINT ( 'NONE',  ( 198.5371898822048990, 65.94618789579841689, 10.76511267510459824 ) ) ;
#8405=CYLINDRICAL_SURFACE ( 'NONE', #30851, 9.550761578869391144 ) ;
#8425=LINE ( 'NONE', #65768, #63973 ) ;
#8430=ORIENTED_EDGE ( 'NONE', *, *, #78193, .F. ) ;
#8443=CARTESIAN_POINT ( 'NONE',  ( 175.2296996224750103, 149.6461846693799487, 0.000000000000000000 ) ) ;
#8455=CARTESIAN_POINT ( 'NONE',  ( 198.0541817046291726, 70.37814311852002902, -10.52985504265800643 ) ) ;
#8457=CONICAL_SURFACE ( 'NONE', #71822, 9.550761578869391144, 0.7853981633974327359 ) ;
#8462=CARTESIAN_POINT ( 'NONE',  ( 196.4653187812577926, 42.25725872477071476, 13.19426264048105146 ) ) ;
#8476=EDGE_CURVE ( 'NONE', #10127, #10282, #49163, .T. ) ;
#8511=ORIENTED_EDGE ( 'NONE', *, *, #62646, .F. ) ;
#8512=CARTESIAN_POINT ( 'NONE',  ( 170.2305261370685798, 214.9910457053126720, -24.90909090909089940 ) ) ;
#8524=ORIENTED_EDGE ( 'NONE', *, *, #72006, .F. ) ;
#8531=CARTESIAN_POINT ( 'NONE',  ( 160.5350683151633291, 250.0000000000000568, 20.22542485937379908 ) ) ;
#8547=ORIENTED_EDGE ( 'NONE', *, *, #17570, .F. ) ;
#8555=DIRECTION ( 'NONE',  ( 0.000000000000000000, -0.000000000000000000, 1.000000000000000000 ) ) ;
#8560=ORIENTED_EDGE ( 'NONE', *, *, #77692, .F. ) ;
#8567=ORIENTED_EDGE ( 'NONE', *, *, #20400, .F. ) ;
#8568=CARTESIAN_POINT ( 'NONE',  ( 185.4166944662832179, 275.5000000000000568, 23.37680765314684450 ) ) ;
#8585=ORIENTED_EDGE ( 'NONE', *, *, #72108, .F. ) ;
#8590=EDGE_CURVE ( 'NONE', #43024, #6020, #40054, .T. ) ;
#8593=CARTESIAN_POINT ( 'NONE',  ( 165.0427047786672290, 276.0000000000000568, 23.37680765314704701 ) ) ;
#8599=DIRECTION ( 'NONE',  ( 0.000000000000000000, 0.000000000000000000, -1.000000000000000000 ) ) ;
#8601=CARTESIAN_POINT ( 'NONE',  ( 175.2296996224750103, 250.0000000000000568, 0.000000000000000000 ) ) ;
#8605=EDGE_CURVE ( 'NONE', #86359, #36583, #93010, .T. ) ;
#8615=ORIENTED_EDGE ( 'NONE', *, *, #41537, .T. ) ;
#8619=LINE ( 'NONE', #17606, #23128 ) ;
#8631=CARTESIAN_POINT ( 'NONE',  ( 197.1659783536655937, 296.4152130614111798, -7.628516150743300805 ) ) ;
#8634=DIRECTION ( 'NONE',  ( 0.000000000000000000, 0.000000000000000000, -1.000000000000000000 ) ) ;
#8647=ORIENTED_EDGE ( 'NONE', *, *, #11869, .T. ) ;
#8650=ORIENTED_EDGE ( 'NONE', *, *, #84782, .F. ) ;
#8660=ORIENTED_EDGE ( 'NONE', *, *, #28307, .T. ) ;
#8671=ORIENTED_EDGE ( 'NONE', *, *, #12784, .F. ) ;
#8678=ORIENTED_EDGE ( 'NONE', *, *, #608, .T. ) ;
#8679=DIRECTION ( 'NONE',  ( 0.000000000000000000, 0.000000000000000000, 1.000000000000000000 ) ) ;
#8682=ORIENTED_EDGE ( 'NONE', *, *, #9521, .T. ) ;
#8683=EDGE_CURVE ( 'NONE', #15791, #85642, #28371, .T. ) ;
#8693=DIRECTION ( 'NONE',  ( -1.000000000000000000, 0.000000000000000000, -5.880589007913310608E-16 ) ) ;
#8698=FACE_OUTER_BOUND ( 'NONE', #73906, .T. ) ;
#8701=EDGE_CURVE ( 'NONE', #20790, #57747, #14610, .T. ) ;
#8706=DIRECTION ( 'NONE',  ( -0.000000000000000000, -0.000000000000000000, -1.000000000000000000 ) ) ;
#8717=DIRECTION ( 'NONE',  ( 0.4995866236608238475, 0.04065491159389757192, -0.8653094149623422604 ) ) ;
#8722=EDGE_CURVE ( 'NONE', #19459, #80899, #30756, .T. ) ;
#8734=DIRECTION ( 'NONE',  ( -0.000000000000000000, -1.000000000000000000, -0.000000000000000000 ) ) ;
#8766=EDGE_CURVE ( 'NONE', #46489, #88967, #57675, .T. ) ;
#8770=VECTOR ( 'NONE', #47401, 1000.000000000000000 ) ;
#8786=ORIENTED_EDGE ( 'NONE', *, *, #78611, .F. ) ;
#8787=DIRECTION ( 'NONE',  ( 0.9998346970812741485, 0.000000000000000000, -0.01818181818182024179 ) ) ;
#8792=DIRECTION ( 'NONE',  ( 0.000000000000000000, 0.000000000000000000, 1.000000000000000000 ) ) ;
#8793=CARTESIAN_POINT ( 'NONE',  ( 152.4536156746142410, 250.5000000000000568, -12.49999999999999289 ) ) ;
#8799=FACE_OUTER_BOUND ( 'NONE', #26686, .T. ) ;
#8827=ADVANCED_FACE ( 'NONE', ( #53218 ), #76107, .T. ) ;
#8828=CARTESIAN_POINT ( 'NONE',  ( 209.1374487190023501, 30.94653725228601715, 14.00000000000000000 ) ) ;
#8838=DIRECTION ( 'NONE',  ( 0.000000000000000000, 0.000000000000000000, 1.000000000000000000 ) ) ;
#8841=CARTESIAN_POINT ( 'NONE',  ( 169.7306087885279169, 250.0000000000000568, -24.89999999999998792 ) ) ;
#8855=CARTESIAN_POINT ( 'NONE',  ( 197.5215339232793497, 69.56983351252434034, 11.61569241699052668 ) ) ;
#8857=CARTESIAN_POINT ( 'NONE',  ( 175.2296996224750103, 161.0000000000000853, 9.550761578869391144 ) ) ;
#8888=EDGE_CURVE ( 'NONE', #15166, #65093, #21683, .T. ) ;
#8898=DIRECTION ( 'NONE',  ( 0.7071067811864494290, 0.000000000000000000, 0.7071067811866457165 ) ) ;
#8901=CARTESIAN_POINT ( 'NONE',  ( 210.1640492649794396, 37.84931640281016030, 12.09245862095555601 ) ) ;
#8915=ORIENTED_EDGE ( 'NONE', *, *, #22733, .T. ) ;
#8916=EDGE_LOOP ( 'NONE', ( #62121, #48444, #85753, #28821 ) ) ;
#8917=LINE ( 'NONE', #55761, #51880 ) ;
#8930=DIRECTION ( 'NONE',  ( -1.000000000000000000, 0.000000000000000000, 0.000000000000000000 ) ) ;
#8939=CARTESIAN_POINT ( 'NONE',  ( 189.4188515237862589, 293.9636489450775798, -40.00000000000000711 ) ) ;
#8943=CARTESIAN_POINT ( 'NONE',  ( 156.8934089303672295, 250.0000000000000568, 16.24901362097164537 ) ) ;
#8945=DIRECTION ( 'NONE',  ( -0.000000000000000000, -1.000000000000000000, -0.000000000000000000 ) ) ;
#8954=EDGE_CURVE ( 'NONE', #65891, #13595, #89658, .T. ) ;
#8967=ORIENTED_EDGE ( 'NONE', *, *, #45431, .T. ) ;
#8968=CARTESIAN_POINT ( 'NONE',  ( 208.6208076322478746, 32.98517505407394168, 9.000000000000001776 ) ) ;
#8971=PLANE ( 'NONE',  #54959 ) ;
#8974=ADVANCED_FACE ( 'NONE', ( #75020 ), #50560, .F. ) ;
#8981=ORIENTED_EDGE ( 'NONE', *, *, #74020, .T. ) ;
#8984=FACE_OUTER_BOUND ( 'NONE', #61925, .T. ) ;
#8985=LINE ( 'NONE', #89443, #85958 ) ;
#8991=EDGE_CURVE ( 'NONE', #2063, #10842, #91378, .T. ) ;
#9011=DIRECTION ( 'NONE',  ( 0.000000000000000000, 1.000000000000000000, 0.000000000000000000 ) ) ;
#9022=EDGE_LOOP ( 'NONE', ( #77636, #3269, #47700, #15442 ) ) ;
#9023=CARTESIAN_POINT ( 'NONE',  ( 207.5220701109484764, 35.61982174545049418, 14.46441793359389472 ) ) ;
#9028=AXIS2_PLACEMENT_3D ( 'NONE', #32266, #18061, #54037 ) ;
#9043=CARTESIAN_POINT ( 'NONE',  ( 159.4851178187871312, 3.000000000000000000, 10.00000000000000000 ) ) ;
#9045=CARTESIAN_POINT ( 'NONE',  ( 194.7559826945684165, 25.47273943569134858, 13.95515289467987152 ) ) ;
#9053=LINE ( 'NONE', #45036, #84600 ) ;
#9070=CARTESIAN_POINT ( 'NONE',  ( 154.5625123364532101, 276.0000000000000568, 13.15740740740740655 ) ) ;
#9082=CARTESIAN_POINT ( 'NONE',  ( 156.4851178187871312, 15.09609934344202387, 9.999999999995333511 ) ) ;
#9083=EDGE_CURVE ( 'NONE', #36747, #82861, #28330, .T. ) ;
#9085=TOROIDAL_SURFACE ( 'NONE', #49933, 24.50000000000000355, 0.5000000000000000000 ) ;
#9087=DIRECTION ( 'NONE',  ( 0.000000000000000000, 1.000000000000000000, 0.000000000000000000 ) ) ;
#9102=ORIENTED_EDGE ( 'NONE', *, *, #63994, .F. ) ;
#9105=ORIENTED_EDGE ( 'NONE', *, *, #470, .T. ) ;
#9108=EDGE_CURVE ( 'NONE', #19715, #38465, #78975, .T. ) ;
#9116=ORIENTED_EDGE ( 'NONE', *, *, #65647, .F. ) ;
#9126=ORIENTED_EDGE ( 'NONE', *, *, #65006, .F. ) ;
#9138=ORIENTED_EDGE ( 'NONE', *, *, #6687, .T. ) ;
#9159=TOROIDAL_SURFACE ( 'NONE', #62106, 1.500000000000000000, 0.5000000000000000000 ) ;
#9162=CARTESIAN_POINT ( 'NONE',  ( 153.9133111279456045, 20.47222690886500729, 13.06183683676587037 ) ) ;
#9166=DIRECTION ( 'NONE',  ( -0.000000000000000000, -1.000000000000000000, -0.000000000000000000 ) ) ;
#9170=DIRECTION ( 'NONE',  ( 0.000000000000000000, 0.000000000000000000, 1.000000000000000000 ) ) ;
#9183=B_SPLINE_CURVE_WITH_KNOTS ( 'NONE', 3,
 ( #10455, #40722, #9994, #32250, #67773, #40257 ),
 .UNSPECIFIED., .F., .F.,
 ( 4, 2, 4 ),
 ( 0.000000000000000000, 0.001358919387270749205, 0.002717838774541498411 ),
 .UNSPECIFIED. ) ;
#9184=ORIENTED_EDGE ( 'NONE', *, *, #25508, .T. ) ;
#9188=CARTESIAN_POINT ( 'NONE',  ( 210.8848006936870263, 293.9636489450776367, -54.00000000000000000 ) ) ;
#9191=CARTESIAN_POINT ( 'NONE',  ( 156.1760182705795899, 20.00000000000000355, -14.66829968254867111 ) ) ;
#9209=CARTESIAN_POINT ( 'NONE',  ( 201.0592549708491958, 40.73798607845790798, 10.50000000000000000 ) ) ;
#9221=VERTEX_POINT ( 'NONE', #2117 ) ;
#9225=EDGE_CURVE ( 'NONE', #74598, #10872, #52749, .T. ) ;
#9233=CONICAL_SURFACE ( 'NONE', #21421, 8.550761578869359170, 0.7853981633974639331 ) ;
#9245=ORIENTED_EDGE ( 'NONE', *, *, #50089, .F. ) ;
#9246=DIRECTION ( 'NONE',  ( 0.000000000000000000, 0.000000000000000000, 1.000000000000000000 ) ) ;
#9253=DIRECTION ( 'NONE',  ( 0.000000000000000000, -0.000000000000000000, 1.000000000000000000 ) ) ;
#9258=ORIENTED_EDGE ( 'NONE', *, *, #17906, .F. ) ;
#9271=CYLINDRICAL_SURFACE ( 'NONE', #68592, 7.500000000000013323 ) ;
#9280=DIRECTION ( 'NONE',  ( 0.000000000000000000, 1.000000000000000000, 0.000000000000000000 ) ) ;
#9281=CARTESIAN_POINT ( 'NONE',  ( 201.2104617360081704, 15.00000000000000000, 10.00000000000000000 ) ) ;
#9294=VECTOR ( 'NONE', #62190, 1000.000000000000000 ) ;
#9298=CARTESIAN_POINT ( 'NONE',  ( 193.9343195356973126, 214.9970011440366875, 17.23862273017082458 ) ) ;
#9301=DIRECTION ( 'NONE',  ( 0.000000000000000000, 0.000000000000000000, 1.000000000000000000 ) ) ;
#9303=CIRCLE ( 'NONE', #30486, 4.999999999999986677 ) ;
#9315=ORIENTED_EDGE ( 'NONE', *, *, #25921, .F. ) ;
#9316=LINE ( 'NONE', #67112, #28797 ) ;
#9318=CARTESIAN_POINT ( 'NONE',  ( 204.6539576904058606, 300.2961574867697436, -4.888549259831427740 ) ) ;
#9329=ORIENTED_EDGE ( 'NONE', *, *, #40401, .T. ) ;
#9344=ORIENTED_EDGE ( 'NONE', *, *, #48992, .T. ) ;
#9361=EDGE_CURVE ( 'NONE', #49098, #200, #83490, .T. ) ;
#9363=DIRECTION ( 'NONE',  ( 0.7806247497998687335, 0.000000000000000000, 0.6249999999999139577 ) ) ;
#9365=CARTESIAN_POINT ( 'NONE',  ( 211.1232656141943949, 0.000000000000000000, -7.000000000000000000 ) ) ;
#9373=FACE_OUTER_BOUND ( 'NONE', #57966, .T. ) ;
#9375=AXIS2_PLACEMENT_3D ( 'NONE', #65024, #22357, #14810 ) ;
#9403=DIRECTION ( 'NONE',  ( 0.000000000000000000, 0.000000000000000000, 1.000000000000000000 ) ) ;
#9409=FACE_OUTER_BOUND ( 'NONE', #43730, .T. ) ;
#9420=CARTESIAN_POINT ( 'NONE',  ( 206.9189553108847406, 30.70889394204682787, 14.50000000000000000 ) ) ;
#9429=CIRCLE ( 'NONE', #62386, 1.000000000000000000 ) ;
#9431=VERTEX_POINT ( 'NONE', #47514 ) ;
#9432=CARTESIAN_POINT ( 'NONE',  ( 203.5977283565847813, 62.01285785379747040, -6.999999999999999112 ) ) ;
#9441=VECTOR ( 'NONE', #91403, 1000.000000000000000 ) ;
#9445=ORIENTED_EDGE ( 'NONE', *, *, #54191, .F. ) ;
#9449=CARTESIAN_POINT ( 'NONE',  ( 160.5350683151633291, 250.0000000000000568, 24.72542485937378842 ) ) ;
#9450=B_SPLINE_CURVE_WITH_KNOTS ( 'NONE', 3,
 ( #30884, #59299, #60235, #88619, #23766, #44605, #75359, #53098, #9544, #52631, #81511, #80589, #38430, #2919, #31347, #45056 ),
 .UNSPECIFIED., .F., .F.,
 ( 4, 2, 2, 2, 2, 2, 2, 4 ),
 ( 0.000000000000000000, 0.0005475143912465603533, 0.001095028782493120707, 0.001642543173739681060, 0.002190057564986241413, 0.002737571956232801550, 0.003285086347479362120, 0.004380115129972482826 ),
 .UNSPECIFIED. ) ;
#9461=CIRCLE ( 'NONE', #59449, 2.999999999999999556 ) ;
#9462=ORIENTED_EDGE ( 'NONE', *, *, #83602, .F. ) ;
#9470=ORIENTED_EDGE ( 'NONE', *, *, #74672, .F. ) ;
#9477=DIRECTION ( 'NONE',  ( -0.000000000000000000, -1.000000000000000000, -0.000000000000000000 ) ) ;
#9488=EDGE_LOOP ( 'NONE', ( #43064, #86296, #46913, #72753 ) ) ;
#9491=AXIS2_PLACEMENT_3D ( 'NONE', #53186, #17220, #27472 ) ;
#9505=VECTOR ( 'NONE', #81174, 1000.000000000000000 ) ;
#9515=CARTESIAN_POINT ( 'NONE',  ( 196.2226125757317163, 24.40159866106579400, 11.63920816608860243 ) ) ;
#9521=EDGE_CURVE ( 'NONE', #30328, #76803, #33724, .T. ) ;
#9524=CARTESIAN_POINT ( 'NONE',  ( 152.4536156746142410, 250.5000000000000568, 12.00000000000000000 ) ) ;
#9527=FACE_BOUND ( 'NONE', #57454, .T. ) ;
#9530=CARTESIAN_POINT ( 'NONE',  ( 198.4456942626906368, 41.56718807020170203, 10.77776320379719444 ) ) ;
#9531=LINE ( 'NONE', #58823, #50347 ) ;
#9544=CARTESIAN_POINT ( 'NONE',  ( 195.9349804655796277, 25.71257817237890109, 14.38313153394006605 ) ) ;
#9560=CARTESIAN_POINT ( 'NONE',  ( 197.2116943569230045, 215.0000000000000568, -12.92446933126075592 ) ) ;
#9562=CIRCLE ( 'NONE', #86690, 20.15985230015483154 ) ;
#9576=EDGE_LOOP ( 'NONE', ( #65271, #50235, #69335, #68879 ) ) ;
#9579=ORIENTED_EDGE ( 'NONE', *, *, #74557, .T. ) ;
#9590=ORIENTED_EDGE ( 'NONE', *, *, #40721, .F. ) ;
#9593=CIRCLE ( 'NONE', #50435, 0.4999999999999977796 ) ;
#9606=AXIS2_PLACEMENT_3D ( 'NONE', #967, #1417, #66755 ) ;
#9610=VERTEX_POINT ( 'NONE', #25736 ) ;
#9611=CARTESIAN_POINT ( 'NONE',  ( 139.6539576904058606, 131.4142135623731633, -11.08578643762690241 ) ) ;
#9615=ORIENTED_EDGE ( 'NONE', *, *, #53799, .F. ) ;
#9627=FACE_OUTER_BOUND ( 'NONE', #58900, .T. ) ;
#9632=CARTESIAN_POINT ( 'NONE',  ( 152.4536156746142410, 250.5000000000000568, 14.50000000000000000 ) ) ;
#9639=CARTESIAN_POINT ( 'NONE',  ( 202.9738562182569694, 293.9636489450776367, 3.999999999999991562 ) ) ;
#9640=CARTESIAN_POINT ( 'NONE',  ( 195.1071592636706384, 20.05007635861079152, 15.17306086504857809 ) ) ;
#9645=DIRECTION ( 'NONE',  ( 0.000000000000000000, 0.000000000000000000, 1.000000000000000000 ) ) ;
#9647=TOROIDAL_SURFACE ( 'NONE', #47489, 4.499999999999993783, 0.5000000000000000000 ) ;
#9648=FACE_OUTER_BOUND ( 'NONE', #1331, .T. ) ;
#9650=DIRECTION ( 'NONE',  ( 0.9764705882352960886, -0.000000000000000000, 0.2156506209390900708 ) ) ;
#9654=DIRECTION ( 'NONE',  ( -0.9531768234071978929, 0.3024135303179465439, 0.000000000000000000 ) ) ;
#9658=AXIS2_PLACEMENT_3D ( 'NONE', #77093, #12223, #62916 ) ;
#9671=CARTESIAN_POINT ( 'NONE',  ( 154.7659666677360235, 19.56018909072649237, -12.94946946942526189 ) ) ;
#9676=VECTOR ( 'NONE', #78988, 1000.000000000000000 ) ;
#9690=DIRECTION ( 'NONE',  ( 0.000000000000000000, 0.000000000000000000, 1.000000000000000000 ) ) ;
#9704=ORIENTED_EDGE ( 'NONE', *, *, #61720, .F. ) ;
#9721=EDGE_LOOP ( 'NONE', ( #25196, #9470, #34189, #26568 ) ) ;
#9727=ORIENTED_EDGE ( 'NONE', *, *, #47895, .F. ) ;
#9728=CARTESIAN_POINT ( 'NONE',  ( 199.0029451100810434, 66.39899626990381876, -8.059931973035714847 ) ) ;
#9730=CIRCLE ( 'NONE', #62695, 0.5000000000000003331 ) ;
#9733=CIRCLE ( 'NONE', #46017, 24.50000000000001066 ) ;
#9737=CARTESIAN_POINT ( 'NONE',  ( 197.9812641850257080, 65.99374301882849636, -9.931412343739248527 ) ) ;
#9740=AXIS2_PLACEMENT_3D ( 'NONE', #55474, #70624, #54991 ) ;
#9747=EDGE_CURVE ( 'NONE', #15079, #15987, #41264, .T. ) ;
#9767=FACE_OUTER_BOUND ( 'NONE', #36839, .T. ) ;
#9771=EDGE_CURVE ( 'NONE', #80899, #38465, #26144, .T. ) ;
#9812=VERTEX_POINT ( 'NONE', #84430 ) ;
#9813=CARTESIAN_POINT ( 'NONE',  ( 196.1089143772224759, 40.84001755061112959, 13.20492811982817294 ) ) ;
#9822=CARTESIAN_POINT ( 'NONE',  ( 209.3190042249899250, 30.23012903947020646, 14.26380412667039010 ) ) ;
#9827=ORIENTED_EDGE ( 'NONE', *, *, #69553, .F. ) ;
#9840=DIRECTION ( 'NONE',  ( 0.9167375550253826777, 5.544037366339495023E-15, 0.3994899938747948354 ) ) ;
#9842=EDGE_CURVE ( 'NONE', #4469, #69769, #12576, .T. ) ;
#9844=CARTESIAN_POINT ( 'NONE',  ( 180.5235960634565799, 214.6007075219689000, -24.43326837773227211 ) ) ;
#9845=DIRECTION ( 'NONE',  ( 1.000000000000000000, 0.000000000000000000, 1.224646799147353207E-16 ) ) ;
#9856=ORIENTED_EDGE ( 'NONE', *, *, #89600, .T. ) ;
#9857=ORIENTED_EDGE ( 'NONE', *, *, #56217, .T. ) ;
#9858=CARTESIAN_POINT ( 'NONE',  ( 195.3470921470671158, 40.91257177144665746, 14.84270801981803700 ) ) ;
#9862=EDGE_CURVE ( 'NONE', #33982, #56036, #65525, .T. ) ;
#9872=CARTESIAN_POINT ( 'NONE',  ( 185.0172044724083946, 276.0000000000000568, 22.46007009812148425 ) ) ;
#9873=CARTESIAN_POINT ( 'NONE',  ( 152.4536156746142410, 249.5000000000000568, 12.50000000000000000 ) ) ;
#9881=CARTESIAN_POINT ( 'NONE',  ( 206.1702329640447147, -6.606856988583545110E-17, 7.166221634559009956 ) ) ;
#9895=DIRECTION ( 'NONE',  ( 0.000000000000000000, 1.000000000000000000, 0.000000000000000000 ) ) ;
#9899=DIRECTION ( 'NONE',  ( -1.000000000000000000, -4.095251346825557639E-15, 0.000000000000000000 ) ) ;
#9906=EDGE_CURVE ( 'NONE', #33474, #46837, #71534, .T. ) ;
#9911=DIRECTION ( 'NONE',  ( -0.7957555401921962979, -0.6056179655966504871, 0.000000000000000000 ) ) ;
#9922=ORIENTED_EDGE ( 'NONE', *, *, #31774, .F. ) ;
#9927=DIRECTION ( 'NONE',  ( 0.000000000000000000, 0.000000000000000000, 1.000000000000000000 ) ) ;
#9930=DIRECTION ( 'NONE',  ( -1.000000000000000000, -0.000000000000000000, 0.000000000000000000 ) ) ;
#9944=EDGE_CURVE ( 'NONE', #37492, #55107, #24662, .T. ) ;
#9954=CARTESIAN_POINT ( 'NONE',  ( 183.0442525570908288, 275.0000000000000568, 7.500000000000000000 ) ) ;
#9987=CARTESIAN_POINT ( 'NONE',  ( 197.1034181619488663, 25.84651970789479947, 12.27392387986159505 ) ) ;
#9994=CARTESIAN_POINT ( 'NONE',  ( 155.8725544043011553, 19.96731923950661525, 14.33077026901213635 ) ) ;
#9997=CARTESIAN_POINT ( 'NONE',  ( 175.2296996224750103, 250.0000000000000568, -25.00000000000000355 ) ) ;
#10000=CARTESIAN_POINT ( 'NONE',  ( 200.3789899249135544, 40.95381314121857486, 10.02076201298226721 ) ) ;
#10009=EDGE_CURVE ( 'NONE', #6373, #73562, #22462, .T. ) ;
#10011=EDGE_LOOP ( 'NONE', ( #48919, #75051, #14745, #33558 ) ) ;
#10027=DIRECTION ( 'NONE',  ( 1.000000000000000000, 0.000000000000000000, -0.000000000000000000 ) ) ;
#10030=CARTESIAN_POINT ( 'NONE',  ( 199.2296996224750103, 68.12454877777268791, -4.237361107270372962 ) ) ;
#10048=ORIENTED_EDGE ( 'NONE', *, *, #44981, .T. ) ;
#10065=ADVANCED_FACE ( 'NONE', ( #12482 ), #34266, .F. ) ;
#10071=VERTEX_POINT ( 'NONE', #37702 ) ;
#10079=CARTESIAN_POINT ( 'NONE',  ( 157.4851178187871312, 14.99999999999999467, 7.000000000000000888 ) ) ;
#10094=DIRECTION ( 'NONE',  ( -0.6249999999999938938, -1.734723475976788793E-14, -0.7806247497998048956 ) ) ;
#10097=( BOUNDED_SURFACE ( )  B_SPLINE_SURFACE ( 3, 2, ( 
 ( #58744, #50222, #87133 ),
 ( #22284, #979, #93314 ),
 ( #21351, #57814, #29860 ),
 ( #51606, #43133, #21829 ) ),
 .UNSPECIFIED., .F., .F., .F. ) 
 B_SPLINE_SURFACE_WITH_KNOTS ( ( 4, 4 ),
 ( 3, 3 ),
 ( 1.570796326794896558, 2.004620063563922638 ),
 ( 0.000000000000000000, 1.000000000000000000 ),
 .UNSPECIFIED. ) 
 GEOMETRIC_REPRESENTATION_ITEM ( )  RATIONAL_B_SPLINE_SURFACE ( (
 ( 1.000000000000000000, 0.7071067811865475727, 1.000000000000000000),
 ( 1.000000000000000000, 0.7478056585118743049, 1.000000000000000000),
 ( 1.000000000000000000, 0.7849082635113588946, 1.000000000000000000),
 ( 1.000000000000000000, 0.8168508380123956636, 1.000000000000000000) ) ) 
 REPRESENTATION_ITEM ( '' )  SURFACE ( )  );
#10100=DIRECTION ( 'NONE',  ( 0.000000000000000000, -0.000000000000000000, -1.000000000000000000 ) ) ;
#10106=CARTESIAN_POINT ( 'NONE',  ( 175.2296996224750103, 250.0000000000000568, -12.00000000000000000 ) ) ;
#10107=CARTESIAN_POINT ( 'NONE',  ( 175.2296996224750103, 150.9142415853029036, 0.000000000000000000 ) ) ;
#10112=FACE_OUTER_BOUND ( 'NONE', #4144, .T. ) ;
#10127=VERTEX_POINT ( 'NONE', #74165 ) ;
#10133=DIRECTION ( 'NONE',  ( -1.000000000000000000, 0.000000000000000000, 0.000000000000000000 ) ) ;
#10178=ADVANCED_FACE ( 'NONE', ( #23038 ), #80617, .T. ) ;
#10184=VERTEX_POINT ( 'NONE', #66157 ) ;
#10190=CARTESIAN_POINT ( 'NONE',  ( 197.1858402786432976, 68.15263271079744811, -10.54024884218787861 ) ) ;
#10196=CARTESIAN_POINT ( 'NONE',  ( 194.7453183674699915, 20.99999999999998934, -15.62500000000000355 ) ) ;
#10209=EDGE_CURVE ( 'NONE', #16726, #49537, #91137, .T. ) ;
#10220=DIRECTION ( 'NONE',  ( -0.5877852522924792433, 0.000000000000000000, -0.8090169943749430104 ) ) ;
#10225=DIRECTION ( 'NONE',  ( 0.000000000000000000, 0.000000000000000000, -1.000000000000000000 ) ) ;
#10248=EDGE_CURVE ( 'NONE', #26035, #12543, #85155, .T. ) ;
#10252=CIRCLE ( 'NONE', #76851, 1.000000000000000888 ) ;
#10257=CARTESIAN_POINT ( 'NONE',  ( 203.4339565214082484, 300.2380916213085698, -4.962874975894024487 ) ) ;
#10267=DIRECTION ( 'NONE',  ( -0.000000000000000000, -1.000000000000000000, -0.000000000000000000 ) ) ;
#10271=ADVANCED_FACE ( 'NONE', ( #16872 ), #73066, .T. ) ;
#10277=CARTESIAN_POINT ( 'NONE',  ( 184.5340210998923283, 2.974099043298211953, 8.999832278985701706 ) ) ;
#10278=LINE ( 'NONE', #54305, #52323 ) ;
#10282=VERTEX_POINT ( 'NONE', #67546 ) ;
#10291=ORIENTED_EDGE ( 'NONE', *, *, #15662, .T. ) ;
#10300=CARTESIAN_POINT ( 'NONE',  ( 180.6209651459523968, 214.5000000000000568, -24.41176470588237635 ) ) ;
#10309=CARTESIAN_POINT ( 'NONE',  ( 175.2296996224750103, 133.0000000000000000, 0.000000000000000000 ) ) ;
#10312=ORIENTED_EDGE ( 'NONE', *, *, #29988, .F. ) ;
#10313=EDGE_LOOP ( 'NONE', ( #27297, #14258 ) ) ;
#10314=EDGE_CURVE ( 'NONE', #82861, #22798, #39670, .T. ) ;
#10315=CARTESIAN_POINT ( 'NONE',  ( 175.2296996224750103, 250.0000000000000568, 0.000000000000000000 ) ) ;
#10322=AXIS2_PLACEMENT_3D ( 'NONE', #81885, #74812, #9927 ) ;
#10330=CARTESIAN_POINT ( 'NONE',  ( 175.2296996224750103, 158.6892791692949629, 0.000000000000000000 ) ) ;
#10331=FACE_OUTER_BOUND ( 'NONE', #85263, .T. ) ;
#10343=LINE ( 'NONE', #2791, #62600 ) ;
#10345=CARTESIAN_POINT ( 'NONE',  ( 204.6539576904058606, 296.7472757692770529, -7.500000000000000000 ) ) ;
#10352=FACE_OUTER_BOUND ( 'NONE', #47267, .T. ) ;
#10355=CARTESIAN_POINT ( 'NONE',  ( 207.1352294840503134, 30.54719743553542344, 14.49999997652496475 ) ) ;
#10369=CARTESIAN_POINT ( 'NONE',  ( 175.2296996224750103, 250.0000000000000568, 24.50000000000000355 ) ) ;
#10377=VERTEX_POINT ( 'NONE', #1730 ) ;
#10383=CARTESIAN_POINT ( 'NONE',  ( 156.9788729827742202, 275.8411434044543284, 16.89623125813446336 ) ) ;
#10385=ORIENTED_EDGE ( 'NONE', *, *, #40721, .T. ) ;
#10387=AXIS2_PLACEMENT_3D ( 'NONE', #36103, #92447, #6301 ) ;
#10390=CARTESIAN_POINT ( 'NONE',  ( 195.4192251500433031, 26.20723835156640291, 14.74561642346474777 ) ) ;
#10404=ADVANCED_FACE ( 'NONE', ( #38164 ), #59038, .T. ) ;
#10409=ORIENTED_EDGE ( 'NONE', *, *, #92815, .F. ) ;
#10410=CARTESIAN_POINT ( 'NONE',  ( 208.4306832106271088, 20.44233620800389772, -7.500000000000013323 ) ) ;
#10415=CARTESIAN_POINT ( 'NONE',  ( 198.4290158740602976, 26.16953160995604577, 11.14960445189099048 ) ) ;
#10426=EDGE_LOOP ( 'NONE', ( #61792, #11771, #8647, #7642 ) ) ;
#10447=CIRCLE ( 'NONE', #39229, 1.999999999999988454 ) ;
#10448=CARTESIAN_POINT ( 'NONE',  ( 210.2502938138737250, 0.01288801604375340581, 7.290233312756248196 ) ) ;
#10455=CARTESIAN_POINT ( 'NONE',  ( 156.4947056272797852, 20.00000000000000000, 15.00000000000000000 ) ) ;
#10457=CARTESIAN_POINT ( 'NONE',  ( 197.3748232817348764, 214.9910457053126720, -12.45182892472558756 ) ) ;
#10459=DIRECTION ( 'NONE',  ( 0.000000000000000000, 0.000000000000000000, 1.000000000000000000 ) ) ;
#10460=DIRECTION ( 'NONE',  ( 0.000000000000000000, 0.000000000000000000, -1.000000000000000000 ) ) ;
#10468=ADVANCED_FACE ( 'NONE', ( #73712 ), #80337, .F. ) ;
#10470=ORIENTED_EDGE ( 'NONE', *, *, #87659, .F. ) ;
#10474=DIRECTION ( 'NONE',  ( 0.000000000000000000, 0.000000000000000000, 1.000000000000000000 ) ) ;
#10485=DIRECTION ( 'NONE',  ( 0.000000000000000000, 1.000000000000000000, 0.000000000000000000 ) ) ;
#10486=CARTESIAN_POINT ( 'NONE',  ( 186.6539576904058890, 293.9636489450775230, 0.000000000000000000 ) ) ;
#10488=LINE ( 'NONE', #39356, #16822 ) ;
#10511=CARTESIAN_POINT ( 'NONE',  ( 200.2296996224750387, 68.12454877777268791, -4.413917820073306686 ) ) ;
#10514=CIRCLE ( 'NONE', #72590, 4.500000000000003553 ) ;
#10517=EDGE_LOOP ( 'NONE', ( #40382, #46407, #10652, #28400 ) ) ;
#10520=B_SPLINE_CURVE_WITH_KNOTS ( 'NONE', 3,
 ( #13149, #26404, #41985, #70898, #62881, #6031 ),
 .UNSPECIFIED., .F., .F.,
 ( 4, 2, 4 ),
 ( 5.204170427930421283E-18, 0.0006312149994345400694, 0.001262429998869074935 ),
 .UNSPECIFIED. ) ;
#10521=VECTOR ( 'NONE', #88710, 1000.000000000000000 ) ;
#10530=ORIENTED_EDGE ( 'NONE', *, *, #79777, .T. ) ;
#10538=ORIENTED_EDGE ( 'NONE', *, *, #65821, .F. ) ;
#10539=DIRECTION ( 'NONE',  ( -1.000000000000000000, 0.000000000000000000, 0.000000000000000000 ) ) ;
#10542=ADVANCED_FACE ( 'NONE', ( #9767 ), #88823, .T. ) ;
#10544=EDGE_LOOP ( 'NONE', ( #35103, #40798, #57160, #20694 ) ) ;
#10545=ORIENTED_EDGE ( 'NONE', *, *, #8160, .T. ) ;
#10560=B_SPLINE_CURVE_WITH_KNOTS ( 'NONE', 3,
 ( #18411, #25973, #54857, #33088, #4213, #4674, #61527, #69085 ),
 .UNSPECIFIED., .F., .F.,
 ( 4, 2, 2, 4 ),
 ( 2.845565583954363981E-21, 0.001369958260980387805, 0.002054937391470581382, 0.002739916521960775175 ),
 .UNSPECIFIED. ) ;
#10567=CARTESIAN_POINT ( 'NONE',  ( 221.8344101925596306, 35.72494958537217968, 7.000000000000000000 ) ) ;
#10571=CARTESIAN_POINT ( 'NONE',  ( 184.1778392089217107, 3.000000000000000000, 10.00000000000000178 ) ) ;
#10573=ORIENTED_EDGE ( 'NONE', *, *, #52296, .F. ) ;
#10574=CARTESIAN_POINT ( 'NONE',  ( 156.4851178187871312, 15.09609934344103976, -9.999999999996333599 ) ) ;
#10588=AXIS2_PLACEMENT_3D ( 'NONE', #73851, #44025, #52995 ) ;
#10590=ORIENTED_EDGE ( 'NONE', *, *, #22050, .F. ) ;
#10599=ADVANCED_FACE ( 'NONE', ( #40479 ), #65181, .F. ) ;
#10600=DIRECTION ( 'NONE',  ( 1.000000000000000000, 1.359745199634109878E-15, 0.000000000000000000 ) ) ;
#10615=CARTESIAN_POINT ( 'NONE',  ( 198.5720013812636751, 41.52711472736257292, 11.03083405179678778 ) ) ;
#10628=ORIENTED_EDGE ( 'NONE', *, *, #83917, .T. ) ;
#10630=ORIENTED_EDGE ( 'NONE', *, *, #12020, .T. ) ;
#10646=EDGE_LOOP ( 'NONE', ( #84596, #37762, #15306, #93441 ) ) ;
#10647=( BOUNDED_CURVE ( )  B_SPLINE_CURVE ( 3, ( #32312, #10511, #47424, #4355 ),
 .UNSPECIFIED., .F., .F. ) 
 B_SPLINE_CURVE_WITH_KNOTS ( ( 4, 4 ),
 ( 0.000000000000000000, 0.5235987755982978165 ),
 .UNSPECIFIED. ) 
 CURVE ( )  GEOMETRIC_REPRESENTATION_ITEM ( )  RATIONAL_B_SPLINE_CURVE ( ( 1.000000000000000000, 0.9772838841927122822, 0.9772838841927122822, 1.000000000000000000 ) ) 
 REPRESENTATION_ITEM ( '' )  );
#10652=ORIENTED_EDGE ( 'NONE', *, *, #81790, .T. ) ;
#10653=( BOUNDED_CURVE ( )  B_SPLINE_CURVE ( 3, ( #3134, #32014, #7682, #58822 ),
 .UNSPECIFIED., .F., .F. ) 
 B_SPLINE_CURVE_WITH_KNOTS ( ( 4, 4 ),
 ( 4.712388980384683457, 7.853981633974489007 ),
 .UNSPECIFIED. ) 
 CURVE ( )  GEOMETRIC_REPRESENTATION_ITEM ( )  RATIONAL_B_SPLINE_CURVE ( ( 1.000000000000000000, 0.3333333333333292070, 0.3333333333333292070, 1.000000000000000000 ) ) 
 REPRESENTATION_ITEM ( '' )  );
#10655=AXIS2_PLACEMENT_3D ( 'NONE', #16797, #39017, #52770 ) ;
#10660=CARTESIAN_POINT ( 'NONE',  ( 196.0143093133015384, 73.40565171261609123, -11.99999999999998046 ) ) ;
#10667=CARTESIAN_POINT ( 'NONE',  ( 196.5845095011719081, 20.48014462998423824, -13.01238430412327673 ) ) ;
#10680=CARTESIAN_POINT ( 'NONE',  ( 197.7360402925001779, 68.71846123420905883, 9.407289490885741401 ) ) ;
#10688=CARTESIAN_POINT ( 'NONE',  ( 196.8803347170859865, 42.36571313990103960, 12.49999999999999289 ) ) ;
#10705=EDGE_CURVE ( 'NONE', #41724, #72750, #59560, .T. ) ;
#10721=ORIENTED_EDGE ( 'NONE', *, *, #81598, .T. ) ;
#10724=CARTESIAN_POINT ( 'NONE',  ( 139.1539576904058606, 249.5000000000000568, 12.50000000000000000 ) ) ;
#10725=AXIS2_PLACEMENT_3D ( 'NONE', #88163, #37067, #632 ) ;
#10736=ORIENTED_EDGE ( 'NONE', *, *, #18738, .T. ) ;
#10737=CARTESIAN_POINT ( 'NONE',  ( 165.2494399300530290, 8.542400036368780647, 9.000000000000001776 ) ) ;
#10747=CARTESIAN_POINT ( 'NONE',  ( 153.7799452197002665, 19.44319250842783120, -11.58598955890918702 ) ) ;
#10751=EDGE_LOOP ( 'NONE', ( #69305, #43017 ) ) ;
#10760=ORIENTED_EDGE ( 'NONE', *, *, #93562, .T. ) ;
#10765=DIRECTION ( 'NONE',  ( 0.000000000000000000, -0.000000000000000000, 1.000000000000000000 ) ) ;
#10769=CARTESIAN_POINT ( 'NONE',  ( 198.8852758280538353, 66.55360856415096293, 4.692040283685088298 ) ) ;
#10777=PLANE ( 'NONE',  #80412 ) ;
#10779=ORIENTED_EDGE ( 'NONE', *, *, #70232, .F. ) ;
#10781=CARTESIAN_POINT ( 'NONE',  ( 196.5975808051811669, 18.84406744235270281, 11.77299963048721843 ) ) ;
#10793=VECTOR ( 'NONE', #60490, 1000.000000000000000 ) ;
#10797=DIRECTION ( 'NONE',  ( -0.8786741093294601068, 0.000000000000000000, 0.4774220455677345987 ) ) ;
#10805=CARTESIAN_POINT ( 'NONE',  ( 207.9699384896711933, 0.04196010845019407243, 7.500000000000011546 ) ) ;
#10809=EDGE_CURVE ( 'NONE', #14834, #31737, #27800, .T. ) ;
#10812=DIRECTION ( 'NONE',  ( -0.000000000000000000, -1.000000000000000000, -0.000000000000000000 ) ) ;
#10818=EDGE_CURVE ( 'NONE', #71850, #19571, #80687, .T. ) ;
#10831=VERTEX_POINT ( 'NONE', #3603 ) ;
#10832=CARTESIAN_POINT ( 'NONE',  ( 197.3507970371305476, 24.88295298518901078, 12.40598166297186111 ) ) ;
#10834=DIRECTION ( 'NONE',  ( -0.000000000000000000, -1.000000000000000000, -0.000000000000000000 ) ) ;
#10842=VERTEX_POINT ( 'NONE', #76510 ) ;
#10851=AXIS2_PLACEMENT_3D ( 'NONE', #55757, #77528, #84610 ) ;
#10853=DIRECTION ( 'NONE',  ( -1.000000000000000000, -0.000000000000000000, -0.000000000000000000 ) ) ;
#10854=VECTOR ( 'NONE', #83352, 1000.000000000000000 ) ;
#10855=CARTESIAN_POINT ( 'NONE',  ( 196.4767969875140352, 25.16014212029416086, 13.66798976973107749 ) ) ;
#10861=CIRCLE ( 'NONE', #1751, 4.999999999999990230 ) ;
#10872=VERTEX_POINT ( 'NONE', #68000 ) ;
#10873=ORIENTED_EDGE ( 'NONE', *, *, #70157, .T. ) ;
#10874=CARTESIAN_POINT ( 'NONE',  ( 155.0193446949349152, 20.65816215000725720, -12.95286603764679256 ) ) ;
#10879=CARTESIAN_POINT ( 'NONE',  ( 200.4644824113734387, 214.9910457053126720, -2.942835885954282471 ) ) ;
#10890=VERTEX_POINT ( 'NONE', #76971 ) ;
#10899=DIRECTION ( 'NONE',  ( 0.000000000000000000, 0.000000000000000000, 1.000000000000000000 ) ) ;
#10910=DIRECTION ( 'NONE',  ( 0.000000000000000000, 0.000000000000000000, -1.000000000000000000 ) ) ;
#10912=PLANE ( 'NONE',  #20227 ) ;
#10913=CIRCLE ( 'NONE', #38145, 23.00000000000000711 ) ;
#10916=AXIS2_PLACEMENT_3D ( 'NONE', #29721, #58603, #87444 ) ;
#10920=AXIS2_PLACEMENT_3D ( 'NONE', #13417, #5839, #42262 ) ;
#10922=AXIS2_PLACEMENT_3D ( 'NONE', #60219, #89522, #88131 ) ;
#10924=CARTESIAN_POINT ( 'NONE',  ( 200.7510921130352415, 288.0788353042884751, -5.420371282781244027 ) ) ;
#10926=CARTESIAN_POINT ( 'NONE',  ( 200.1030226942293098, 214.6007075219629030, -2.515500450062353899 ) ) ;
#10939=CARTESIAN_POINT ( 'NONE',  ( 175.2296996224750103, 21.00000000000000000, -15.00000000000000000 ) ) ;
#10942=ADVANCED_FACE ( 'NONE', ( #84060 ), #5006, .T. ) ;
#10943=DIRECTION ( 'NONE',  ( 0.2456588035076310295, -0.9693563597868428694, 0.000000000000000000 ) ) ;
#10954=PLANE ( 'NONE',  #33883 ) ;
#10969=ORIENTED_EDGE ( 'NONE', *, *, #21310, .F. ) ;
#10976=CARTESIAN_POINT ( 'NONE',  ( 195.7317764926344239, 19.56557103583841695, -12.90780099963700600 ) ) ;
#10981=ORIENTED_EDGE ( 'NONE', *, *, #7600, .F. ) ;
#10990=AXIS2_PLACEMENT_3D ( 'NONE', #10309, #3215, #58669 ) ;
#10995=ORIENTED_EDGE ( 'NONE', *, *, #53031, .T. ) ;
#10997=VECTOR ( 'NONE', #33030, 1000.000000000000000 ) ;
#11007=EDGE_CURVE ( 'NONE', #71850, #7049, #81988, .T. ) ;
#11020=CARTESIAN_POINT ( 'NONE',  ( 154.9842916688210153, 275.0000000000000568, 12.88888888888891771 ) ) ;
#11026=CIRCLE ( 'NONE', #71556, 0.9999999999999991118 ) ;
#11028=CARTESIAN_POINT ( 'NONE',  ( 208.4306832106271088, -74.55766379199613425, 0.000000000000000000 ) ) ;
#11035=DIRECTION ( 'NONE',  ( 0.000000000000000000, 1.000000000000000000, 0.000000000000000000 ) ) ;
#11038=CARTESIAN_POINT ( 'NONE',  ( 200.1126601882107252, 250.0000000000000568, -2.416251949619908412 ) ) ;
#11040=CARTESIAN_POINT ( 'NONE',  ( 208.6451419912077085, 38.33121871055298868, 12.00000001296747598 ) ) ;
#11045=CARTESIAN_POINT ( 'NONE',  ( 156.1965750133424251, 18.75975317436470391, -8.718057073926514633 ) ) ;
#11051=CIRCLE ( 'NONE', #51877, 24.00000000000000355 ) ;
#11060=CARTESIAN_POINT ( 'NONE',  ( 209.6287663260175975, 29.00782453271232697, 10.49999999999999822 ) ) ;
#11067=AXIS2_PLACEMENT_3D ( 'NONE', #16409, #31554, #46205 ) ;
#11080=EDGE_CURVE ( 'NONE', #55107, #91332, #46662, .T. ) ;
#11117=ORIENTED_EDGE ( 'NONE', *, *, #56881, .T. ) ;
#11123=ORIENTED_EDGE ( 'NONE', *, *, #266, .F. ) ;
#11128=CIRCLE ( 'NONE', #2090, 2.000000000000000000 ) ;
#11134=DIRECTION ( 'NONE',  ( -1.000000000000000000, -4.095251346825558428E-15, 0.000000000000000000 ) ) ;
#11140=CARTESIAN_POINT ( 'NONE',  ( 208.4306832106271088, 0.000000000000000000, 0.000000000000000000 ) ) ;
#11143=CIRCLE ( 'NONE', #51965, 0.4999999999999989453 ) ;
#11150=DIRECTION ( 'NONE',  ( 0.000000000000000000, 0.000000000000000000, 1.000000000000000000 ) ) ;
#11152=CIRCLE ( 'NONE', #51974, 1.499999999999999556 ) ;
#11162=CYLINDRICAL_SURFACE ( 'NONE', #16418, 0.5000000000000004441 ) ;
#11176=VECTOR ( 'NONE', #86013, 1000.000000000000000 ) ;
#11181=CARTESIAN_POINT ( 'NONE',  ( 150.6539576904058606, 293.9636489450775230, 9.103929867429224387 ) ) ;
#11184=DIRECTION ( 'NONE',  ( 0.000000000000000000, 1.000000000000000000, 0.000000000000000000 ) ) ;
#11195=EDGE_CURVE ( 'NONE', #13726, #23799, #50419, .T. ) ;
#11198=VERTEX_POINT ( 'NONE', #50425 ) ;
#11200=CIRCLE ( 'NONE', #82306, 4.025000000000000355 ) ;
#11202=FACE_OUTER_BOUND ( 'NONE', #10646, .T. ) ;
#11210=CIRCLE ( 'NONE', #91283, 0.5000000000000004441 ) ;
#11229=FACE_OUTER_BOUND ( 'NONE', #45322, .T. ) ;
#11233=ORIENTED_EDGE ( 'NONE', *, *, #64718, .F. ) ;
#11243=VERTEX_POINT ( 'NONE', #63265 ) ;
#11248=CARTESIAN_POINT ( 'NONE',  ( 165.4421947725420523, 275.5000000000000568, 22.46007009812167254 ) ) ;
#11250=CARTESIAN_POINT ( 'NONE',  ( 152.9190334681021000, 20.54289017631687742, 11.30277777986246335 ) ) ;
#11258=EDGE_CURVE ( 'NONE', #26346, #69103, #36834, .T. ) ;
#11261=CARTESIAN_POINT ( 'NONE',  ( 194.5337174367984687, 40.88867648032507418, 14.26073298213507812 ) ) ;
#11264=ORIENTED_EDGE ( 'NONE', *, *, #39673, .F. ) ;
#11265=DIRECTION ( 'NONE',  ( -0.000000000000000000, -1.000000000000000000, -0.000000000000000000 ) ) ;
#11279=DIRECTION ( 'NONE',  ( 0.000000000000000000, 0.000000000000000000, 1.000000000000000000 ) ) ;
#11291=VECTOR ( 'NONE', #52517, 1000.000000000000000 ) ;
#11293=CARTESIAN_POINT ( 'NONE',  ( 199.0061125298537377, 275.0000000000000568, -7.725424859374024678 ) ) ;
#11295=DIRECTION ( 'NONE',  ( 0.000000000000000000, 1.000000000000000000, 0.000000000000000000 ) ) ;
#11301=CARTESIAN_POINT ( 'NONE',  ( 156.4851178187871312, 1.000000000000000000, 10.00000000000000000 ) ) ;
#11305=FACE_OUTER_BOUND ( 'NONE', #69939, .T. ) ;
#11314=ORIENTED_EDGE ( 'NONE', *, *, #62646, .T. ) ;
#11315=DIRECTION ( 'NONE',  ( 0.000000000000000000, 1.000000000000000000, 0.000000000000000000 ) ) ;
#11317=DIRECTION ( 'NONE',  ( 0.000000000000000000, 0.000000000000000000, -1.000000000000000000 ) ) ;
#11326=VERTEX_POINT ( 'NONE', #65136 ) ;
#11336=CARTESIAN_POINT ( 'NONE',  ( 180.2288731078812702, 214.9910457053126720, -24.90909090909092782 ) ) ;
#11337=CARTESIAN_POINT ( 'NONE',  ( 195.5071814400074572, 25.58662921606786256, 14.62325102173291924 ) ) ;
#11345=ORIENTED_EDGE ( 'NONE', *, *, #83721, .F. ) ;
#11350=AXIS2_PLACEMENT_3D ( 'NONE', #60580, #75240, #25502 ) ;
#11356=ORIENTED_EDGE ( 'NONE', *, *, #21572, .F. ) ;
#11357=CARTESIAN_POINT ( 'NONE',  ( 211.1232656141943949, 0.000000000000000000, 7.000000000000000000 ) ) ;
#11363=CARTESIAN_POINT ( 'NONE',  ( 199.5287591260213560, 25.00736135706073426, 9.179409580711885397 ) ) ;
#11367=EDGE_CURVE ( 'NONE', #54755, #91019, #49495, .T. ) ;
#11371=VECTOR ( 'NONE', #41606, 1000.000000000000000 ) ;
#11375=VERTEX_POINT ( 'NONE', #48538 ) ;
#11376=DIRECTION ( 'NONE',  ( 0.000000000000000000, 0.000000000000000000, -1.000000000000000000 ) ) ;
#11395=CARTESIAN_POINT ( 'NONE',  ( 198.5086862847058171, 68.69963673589226971, 12.80442219776277213 ) ) ;
#11409=CARTESIAN_POINT ( 'NONE',  ( 196.7383257810085979, 42.27872732282705925, 11.00000000000000000 ) ) ;
#11410=CARTESIAN_POINT ( 'NONE',  ( 156.4851178187871312, 1.000000000000000000, 10.00000000000000000 ) ) ;
#11420=ORIENTED_EDGE ( 'NONE', *, *, #11662, .T. ) ;
#11429=AXIS2_PLACEMENT_3D ( 'NONE', #55746, #13141, #93571 ) ;
#11435=ADVANCED_FACE ( 'NONE', ( #71766 ), #41903, .F. ) ;
#11437=CARTESIAN_POINT ( 'NONE',  ( 175.2296996224750103, 275.0000000000000568, 0.000000000000000000 ) ) ;
#11452=EDGE_LOOP ( 'NONE', ( #70609, #72394, #40072, #5192 ) ) ;
#11460=CARTESIAN_POINT ( 'NONE',  ( 186.6539576904058890, 293.9636489450775230, -11.60392986742922261 ) ) ;
#11465=ORIENTED_EDGE ( 'NONE', *, *, #84689, .F. ) ;
#11478=ORIENTED_EDGE ( 'NONE', *, *, #29868, .T. ) ;
#11485=ORIENTED_EDGE ( 'NONE', *, *, #60783, .T. ) ;
#11486=DIRECTION ( 'NONE',  ( -1.000000000000000000, 0.000000000000000000, 0.000000000000000000 ) ) ;
#11489=ADVANCED_FACE ( 'NONE', ( #92096 ), #85229, .F. ) ;
#11497=DIRECTION ( 'NONE',  ( 0.5729786897769424403, -5.686911123206802946E-15, -0.8195702660916258653 ) ) ;
#11502=CARTESIAN_POINT ( 'NONE',  ( 140.6539576904058606, 276.0000000000000568, -12.00000000000000178 ) ) ;
#11508=EDGE_CURVE ( 'NONE', #84479, #75355, #20146, .T. ) ;
#11514=DIRECTION ( 'NONE',  ( 0.2456588035076310295, -0.9693563597868428694, 0.000000000000000000 ) ) ;
#11518=DIRECTION ( 'NONE',  ( 0.4999999999999967248, 0.8660254037844404840, 0.000000000000000000 ) ) ;
#11520=ORIENTED_EDGE ( 'NONE', *, *, #65065, .T. ) ;
#11521=CARTESIAN_POINT ( 'NONE',  ( 158.6539576904058606, 293.9636489450775230, 0.000000000000000000 ) ) ;
#11523=DIRECTION ( 'NONE',  ( 0.000000000000000000, 0.000000000000000000, 1.000000000000000000 ) ) ;
#11535=ORIENTED_EDGE ( 'NONE', *, *, #36693, .F. ) ;
#11538=DIRECTION ( 'NONE',  ( 0.000000000000000000, 0.000000000000000000, 1.000000000000000000 ) ) ;
#11556=CARTESIAN_POINT ( 'NONE',  ( 180.7149167944524493, 8.542400036368780647, -9.000000000000001776 ) ) ;
#11569=ORIENTED_EDGE ( 'NONE', *, *, #27631, .F. ) ;
#11583=CIRCLE ( 'NONE', #55461, 0.5000000000000004441 ) ;
#11598=EDGE_CURVE ( 'NONE', #2535, #307, #76171, .T. ) ;
#11599=ORIENTED_EDGE ( 'NONE', *, *, #15267, .F. ) ;
#11607=CARTESIAN_POINT ( 'NONE',  ( 153.4245301327638344, 19.61868323046913432, -10.85241966621300591 ) ) ;
#11611=DIRECTION ( 'NONE',  ( 0.8348322475753292560, 0.5505044217881672752, -0.000000000000000000 ) ) ;
#11624=CARTESIAN_POINT ( 'NONE',  ( 196.0143093133015384, 73.40565171261611965, 12.00000000000000711 ) ) ;
#11638=DIRECTION ( 'NONE',  ( 1.000000000000000000, -0.000000000000000000, 0.000000000000000000 ) ) ;
#11647=DIRECTION ( 'NONE',  ( -0.000000000000000000, -1.000000000000000000, -0.000000000000000000 ) ) ;
#11662=EDGE_CURVE ( 'NONE', #4210, #49577, #1017, .T. ) ;
#11679=ORIENTED_EDGE ( 'NONE', *, *, #33815, .F. ) ;
#11689=FACE_OUTER_BOUND ( 'NONE', #19985, .T. ) ;
#11694=ORIENTED_EDGE ( 'NONE', *, *, #80334, .F. ) ;
#11703=ORIENTED_EDGE ( 'NONE', *, *, #42165, .F. ) ;
#11710=DIRECTION ( 'NONE',  ( 0.000000000000000000, 0.000000000000000000, 1.000000000000000000 ) ) ;
#11711=CARTESIAN_POINT ( 'NONE',  ( 199.2296996224750103, 68.12454877784578855, 2.107038703926640721 ) ) ;
#11719=CARTESIAN_POINT ( 'NONE',  ( 195.9136854370872811, 42.35701288050587721, 12.17428566605772922 ) ) ;
#11724=DIRECTION ( 'NONE',  ( -0.000000000000000000, -1.000000000000000000, -0.000000000000000000 ) ) ;
#11727=EDGE_CURVE ( 'NONE', #49577, #610, #40228, .T. ) ;
#11739=CARTESIAN_POINT ( 'NONE',  ( 209.2599468862078140, 293.9636489450776367, 3.999999999999991562 ) ) ;
#11740=DIRECTION ( 'NONE',  ( 0.000000000000000000, 1.000000000000000000, 0.000000000000000000 ) ) ;
#11754=DIRECTION ( 'NONE',  ( 0.000000000000000000, 0.000000000000000000, 1.000000000000000000 ) ) ;
#11763=CARTESIAN_POINT ( 'NONE',  ( 195.4093337208560399, 40.63452519861395729, 14.75905111207264220 ) ) ;
#11771=ORIENTED_EDGE ( 'NONE', *, *, #49238, .T. ) ;
#11772=CARTESIAN_POINT ( 'NONE',  ( 184.7149167944524493, 8.542400036368780647, -9.000000000000001776 ) ) ;
#11778=EDGE_CURVE ( 'NONE', #1585, #19733, #52981, .T. ) ;
#11779=EDGE_CURVE ( 'NONE', #24854, #25416, #65594, .T. ) ;
#11807=ORIENTED_EDGE ( 'NONE', *, *, #80555, .F. ) ;
#11817=VERTEX_POINT ( 'NONE', #87782 ) ;
#11819=CARTESIAN_POINT ( 'NONE',  ( 165.2688068684385883, 275.0000000000000568, 21.83530662808711398 ) ) ;
#11824=CARTESIAN_POINT ( 'NONE',  ( 197.4878715644970555, 25.93102243561467546, 11.99999999999999112 ) ) ;
#11834=ORIENTED_EDGE ( 'NONE', *, *, #67723, .F. ) ;
#11844=CARTESIAN_POINT ( 'NONE',  ( 219.8344101925596021, 0.000000000000000000, 9.000000000000001776 ) ) ;
#11852=EDGE_CURVE ( 'NONE', #49537, #37280, #91679, .T. ) ;
#11859=CARTESIAN_POINT ( 'NONE',  ( 198.5394373320682746, 68.65923120349998499, 9.381478303810135699 ) ) ;
#11861=FACE_OUTER_BOUND ( 'NONE', #15049, .T. ) ;
#11869=EDGE_CURVE ( 'NONE', #70, #69962, #18718, .T. ) ;
#11870=LINE ( 'NONE', #18501, #10854 ) ;
#11872=FACE_OUTER_BOUND ( 'NONE', #64731, .T. ) ;
#11874=CARTESIAN_POINT ( 'NONE',  ( 159.4851178187871312, 3.000000000000000000, -9.000000000000001776 ) ) ;
#11875=DIRECTION ( 'NONE',  ( 0.9531768234071978929, -0.3024135303179465439, -0.000000000000000000 ) ) ;
#11886=FACE_OUTER_BOUND ( 'NONE', #77346, .T. ) ;
#11889=LINE ( 'NONE', #33666, #51849 ) ;
#11892=EDGE_CURVE ( 'NONE', #56772, #70448, #23866, .T. ) ;
#11903=CARTESIAN_POINT ( 'NONE',  ( 153.1590225954906543, 19.71789692321348397, -10.20076944887112269 ) ) ;
#11919=ORIENTED_EDGE ( 'NONE', *, *, #62384, .F. ) ;
#11924=CARTESIAN_POINT ( 'NONE',  ( 195.4663476211042052, 20.04167166511072651, -14.69138476959436623 ) ) ;
#11929=ORIENTED_EDGE ( 'NONE', *, *, #46756, .F. ) ;
#11936=DIRECTION ( 'NONE',  ( 0.000000000000000000, 0.000000000000000000, 1.000000000000000000 ) ) ;
#11954=ORIENTED_EDGE ( 'NONE', *, *, #41498, .T. ) ;
#11956=VECTOR ( 'NONE', #88714, 1000.000000000000000 ) ;
#11962=LINE ( 'NONE', #19997, #14298 ) ;
#11967=CARTESIAN_POINT ( 'NONE',  ( 209.0355956570440412, 30.15830632019625313, 14.26380412825890787 ) ) ;
#11977=DIRECTION ( 'NONE',  ( 1.000000000000000000, 0.000000000000000000, 0.000000000000000000 ) ) ;
#11978=DIRECTION ( 'NONE',  ( -0.2456588035076248677, 0.9693563597868444237, 0.000000000000000000 ) ) ;
#11982=CARTESIAN_POINT ( 'NONE',  ( 140.6539576904058606, 275.0000000000000568, 12.50000000000000000 ) ) ;
#11987=CARTESIAN_POINT ( 'NONE',  ( 156.4947056272797852, 21.00000000000000000, 15.00000000000000000 ) ) ;
#11999=EDGE_CURVE ( 'NONE', #51424, #33982, #28195, .T. ) ;
#12004=CARTESIAN_POINT ( 'NONE',  ( 169.7306087885279453, 275.5000000000000568, -24.89999999999999147 ) ) ;
#12006=ORIENTED_EDGE ( 'NONE', *, *, #51325, .T. ) ;
#12008=CARTESIAN_POINT ( 'NONE',  ( 198.5113747970946179, 66.01554725018998226, 10.78125329330598348 ) ) ;
#12020=EDGE_CURVE ( 'NONE', #10127, #44168, #24728, .T. ) ;
#12022=AXIS2_PLACEMENT_3D ( 'NONE', #16185, #65944, #52612 ) ;
#12040=ORIENTED_EDGE ( 'NONE', *, *, #6789, .F. ) ;
#12059=EDGE_LOOP ( 'NONE', ( #52244, #91910 ) ) ;
#12067=EDGE_LOOP ( 'NONE', ( #24580, #17667, #8430, #49991 ) ) ;
#12074=DIRECTION ( 'NONE',  ( -0.9693563597868444237, -0.2456588035076248677, 0.000000000000000000 ) ) ;
#12079=FACE_OUTER_BOUND ( 'NONE', #536, .T. ) ;
#12084=AXIS2_PLACEMENT_3D ( 'NONE', #75709, #89904, #25513 ) ;
#12087=CARTESIAN_POINT ( 'NONE',  ( 153.3642062430809858, 20.33187285098938091, -12.12209853637909696 ) ) ;
#12097=CARTESIAN_POINT ( 'NONE',  ( 180.0056393205866812, 275.0000000000000568, -23.52000000000002800 ) ) ;
#12108=EDGE_CURVE ( 'NONE', #2466, #78327, #51341, .T. ) ;
#12116=CARTESIAN_POINT ( 'NONE',  ( 208.0457363859825932, 36.70443730966733398, 13.54762445178161556 ) ) ;
#12137=DIRECTION ( 'NONE',  ( 0.000000000000000000, 0.000000000000000000, -1.000000000000000000 ) ) ;
#12148=ORIENTED_EDGE ( 'NONE', *, *, #17507, .F. ) ;
#12161=AXIS2_PLACEMENT_3D ( 'NONE', #47973, #91532, #54614 ) ;
#12173=VERTEX_POINT ( 'NONE', #65456 ) ;
#12187=CARTESIAN_POINT ( 'NONE',  ( 160.5350683151633291, 250.0000000000000568, 20.22542485937379908 ) ) ;
#12189=CARTESIAN_POINT ( 'NONE',  ( 199.0061125298537377, 275.5000000000000568, -7.725424859374024678 ) ) ;
#12191=ORIENTED_EDGE ( 'NONE', *, *, #80971, .F. ) ;
#12193=LINE ( 'NONE', #62886, #47404 ) ;
#12195=EDGE_CURVE ( 'NONE', #52563, #1567, #45873, .T. ) ;
#12208=CARTESIAN_POINT ( 'NONE',  ( 193.2782779784440379, 275.9651295423822717, 16.89756555088499113 ) ) ;
#12209=CARTESIAN_POINT ( 'NONE',  ( 153.9133111279456045, 20.47222690886501439, -13.06183683676588991 ) ) ;
#12221=CARTESIAN_POINT ( 'NONE',  ( 175.2296996224750103, 249.5000000000000568, 0.000000000000000000 ) ) ;
#12223=DIRECTION ( 'NONE',  ( 0.000000000000000000, 1.000000000000000000, 0.000000000000000000 ) ) ;
#12228=CIRCLE ( 'NONE', #65192, 1.499999999999992673 ) ;
#12234=CARTESIAN_POINT ( 'NONE',  ( 195.4675039778850874, 40.79415162994154542, 14.67933883143855844 ) ) ;
#12242=ORIENTED_EDGE ( 'NONE', *, *, #46507, .F. ) ;
#12254=EDGE_CURVE ( 'NONE', #79037, #42785, #56532, .T. ) ;
#12256=EDGE_LOOP ( 'NONE', ( #34034, #70174, #3561, #19174 ) ) ;
#12257=DIRECTION ( 'NONE',  ( -0.000000000000000000, -1.000000000000000000, -0.000000000000000000 ) ) ;
#12265=ORIENTED_EDGE ( 'NONE', *, *, #53102, .F. ) ;
#12270=CARTESIAN_POINT ( 'NONE',  ( 196.8803347170859865, 250.0000000000000568, 12.49999999999999289 ) ) ;
#12271=CARTESIAN_POINT ( 'NONE',  ( 175.2296996224750103, 247.0000000000001137, 8.550761578869359170 ) ) ;
#12272=DIRECTION ( 'NONE',  ( 0.000000000000000000, 0.000000000000000000, 1.000000000000000000 ) ) ;
#12291=VERTEX_POINT ( 'NONE', #86254 ) ;
#12307=ORIENTED_EDGE ( 'NONE', *, *, #907, .F. ) ;
#12308=CARTESIAN_POINT ( 'NONE',  ( 206.8799559751410584, 30.07585723490866059, 15.00000000000000178 ) ) ;
#12329=DIRECTION ( 'NONE',  ( 0.000000000000000000, 0.000000000000000000, 1.000000000000000000 ) ) ;
#12331=DIRECTION ( 'NONE',  ( 1.000000000000000000, -0.000000000000000000, -0.000000000000000000 ) ) ;
#12341=CARTESIAN_POINT ( 'NONE',  ( 202.9270896288134907, 287.6726455163375249, -4.941865385500935126 ) ) ;
#12354=AXIS2_PLACEMENT_3D ( 'NONE', #82747, #48156, #48626 ) ;
#12362=AXIS2_PLACEMENT_3D ( 'NONE', #79885, #29710, #58592 ) ;
#12371=DIRECTION ( 'NONE',  ( 0.7484200282493165268, 0.000000000000000000, -0.6632250457539224930 ) ) ;
#12390=ORIENTED_EDGE ( 'NONE', *, *, #79580, .F. ) ;
#12406=CARTESIAN_POINT ( 'NONE',  ( 208.6208076322478746, 32.98517505407394168, 12.09245862095555601 ) ) ;
#12412=EDGE_LOOP ( 'NONE', ( #49233, #85830, #50103, #92985, #51621, #43910 ) ) ;
#12419=VERTEX_POINT ( 'NONE', #17103 ) ;
#12420=DIRECTION ( 'NONE',  ( -1.000000000000000000, 0.000000000000000000, 0.000000000000000000 ) ) ;
#12424=EDGE_LOOP ( 'NONE', ( #66019, #79941, #54756, #43116, #88073, #25649 ) ) ;
#12432=DIRECTION ( 'NONE',  ( 0.000000000000000000, 0.000000000000000000, -1.000000000000000000 ) ) ;
#12443=CIRCLE ( 'NONE', #35218, 9.103929867429224387 ) ;
#12451=CARTESIAN_POINT ( 'NONE',  ( 208.4306832106270519, 1.063508326895939771, 7.500000000000014211 ) ) ;
#12452=CARTESIAN_POINT ( 'NONE',  ( 197.2116943569230330, 276.0000000000000568, -12.92446933126074882 ) ) ;
#12457=DIRECTION ( 'NONE',  ( 0.000000000000000000, 1.000000000000000000, 0.000000000000000000 ) ) ;
#12460=CARTESIAN_POINT ( 'NONE',  ( 156.1243321211817374, 16.88031981476169108, -7.577257116167564810 ) ) ;
#12462=DIRECTION ( 'NONE',  ( -0.000000000000000000, 0.000000000000000000, 1.000000000000000000 ) ) ;
#12465=CARTESIAN_POINT ( 'NONE',  ( 153.9079962421555763, 20.48904911123736028, -11.76949543550875354 ) ) ;
#12478=DIRECTION ( 'NONE',  ( 1.000000000000000000, 0.000000000000000000, 0.000000000000000000 ) ) ;
#12480=VERTEX_POINT ( 'NONE', #23739 ) ;
#12482=FACE_OUTER_BOUND ( 'NONE', #51875, .T. ) ;
#12496=CARTESIAN_POINT ( 'NONE',  ( 160.5350683151633291, 275.0000000000000568, 7.500000000000000000 ) ) ;
#12497=CIRCLE ( 'NONE', #42763, 0.4999999999999938938 ) ;
#12510=CIRCLE ( 'NONE', #41187, 1.000000000000000888 ) ;
#12518=EDGE_LOOP ( 'NONE', ( #63470, #92519, #40437, #82367, #32218 ) ) ;
#12534=EDGE_LOOP ( 'NONE', ( #25226, #90067, #51275, #74225 ) ) ;
#12541=ORIENTED_EDGE ( 'NONE', *, *, #17686, .T. ) ;
#12543=VERTEX_POINT ( 'NONE', #52150 ) ;
#12551=CARTESIAN_POINT ( 'NONE',  ( 185.0172044724083946, 275.5000000000000568, 22.46007009812148425 ) ) ;
#12565=DIRECTION ( 'NONE',  ( 0.9693563597868444237, 0.2456588035076248677, 0.000000000000000000 ) ) ;
#12566=VECTOR ( 'NONE', #35159, 1000.000000000000000 ) ;
#12568=B_SPLINE_CURVE_WITH_KNOTS ( 'NONE', 3,
 ( #87513, #44438, #80422, #15567, #73344, #8455, #37336, #66242, #76598, #69487, #54801, #3698 ),
 .UNSPECIFIED., .F., .F.,
 ( 4, 2, 2, 2, 2, 4 ),
 ( 1.734723475976806902E-18, 0.002272214944544886147, 0.004544429889089770559, 0.006816644833634654538, 0.007952752305907110839, 0.009088859778179567139 ),
 .UNSPECIFIED. ) ;
#12573=AXIS2_PLACEMENT_3D ( 'NONE', #24059, #31186, #52473 ) ;
#12576=CIRCLE ( 'NONE', #36759, 24.50000000000000355 ) ;
#12579=CARTESIAN_POINT ( 'NONE',  ( 207.6175730408114930, 30.32598770090644180, 14.41714557868295898 ) ) ;
#12587=AXIS2_PLACEMENT_3D ( 'NONE', #82070, #90103, #90549 ) ;
#12600=CARTESIAN_POINT ( 'NONE',  ( 186.2362647323748206, 275.5000000000000568, 22.80382896336986320 ) ) ;
#12618=CARTESIAN_POINT ( 'NONE',  ( 156.9594811538147781, 18.65395765032316788, 11.57852291560509883 ) ) ;
#12627=EDGE_CURVE ( 'NONE', #76858, #24854, #75925, .T. ) ;
#12630=VERTEX_POINT ( 'NONE', #45485 ) ;
#12640=CIRCLE ( 'NONE', #65589, 4.999999999999990230 ) ;
#12644=CARTESIAN_POINT ( 'NONE',  ( 154.7381521964306330, 128.4861308677204761, -12.50226176571347381 ) ) ;
#12659=ORIENTED_EDGE ( 'NONE', *, *, #63702, .F. ) ;
#12664=EDGE_CURVE ( 'NONE', #85724, #23580, #67046, .T. ) ;
#12667=SPHERICAL_SURFACE ( 'NONE', #59724, 3.000000000000000000 ) ;
#12670=CARTESIAN_POINT ( 'NONE',  ( 157.7670607448531541, 18.75975317436490286, 10.28854280544483402 ) ) ;
#12677=DIRECTION ( 'NONE',  ( -0.000000000000000000, -0.000000000000000000, 1.000000000000000000 ) ) ;
#12679=FACE_OUTER_BOUND ( 'NONE', #88112, .T. ) ;
#12681=ORIENTED_EDGE ( 'NONE', *, *, #81096, .F. ) ;
#12682=ORIENTED_EDGE ( 'NONE', *, *, #44981, .F. ) ;
#12683=DIRECTION ( 'NONE',  ( 0.9693563597868433135, 0.2456588035076293641, 0.000000000000000000 ) ) ;
#12696=AXIS2_PLACEMENT_3D ( 'NONE', #50032, #84451, #56067 ) ;
#12699=CARTESIAN_POINT ( 'NONE',  ( 199.5070675535761495, 288.7003404203971400, -6.034989766317571558 ) ) ;
#12700=DIRECTION ( 'NONE',  ( 0.000000000000000000, -0.000000000000000000, 1.000000000000000000 ) ) ;
#12718=AXIS2_PLACEMENT_3D ( 'NONE', #17331, #4052, #91117 ) ;
#12726=DIRECTION ( 'NONE',  ( -0.000000000000000000, -1.000000000000000000, -0.000000000000000000 ) ) ;
#12731=AXIS2_PLACEMENT_3D ( 'NONE', #60106, #75231, #52048 ) ;
#12735=ORIENTED_EDGE ( 'NONE', *, *, #61465, .T. ) ;
#12736=LINE ( 'NONE', #78986, #59005 ) ;
#12750=EDGE_LOOP ( 'NONE', ( #90163, #51490, #34785, #16257 ) ) ;
#12751=CARTESIAN_POINT ( 'NONE',  ( 194.7541945649814181, 39.97853125882125624, 13.97297966198307506 ) ) ;
#12754=CARTESIAN_POINT ( 'NONE',  ( 200.1063562618922447, 64.94916223748940354, -5.267193185415704804 ) ) ;
#12755=EDGE_CURVE ( 'NONE', #31130, #21613, #7616, .T. ) ;
#12757=VERTEX_POINT ( 'NONE', #89504 ) ;
#12763=DIRECTION ( 'NONE',  ( 0.000000000000000000, 1.000000000000000000, 0.000000000000000000 ) ) ;
#12764=CARTESIAN_POINT ( 'NONE',  ( 175.2296996224750103, 276.0000000000000568, 24.50000000000000355 ) ) ;
#12767=ORIENTED_EDGE ( 'NONE', *, *, #11727, .T. ) ;
#12784=EDGE_CURVE ( 'NONE', #7661, #1451, #82169, .T. ) ;
#12786=ORIENTED_EDGE ( 'NONE', *, *, #57360, .F. ) ;
#12787=AXIS2_PLACEMENT_3D ( 'NONE', #11028, #90097, #10100 ) ;
#12788=CARTESIAN_POINT ( 'NONE',  ( 139.6539576904058606, 275.0000000000000568, -10.49999999999999822 ) ) ;
#12802=ORIENTED_EDGE ( 'NONE', *, *, #68670, .T. ) ;
#12804=CARTESIAN_POINT ( 'NONE',  ( 159.4851178187871312, 15.00000000000000000, -10.00000000000000000 ) ) ;
#12807=AXIS2_PLACEMENT_3D ( 'NONE', #61227, #25668, #2969 ) ;
#12814=CARTESIAN_POINT ( 'NONE',  ( 154.1407330040854333, 250.5000000000000568, -13.42592592592594158 ) ) ;
#12820=CARTESIAN_POINT ( 'NONE',  ( 199.0061125298537377, 215.0000000000000568, -7.725424859374024678 ) ) ;
#12822=AXIS2_PLACEMENT_3D ( 'NONE', #68164, #3284, #53949 ) ;
#12828=EDGE_CURVE ( 'NONE', #62353, #11375, #20287, .T. ) ;
#12831=FACE_OUTER_BOUND ( 'NONE', #38015, .T. ) ;
#12840=DIRECTION ( 'NONE',  ( -0.000000000000000000, -0.000000000000000000, -1.000000000000000000 ) ) ;
#12842=DIRECTION ( 'NONE',  ( 0.000000000000000000, 0.000000000000000000, 1.000000000000000000 ) ) ;
#12854=CARTESIAN_POINT ( 'NONE',  ( 180.7287904564219332, 275.0000000000000568, -24.90000000000003411 ) ) ;
#12868=CIRCLE ( 'NONE', #34010, 0.4999999999999985567 ) ;
#12869=EDGE_CURVE ( 'NONE', #63051, #82273, #55004, .T. ) ;
#12870=CARTESIAN_POINT ( 'NONE',  ( 160.5350683151633291, 250.0000000000000568, 20.22542485937379908 ) ) ;
#12882=AXIS2_PLACEMENT_3D ( 'NONE', #24997, #53869, #64289 ) ;
#12887=ORIENTED_EDGE ( 'NONE', *, *, #85032, .T. ) ;
#12915=ORIENTED_EDGE ( 'NONE', *, *, #92, .T. ) ;
#12916=LINE ( 'NONE', #34670, #44242 ) ;
#12926=LINE ( 'NONE', #63595, #29365 ) ;
#12928=B_SPLINE_CURVE_WITH_KNOTS ( 'NONE', 3,
 ( #81962, #10926, #16644, #31788, #2456, #67324 ),
 .UNSPECIFIED., .F., .F.,
 ( 4, 2, 4 ),
 ( -4.472146915492242146E-06, 0.0004206930844425495024, 0.0008458583158005913028 ),
 .UNSPECIFIED. ) ;
#12933=DIRECTION ( 'NONE',  ( 0.000000000000000000, 0.000000000000000000, -1.000000000000000000 ) ) ;
#12946=PLANE ( 'NONE',  #14081 ) ;
#12954=CARTESIAN_POINT ( 'NONE',  ( 209.4353741342548005, 38.08050248846151220, 13.99694255477028015 ) ) ;
#12956=FACE_OUTER_BOUND ( 'NONE', #43600, .T. ) ;
#12968=ORIENTED_EDGE ( 'NONE', *, *, #50836, .T. ) ;
#12971=DIRECTION ( 'NONE',  ( -0.9693563597868444237, -0.2456588035076248677, -0.000000000000000000 ) ) ;
#12989=DIRECTION ( 'NONE',  ( -0.000000000000000000, -1.000000000000000000, -0.000000000000000000 ) ) ;
#12998=CARTESIAN_POINT ( 'NONE',  ( 157.4851178187871312, 1.000000000000001332, 7.000000000000000000 ) ) ;
#13000=EDGE_CURVE ( 'NONE', #13010, #67402, #11210, .T. ) ;
#13007=ORIENTED_EDGE ( 'NONE', *, *, #56360, .T. ) ;
#13010=VERTEX_POINT ( 'NONE', #18035 ) ;
#13027=EDGE_LOOP ( 'NONE', ( #34980, #88322 ) ) ;
#13034=ORIENTED_EDGE ( 'NONE', *, *, #47255, .T. ) ;
#13042=DIRECTION ( 'NONE',  ( -0.000000000000000000, -1.000000000000000000, -0.000000000000000000 ) ) ;
#13052=ADVANCED_FACE ( 'NONE', ( #4756 ), #85609, .F. ) ;
#13055=DIRECTION ( 'NONE',  ( 0.000000000000000000, 1.000000000000000000, 0.000000000000000000 ) ) ;
#13063=CARTESIAN_POINT ( 'NONE',  ( 198.6884013828325521, 64.61450673763174279, -9.555809373750800972 ) ) ;
#13067=DIRECTION ( 'NONE',  ( -0.000000000000000000, -0.000000000000000000, 1.000000000000000000 ) ) ;
#13080=DIRECTION ( 'NONE',  ( 1.000000000000000000, -0.000000000000000000, 0.000000000000000000 ) ) ;
#13083=CARTESIAN_POINT ( 'NONE',  ( 202.4316997032785537, 63.54496854667812755, 6.999999999999996447 ) ) ;
#13100=CARTESIAN_POINT ( 'NONE',  ( 196.7647826491495096, 294.9769576964061457, -7.939513337131741011 ) ) ;
#13104=ADVANCED_FACE ( 'NONE', ( #5712 ), #69163, .T. ) ;
#13111=VERTEX_POINT ( 'NONE', #68703 ) ;
#13112=ORIENTED_EDGE ( 'NONE', *, *, #34764, .F. ) ;
#13123=CYLINDRICAL_SURFACE ( 'NONE', #26653, 9.103929867429224387 ) ;
#13136=ORIENTED_EDGE ( 'NONE', *, *, #66277, .T. ) ;
#13140=ORIENTED_EDGE ( 'NONE', *, *, #60551, .T. ) ;
#13141=DIRECTION ( 'NONE',  ( -0.000000000000000000, -1.000000000000000000, -0.000000000000000000 ) ) ;
#13143=DIRECTION ( 'NONE',  ( 0.000000000000000000, 1.000000000000000000, 0.000000000000000000 ) ) ;
#13149=CARTESIAN_POINT ( 'NONE',  ( 154.7659666677267865, 20.47222690886501439, 12.53936336329526391 ) ) ;
#13152=ORIENTED_EDGE ( 'NONE', *, *, #26870, .F. ) ;
#13153=VERTEX_POINT ( 'NONE', #3833 ) ;
#13154=DIRECTION ( 'NONE',  ( 0.000000000000000000, 0.000000000000000000, 1.000000000000000000 ) ) ;
#13171=( BOUNDED_CURVE ( )  B_SPLINE_CURVE ( 3, ( #45369, #1844, #31660, #81833 ),
 .UNSPECIFIED., .F., .F. ) 
 B_SPLINE_CURVE_WITH_KNOTS ( ( 4, 4 ),
 ( 3.665191429188093597, 4.712388980384689674 ),
 .UNSPECIFIED. ) 
 CURVE ( )  GEOMETRIC_REPRESENTATION_ITEM ( )  RATIONAL_B_SPLINE_CURVE ( ( 1.000000000000000000, 0.9106836025229593234, 0.9106836025229593234, 1.000000000000000000 ) ) 
 REPRESENTATION_ITEM ( '' )  );
#13181=( BOUNDED_SURFACE ( )  B_SPLINE_SURFACE ( 3, 2, ( 
 ( #35975, #51102, #92317 ),
 ( #6169, #71986, #6642 ),
 ( #85227, #58239, #7104 ),
 ( #86149, #71509, #27471 ),
 ( #14682, #21300, #50172 ),
 ( #78602, #20508, #28876 ) ),
 .UNSPECIFIED., .F., .F., .F. ) 
 B_SPLINE_SURFACE_WITH_KNOTS ( ( 4, 2, 4 ),
 ( 3, 3 ),
 ( 5.756444938927698374, 6.019815123053642303, 6.283185307179586232 ),
 ( 0.000000000000000000, 1.000000000000000000 ),
 .UNSPECIFIED. ) 
 GEOMETRIC_REPRESENTATION_ITEM ( )  RATIONAL_B_SPLINE_SURFACE ( (
 ( 1.000000000000000000, 0.9186651033962678348, 1.000000000000000000),
 ( 1.000000000000000000, 0.9282241625911032967, 1.000000000000000000),
 ( 1.000000000000000000, 0.9354614375524443748, 1.000000000000000000),
 ( 1.000000000000000000, 0.9451322790882570324, 1.000000000000000000),
 ( 1.000000000000000000, 0.9475641245298920268, 1.000000000000000000),
 ( 1.000000000000000000, 0.9475641245298920268, 1.000000000000000000) ) ) 
 REPRESENTATION_ITEM ( '' )  SURFACE ( )  );
#13184=DIRECTION ( 'NONE',  ( 1.000000000000000000, -0.000000000000000000, 0.000000000000000000 ) ) ;
#13186=DIRECTION ( 'NONE',  ( -0.2456588035076305854, 0.9693563597868429804, 0.000000000000000000 ) ) ;
#13198=CARTESIAN_POINT ( 'NONE',  ( 195.9379236003509845, 41.56271157415176987, 14.00773366423596045 ) ) ;
#13204=ADVANCED_FACE ( 'NONE', ( #32715 ), #70168, .F. ) ;
#13207=ORIENTED_EDGE ( 'NONE', *, *, #80212, .F. ) ;
#13208=CARTESIAN_POINT ( 'NONE',  ( 152.9200301536615427, 20.54241773159251494, 11.30461213544953480 ) ) ;
#13210=CARTESIAN_POINT ( 'NONE',  ( 208.1134247887914057, 29.32324166632049156, 13.52119360038336460 ) ) ;
#13220=ORIENTED_EDGE ( 'NONE', *, *, #4023, .F. ) ;
#13221=CARTESIAN_POINT ( 'NONE',  ( 195.6548686469884331, 40.46313866827317440, 13.67209655823288550 ) ) ;
#13225=ADVANCED_FACE ( 'NONE', ( #56859 ), #58251, .F. ) ;
#13227=VERTEX_POINT ( 'NONE', #7562 ) ;
#13233=CARTESIAN_POINT ( 'NONE',  ( 175.2296996224750103, 161.0000000000000853, -9.550761578869391144 ) ) ;
#13242=ORIENTED_EDGE ( 'NONE', *, *, #45431, .F. ) ;
#13267=ORIENTED_EDGE ( 'NONE', *, *, #18976, .F. ) ;
#13268=DIRECTION ( 'NONE',  ( -0.000000000000000000, -1.000000000000000000, -0.000000000000000000 ) ) ;
#13283=DIRECTION ( 'NONE',  ( 0.000000000000000000, -0.000000000000000000, 1.000000000000000000 ) ) ;
#13315=DIRECTION ( 'NONE',  ( -0.000000000000000000, 1.000000000000000000, -0.000000000000000000 ) ) ;
#13317=DIRECTION ( 'NONE',  ( -0.000000000000000000, -0.000000000000000000, 1.000000000000000000 ) ) ;
#13329=DIRECTION ( 'NONE',  ( 0.000000000000000000, 0.000000000000000000, 1.000000000000000000 ) ) ;
#13330=EDGE_CURVE ( 'NONE', #72522, #69300, #80001, .T. ) ;
#13344=ORIENTED_EDGE ( 'NONE', *, *, #32210, .F. ) ;
#13346=VERTEX_POINT ( 'NONE', #79080 ) ;
#13350=( NAMED_UNIT ( * ) PLANE_ANGLE_UNIT ( ) SI_UNIT ( $, .RADIAN. ) );
#13355=ORIENTED_EDGE ( 'NONE', *, *, #8701, .T. ) ;
#13362=FACE_OUTER_BOUND ( 'NONE', #92185, .T. ) ;
#13368=VERTEX_POINT ( 'NONE', #28886 ) ;
#13375=EDGE_LOOP ( 'NONE', ( #39374, #53160, #70901, #40643, #54433, #65990 ) ) ;
#13400=ADVANCED_FACE ( 'NONE', ( #93273 ), #78612, .F. ) ;
#13404=AXIS2_PLACEMENT_3D ( 'NONE', #51337, #29113, #14463 ) ;
#13405=CARTESIAN_POINT ( 'NONE',  ( 153.6987871352711181, 19.48326534539918597, 11.45812909362558152 ) ) ;
#13411=CARTESIAN_POINT ( 'NONE',  ( 193.6287972472565286, 250.3431421874260252, 16.89650703080491922 ) ) ;
#13414=DIRECTION ( 'NONE',  ( 0.000000000000000000, 0.000000000000000000, 1.000000000000000000 ) ) ;
#13417=CARTESIAN_POINT ( 'NONE',  ( 195.4781563537916043, 39.36132622696000283, 15.50000000000000000 ) ) ;
#13427=ORIENTED_EDGE ( 'NONE', *, *, #78743, .F. ) ;
#13430=CARTESIAN_POINT ( 'NONE',  ( 175.2296996224750103, 133.0000000000000000, 24.00000000000001066 ) ) ;
#13456=CARTESIAN_POINT ( 'NONE',  ( 201.2104617360081704, 60.19600395700749829, -10.00000000000000000 ) ) ;
#13464=EDGE_LOOP ( 'NONE', ( #34100, #37556, #53503 ) ) ;
#13467=EDGE_LOOP ( 'NONE', ( #74735, #90252, #1413, #93246 ) ) ;
#13492=ORIENTED_EDGE ( 'NONE', *, *, #4124, .F. ) ;
#13494=ORIENTED_EDGE ( 'NONE', *, *, #2808, .T. ) ;
#13501=DIRECTION ( 'NONE',  ( 1.000000000000000000, 0.000000000000000000, 0.000000000000000000 ) ) ;
#13512=DIRECTION ( 'NONE',  ( -1.224646799147353207E-16, 1.000000000000000000, 0.000000000000000000 ) ) ;
#13517=EDGE_CURVE ( 'NONE', #62986, #27803, #82242, .T. ) ;
#13521=DIRECTION ( 'NONE',  ( 1.000000000000000000, 0.000000000000000000, 0.000000000000000000 ) ) ;
#13525=DIRECTION ( 'NONE',  ( -0.000000000000000000, 1.000000000000000000, -0.000000000000000000 ) ) ;
#13537=DIRECTION ( 'NONE',  ( 1.000000000000000000, 0.000000000000000000, 0.000000000000000000 ) ) ;
#13538=CARTESIAN_POINT ( 'NONE',  ( 196.7806748523260012, 249.5000000000000568, -12.67104836398113576 ) ) ;
#13541=DIRECTION ( 'NONE',  ( 1.000000000000000000, 0.000000000000000000, 1.224646799147353207E-16 ) ) ;
#13567=ORIENTED_EDGE ( 'NONE', *, *, #14703, .T. ) ;
#13568=VERTEX_POINT ( 'NONE', #51115 ) ;
#13578=PLANE ( 'NONE',  #58088 ) ;
#13591=ORIENTED_EDGE ( 'NONE', *, *, #57795, .F. ) ;
#13595=VERTEX_POINT ( 'NONE', #6179 ) ;
#13597=CARTESIAN_POINT ( 'NONE',  ( 204.6539576904058606, 293.9636489450775230, -7.999911143031724237 ) ) ;
#13598=TOROIDAL_SURFACE ( 'NONE', #52898, 4.500000000000002665, 0.5000000000000000000 ) ;
#13601=VECTOR ( 'NONE', #61721, 1000.000000000000000 ) ;
#13605=CARTESIAN_POINT ( 'NONE',  ( 208.3297354249494902, 27.64700571354669734, 12.00000001296664820 ) ) ;
#13608=CARTESIAN_POINT ( 'NONE',  ( 175.2296996224750103, 138.1603916158177583, -24.00000000000001421 ) ) ;
#13609=VERTEX_POINT ( 'NONE', #63962 ) ;
#13626=ADVANCED_FACE ( 'NONE', ( #35533 ), #3647, .T. ) ;
#13642=CARTESIAN_POINT ( 'NONE',  ( 196.0143093133015384, 250.0000000000000568, 11.99999999999998757 ) ) ;
#13655=CARTESIAN_POINT ( 'NONE',  ( 195.7610338615059220, 41.66501297569730156, 14.26493301926425339 ) ) ;
#13665=VERTEX_POINT ( 'NONE', #92803 ) ;
#13666=CARTESIAN_POINT ( 'NONE',  ( 151.9826577741488904, 20.03748314400953134, 9.225496140117414257 ) ) ;
#13669=AXIS2_PLACEMENT_3D ( 'NONE', #92817, #29371, #43103 ) ;
#13678=ORIENTED_EDGE ( 'NONE', *, *, #65011, .F. ) ;
#13679=CARTESIAN_POINT ( 'NONE',  ( 194.3488207764574156, 40.17711433623663453, 14.50727004101163864 ) ) ;
#13689=CYLINDRICAL_SURFACE ( 'NONE', #29444, 4.999999999999990230 ) ;
#13691=DIRECTION ( 'NONE',  ( 0.2916739763039743472, 0.000000000000000000, 0.9565177946839404921 ) ) ;
#13694=ORIENTED_EDGE ( 'NONE', *, *, #1952, .T. ) ;
#13700=ORIENTED_EDGE ( 'NONE', *, *, #60977, .F. ) ;
#13709=ORIENTED_EDGE ( 'NONE', *, *, #1671, .T. ) ;
#13721=( BOUNDED_SURFACE ( )  B_SPLINE_SURFACE ( 3, 2, ( 
 ( #29592, #88250, #87776 ),
 ( #58471, #44699, #52274 ),
 ( #59872, #81153, #23860 ),
 ( #52726, #67436, #44226 ),
 ( #24320, #30045, #2563 ),
 ( #31442, #53197, #73136 ),
 ( #82075, #67891, #8261 ),
 ( #37142, #26670, #55560 ),
 ( #75454, #47012, #77327 ),
 ( #39437, #32833, #12460 ),
 ( #41307, #83951, #18624 ),
 ( #40368, #54138, #82553 ),
 ( #61723, #60792, #69285 ),
 ( #76859, #4414, #25713 ),
 ( #89630, #10574, #3959 ),
 ( #47490, #68353, #18159 ) ),
 .UNSPECIFIED., .F., .F., .T. ) 
 B_SPLINE_SURFACE_WITH_KNOTS ( ( 4, 2, 2, 2, 2, 2, 2, 4 ),
 ( 3, 3 ),
 ( 1.986477369973030482, 2.275256190877221307, 2.419645601329316609, 2.564035011781411910, 2.708424422233507212, 2.852813832685602513, 2.997203243137697815, 3.141592653589793116 ),
 ( 0.000000000000000000, 1.000000000000000000 ),
 .UNSPECIFIED. ) 
 GEOMETRIC_REPRESENTATION_ITEM ( )  RATIONAL_B_SPLINE_SURFACE ( (
 ( 1.000000000000000000, 0.9583671019093122911, 1.000000000000000000),
 ( 1.000000000000000000, 0.9398658125636130123, 1.000000000000000000),
 ( 1.000000000000000000, 0.9157002655848520689, 1.000000000000000000),
 ( 1.000000000000000000, 0.8756259400452285346, 1.000000000000000000),
 ( 1.000000000000000000, 0.8616433317033627137, 1.000000000000000000),
 ( 1.000000000000000000, 0.8334785261035606574, 1.000000000000000000),
 ( 1.000000000000000000, 0.8192978668689707700, 1.000000000000000000),
 ( 1.000000000000000000, 0.7919708659745015034, 1.000000000000000000),
 ( 1.000000000000000000, 0.7788285231916702855, 1.000000000000000000),
 ( 1.000000000000000000, 0.7549177526733148458, 1.000000000000000000),
 ( 1.000000000000000000, 0.7441566529437350086, 1.000000000000000000),
 ( 1.000000000000000000, 0.7262859251464029997, 1.000000000000000000),
 ( 1.000000000000000000, 0.7191857644035757335, 1.000000000000000000),
 ( 1.000000000000000000, 0.7095926089624606803, 1.000000000000000000),
 ( 1.000000000000000000, 0.7070960980132692253, 1.000000000000000000),
 ( 1.000000000000000000, 0.7071067811865473507, 1.000000000000000000) ) ) 
 REPRESENTATION_ITEM ( '' )  SURFACE ( )  );
#13726=VERTEX_POINT ( 'NONE', #49717 ) ;
#13727=CARTESIAN_POINT ( 'NONE',  ( 195.7261261297331885, 19.57027967189588935, -12.91595659652283423 ) ) ;
#13729=( BOUNDED_CURVE ( )  B_SPLINE_CURVE ( 3, ( #52139, #67754, #61136, #68218 ),
 .UNSPECIFIED., .F., .F. ) 
 B_SPLINE_CURVE_WITH_KNOTS ( ( 4, 4 ),
 ( 0.7297276562269648936, 1.570796326794896558 ),
 .UNSPECIFIED. ) 
 CURVE ( )  GEOMETRIC_REPRESENTATION_ITEM ( )  RATIONAL_B_SPLINE_CURVE ( ( 1.000000000000000000, 0.9419139527835176384, 0.9419139527835176384, 1.000000000000000000 ) ) 
 REPRESENTATION_ITEM ( '' )  );
#13732=EDGE_CURVE ( 'NONE', #74948, #9812, #77728, .T. ) ;
#13734=TOROIDAL_SURFACE ( 'NONE', #66636, 2.500000000000007994, 0.5000000000000000000 ) ;
#13757=DIRECTION ( 'NONE',  ( 0.000000000000000000, 1.000000000000000000, 0.000000000000000000 ) ) ;
#13769=CARTESIAN_POINT ( 'NONE',  ( 197.8754097859456635, 68.08024695722009767, -11.26651182472395085 ) ) ;
#13779=EDGE_LOOP ( 'NONE', ( #53532, #17751, #83525, #68431 ) ) ;
#13782=CARTESIAN_POINT ( 'NONE',  ( 189.9243309297870610, 250.0000000000000568, 15.22542485937351664 ) ) ;
#13795=DIRECTION ( 'NONE',  ( -0.000000000000000000, -1.000000000000000000, -0.000000000000000000 ) ) ;
#13798=CIRCLE ( 'NONE', #66712, 7.910944475430059519 ) ;
#13808=ORIENTED_EDGE ( 'NONE', *, *, #54472, .F. ) ;
#13823=DIRECTION ( 'NONE',  ( -0.000000000000000000, 1.000000000000000000, -0.000000000000000000 ) ) ;
#13829=VERTEX_POINT ( 'NONE', #36919 ) ;
#13837=CARTESIAN_POINT ( 'NONE',  ( 195.2230643128901022, 25.81418032658909567, 13.28579478226901678 ) ) ;
#13841=ADVANCED_FACE ( 'NONE', ( #17475 ), #9647, .T. ) ;
#13861=EDGE_CURVE ( 'NONE', #6353, #34447, #10343, .T. ) ;
#13864=CARTESIAN_POINT ( 'NONE',  ( 154.7659666677267580, 19.56018909072084355, 12.94946946941271193 ) ) ;
#13877=CARTESIAN_POINT ( 'NONE',  ( 196.4665495134686353, 24.53799251391352954, 13.19633711769627382 ) ) ;
#13878=FACE_OUTER_BOUND ( 'NONE', #24335, .T. ) ;
#13888=ORIENTED_EDGE ( 'NONE', *, *, #77208, .F. ) ;
#13893=ORIENTED_EDGE ( 'NONE', *, *, #76503, .F. ) ;
#13903=ORIENTED_EDGE ( 'NONE', *, *, #36821, .F. ) ;
#13909=CARTESIAN_POINT ( 'NONE',  ( 156.4851178187871312, 0.000000000000000000, 10.00000000000000000 ) ) ;
#13924=VERTEX_POINT ( 'NONE', #8943 ) ;
#13930=EDGE_CURVE ( 'NONE', #74899, #42552, #73209, .T. ) ;
#13936=AXIS2_PLACEMENT_3D ( 'NONE', #5100, #46753, #75654 ) ;
#13948=ORIENTED_EDGE ( 'NONE', *, *, #55276, .T. ) ;
#13950=AXIS2_PLACEMENT_3D ( 'NONE', #53569, #17592, #46442 ) ;
#13957=EDGE_LOOP ( 'NONE', ( #26923, #89803, #1303, #27076 ) ) ;
#13958=EDGE_CURVE ( 'NONE', #46065, #29052, #74684, .T. ) ;
#13966=CARTESIAN_POINT ( 'NONE',  ( 200.7568414405312467, 39.78480925505071752, 10.50000000000000000 ) ) ;
#13973=EDGE_CURVE ( 'NONE', #65891, #35945, #89799, .T. ) ;
#13978=DIRECTION ( 'NONE',  ( 0.8435586647355767242, 0.000000000000000000, -0.5370370370370473045 ) ) ;
#13985=DIRECTION ( 'NONE',  ( 0.000000000000000000, 0.000000000000000000, 1.000000000000000000 ) ) ;
#13989=DIRECTION ( 'NONE',  ( 0.000000000000000000, 0.000000000000000000, 1.000000000000000000 ) ) ;
#14004=CARTESIAN_POINT ( 'NONE',  ( 209.5276096738287777, 37.00211571918214304, 12.90116063919866995 ) ) ;
#14009=AXIS2_PLACEMENT_3D ( 'NONE', #83090, #24404, #81232 ) ;
#14033=ORIENTED_EDGE ( 'NONE', *, *, #22733, .F. ) ;
#14043=DIRECTION ( 'NONE',  ( 0.000000000000000000, -0.000000000000000000, 1.000000000000000000 ) ) ;
#14044=CARTESIAN_POINT ( 'NONE',  ( 154.7659666677267580, 20.47222690886501439, -12.53936336329525858 ) ) ;
#14048=ORIENTED_EDGE ( 'NONE', *, *, #22221, .T. ) ;
#14060=ORIENTED_EDGE ( 'NONE', *, *, #65309, .F. ) ;
#14061=LINE ( 'NONE', #34435, #20515 ) ;
#14062=LINE ( 'NONE', #13597, #27962 ) ;
#14063=AXIS2_PLACEMENT_3D ( 'NONE', #92083, #70802, #20130 ) ;
#14064=CARTESIAN_POINT ( 'NONE',  ( 154.9307753191124846, 19.94580804509840277, 10.40578999957047479 ) ) ;
#14065=AXIS2_PLACEMENT_3D ( 'NONE', #61468, #82283, #60994 ) ;
#14071=VECTOR ( 'NONE', #11875, 1000.000000000000114 ) ;
#14072=DIRECTION ( 'NONE',  ( 0.000000000000000000, -0.000000000000000000, 1.000000000000000000 ) ) ;
#14073=DIRECTION ( 'NONE',  ( -0.000000000000000000, -0.000000000000000000, -1.000000000000000000 ) ) ;
#14074=VECTOR ( 'NONE', #31465, 1000.000000000000000 ) ;
#14076=DIRECTION ( 'NONE',  ( -0.000000000000000000, -1.000000000000000000, -0.000000000000000000 ) ) ;
#14081=AXIS2_PLACEMENT_3D ( 'NONE', #56497, #62182, #83462 ) ;
#14092=AXIS2_PLACEMENT_3D ( 'NONE', #60454, #30626, #67554 ) ;
#14095=CARTESIAN_POINT ( 'NONE',  ( 198.3066790443433263, 289.7462787566917655, -6.801086121950744356 ) ) ;
#14098=AXIS2_PLACEMENT_3D ( 'NONE', #54040, #26089, #47388 ) ;
#14110=EDGE_CURVE ( 'NONE', #26503, #90054, #8170, .T. ) ;
#14111=CARTESIAN_POINT ( 'NONE',  ( 184.7149167944524493, 8.542400036368780647, 10.00000000000000000 ) ) ;
#14120=CARTESIAN_POINT ( 'NONE',  ( 152.4536156746142410, 275.0000000000000568, 12.49999999999999289 ) ) ;
#14123=DIRECTION ( 'NONE',  ( 0.000000000000000000, 0.000000000000000000, 1.000000000000000000 ) ) ;
#14127=CARTESIAN_POINT ( 'NONE',  ( 151.9300335927204912, 130.8340072618044303, -11.50000000000000178 ) ) ;
#14133=CIRCLE ( 'NONE', #50404, 4.999999999999990230 ) ;
#14139=EDGE_LOOP ( 'NONE', ( #77161, #78539, #70260, #22433, #72188 ) ) ;
#14141=AXIS2_PLACEMENT_3D ( 'NONE', #90872, #5228, #33148 ) ;
#14143=DIRECTION ( 'NONE',  ( 0.000000000000000000, 0.000000000000000000, 1.000000000000000000 ) ) ;
#14152=VERTEX_POINT ( 'NONE', #80453 ) ;
#14153=CARTESIAN_POINT ( 'NONE',  ( 194.3870867008919561, 40.37665348939776777, 14.45687834341487665 ) ) ;
#14157=AXIS2_PLACEMENT_3D ( 'NONE', #86737, #58358, #7671 ) ;
#14160=ORIENTED_EDGE ( 'NONE', *, *, #2612, .T. ) ;
#14166=CARTESIAN_POINT ( 'NONE',  ( 196.4522879415759462, 72.01292343121092188, -11.25823195237581054 ) ) ;
#14179=AXIS2_PLACEMENT_3D ( 'NONE', #87575, #60132, #38787 ) ;
#14181=VERTEX_POINT ( 'NONE', #60104 ) ;
#14189=ORIENTED_EDGE ( 'NONE', *, *, #52236, .T. ) ;
#14205=ORIENTED_EDGE ( 'NONE', *, *, #66684, .T. ) ;
#14215=AXIS2_PLACEMENT_3D ( 'NONE', #20708, #78929, #13154 ) ;
#14221=CYLINDRICAL_SURFACE ( 'NONE', #92737, 2.000000000000000000 ) ;
#14222=CARTESIAN_POINT ( 'NONE',  ( 160.5350683151633291, 275.5000000000000568, 25.22542485937379553 ) ) ;
#14231=AXIS2_PLACEMENT_3D ( 'NONE', #82257, #69925, #25885 ) ;
#14233=DIRECTION ( 'NONE',  ( 0.000000000000000000, 0.000000000000000000, 1.000000000000000000 ) ) ;
#14245=CARTESIAN_POINT ( 'NONE',  ( 153.4133700136260927, 129.9709486557057119, 11.65454253063697543 ) ) ;
#14247=CARTESIAN_POINT ( 'NONE',  ( 198.9431409017138606, 67.99513008803216962, -10.39089755774709189 ) ) ;
#14258=ORIENTED_EDGE ( 'NONE', *, *, #3543, .T. ) ;
#14259=CARTESIAN_POINT ( 'NONE',  ( 138.6539576904058606, 132.0000000000000568, -10.49999999999999822 ) ) ;
#14279=ADVANCED_FACE ( 'NONE', ( #30272 ), #23639, .F. ) ;
#14282=AXIS2_PLACEMENT_3D ( 'NONE', #89880, #3247, #47729 ) ;
#14287=EDGE_LOOP ( 'NONE', ( #86540, #7193, #73675, #10545 ) ) ;
#14290=VECTOR ( 'NONE', #6067, 1000.000000000000000 ) ;
#14292=AXIS2_PLACEMENT_3D ( 'NONE', #82028, #17186, #18112 ) ;
#14298=VECTOR ( 'NONE', #64062, 1000.000000000000000 ) ;
#14303=DIRECTION ( 'NONE',  ( -0.000000000000000000, -1.000000000000000000, -0.000000000000000000 ) ) ;
#14311=AXIS2_PLACEMENT_3D ( 'NONE', #64945, #71563, #35087 ) ;
#14315=VERTEX_POINT ( 'NONE', #24091 ) ;
#14316=CARTESIAN_POINT ( 'NONE',  ( 195.7548334368592862, 25.47820008840974282, 12.44451950854168132 ) ) ;
#14326=PLANE ( 'NONE',  #6724 ) ;
#14336=EDGE_LOOP ( 'NONE', ( #86677, #8205, #46946, #61353 ) ) ;
#14343=DIRECTION ( 'NONE',  ( -0.000000000000000000, 1.000000000000000000, -0.000000000000000000 ) ) ;
#14351=DIRECTION ( 'NONE',  ( 0.000000000000000000, 1.000000000000000000, 0.000000000000000000 ) ) ;
#14354=CARTESIAN_POINT ( 'NONE',  ( 196.6744398476651554, 24.45234771250604666, 12.85662037485453268 ) ) ;
#14355=CARTESIAN_POINT ( 'NONE',  ( 159.4851178187817879, 15.28877977928778975, -9.000000000000001776 ) ) ;
#14361=AXIS2_PLACEMENT_3D ( 'NONE', #64919, #30290, #14709 ) ;
#14368=CARTESIAN_POINT ( 'NONE',  ( 197.2116943569230330, 275.5000000000000568, -12.92446933126074882 ) ) ;
#14380=EDGE_LOOP ( 'NONE', ( #51085, #20821, #59087, #49404 ) ) ;
#14384=EDGE_CURVE ( 'NONE', #64179, #82136, #52033, .T. ) ;
#14404=ORIENTED_EDGE ( 'NONE', *, *, #7520, .T. ) ;
#14444=CARTESIAN_POINT ( 'NONE',  ( 200.6103193995254230, 276.0000000000000568, -2.464576988612312114 ) ) ;
#14450=CARTESIAN_POINT ( 'NONE',  ( 175.2296996224750103, 215.0000000000000568, 0.000000000000000000 ) ) ;
#14460=DIRECTION ( 'NONE',  ( -0.000000000000000000, 0.000000000000000000, -1.000000000000000000 ) ) ;
#14463=DIRECTION ( 'NONE',  ( 0.000000000000000000, -0.000000000000000000, 1.000000000000000000 ) ) ;
#14513=EDGE_CURVE ( 'NONE', #84890, #40555, #2164, .T. ) ;
#14533=ORIENTED_EDGE ( 'NONE', *, *, #65821, .T. ) ;
#14535=DIRECTION ( 'NONE',  ( -0.000000000000000000, -0.000000000000000000, -1.000000000000000000 ) ) ;
#14542=CARTESIAN_POINT ( 'NONE',  ( 209.2607772797596226, 29.59979094061341343, 14.77866956795157094 ) ) ;
#14543=CARTESIAN_POINT ( 'NONE',  ( 164.2231345125756263, 275.5000000000000568, 22.80382896337009058 ) ) ;
#14545=CARTESIAN_POINT ( 'NONE',  ( 199.6150009768959990, 250.0000000000000568, -2.367926910627516257 ) ) ;
#14548=CARTESIAN_POINT ( 'NONE',  ( 209.2561782394521686, 27.88178916653710715, 12.07126757350762603 ) ) ;
#14562=DIRECTION ( 'NONE',  ( 0.9531768234071952284, -0.3024135303179549261, 0.000000000000000000 ) ) ;
#14563=CARTESIAN_POINT ( 'NONE',  ( 139.1539576904058606, 275.5000000000000568, 20.22542485937379908 ) ) ;
#14565=VECTOR ( 'NONE', #30208, 1000.000000000000000 ) ;
#14576=EDGE_CURVE ( 'NONE', #50286, #92859, #16075, .T. ) ;
#14579=CARTESIAN_POINT ( 'NONE',  ( 196.0722908565159344, 20.74697382034803894, 13.80893104049734177 ) ) ;
#14601=ORIENTED_EDGE ( 'NONE', *, *, #87556, .F. ) ;
#14602=DIRECTION ( 'NONE',  ( 0.000000000000000000, 1.000000000000000000, -0.000000000000000000 ) ) ;
#14604=CARTESIAN_POINT ( 'NONE',  ( 207.7755975652985114, 28.53818587417392649, 12.98477611641283858 ) ) ;
#14610=B_SPLINE_CURVE_WITH_KNOTS ( 'NONE', 3,
 ( #93631, #81631, #14127, #60353, #79457, #64352 ),
 .UNSPECIFIED., .F., .F.,
 ( 4, 2, 4 ),
 ( 0.000000000000000000, 0.0008511423910808053710, 0.001702284782161610742 ),
 .UNSPECIFIED. ) ;
#14615=VERTEX_POINT ( 'NONE', #84179 ) ;
#14628=CARTESIAN_POINT ( 'NONE',  ( 156.4851178187871312, 3.000000000000000000, -7.000000000000000888 ) ) ;
#14629=LINE ( 'NONE', #23576, #14565 ) ;
#14640=EDGE_CURVE ( 'NONE', #7049, #77260, #693, .T. ) ;
#14641=VERTEX_POINT ( 'NONE', #69062 ) ;
#14667=EDGE_LOOP ( 'NONE', ( #40791, #86707, #33545 ) ) ;
#14668=DIRECTION ( 'NONE',  ( 0.000000000000000000, 0.000000000000000000, 1.000000000000000000 ) ) ;
#14682=CARTESIAN_POINT ( 'NONE',  ( 201.2509219214787777, 65.09645894983574976, -2.633798379906725273 ) ) ;
#14683=CARTESIAN_POINT ( 'NONE',  ( 138.6539576904058606, 249.5000000000000568, -10.49999999999999822 ) ) ;
#14695=CARTESIAN_POINT ( 'NONE',  ( 198.6884013828325521, 64.61450673763175701, 9.555809373750797420 ) ) ;
#14701=ADVANCED_FACE ( 'NONE', ( #32614 ), #83712, .T. ) ;
#14703=EDGE_CURVE ( 'NONE', #11375, #13609, #26358, .T. ) ;
#14705=CARTESIAN_POINT ( 'NONE',  ( 140.6539576904058606, 131.0000000000000568, 12.50000000000000000 ) ) ;
#14708=DIRECTION ( 'NONE',  ( 0.000000000000000000, 0.000000000000000000, 1.000000000000000000 ) ) ;
#14709=DIRECTION ( 'NONE',  ( 0.000000000000000000, 0.000000000000000000, 1.000000000000000000 ) ) ;
#14718=ORIENTED_EDGE ( 'NONE', *, *, #54121, .F. ) ;
#14719=DIRECTION ( 'NONE',  ( -1.000000000000000000, 0.000000000000000000, 0.000000000000000000 ) ) ;
#14734=DIRECTION ( 'NONE',  ( 0.000000000000000000, 1.000000000000000000, 0.000000000000000000 ) ) ;
#14745=ORIENTED_EDGE ( 'NONE', *, *, #8476, .T. ) ;
#14753=ORIENTED_EDGE ( 'NONE', *, *, #59618, .F. ) ;
#14755=B_SPLINE_CURVE_WITH_KNOTS ( 'NONE', 3,
 ( #22546, #51885, #29674, #58555, #18598, #2181 ),
 .UNSPECIFIED., .F., .F.,
 ( 4, 2, 4 ),
 ( 0.0006758717013506051769, 0.002293237004444498642, 0.003910602307538392323 ),
 .UNSPECIFIED. ) ;
#14760=CARTESIAN_POINT ( 'NONE',  ( 209.1119202906403984, 36.79962757498938686, 13.15430387672353163 ) ) ;
#14772=VERTEX_POINT ( 'NONE', #55790 ) ;
#14773=CARTESIAN_POINT ( 'NONE',  ( 175.2296996224750103, 275.0000000000000568, 0.000000000000000000 ) ) ;
#14783=DIRECTION ( 'NONE',  ( -0.000000000000000000, -1.000000000000000000, -0.000000000000000000 ) ) ;
#14798=CARTESIAN_POINT ( 'NONE',  ( 197.7953982265470927, 19.09807621135326272, -10.91506350946106885 ) ) ;
#14803=ADVANCED_FACE ( 'NONE', ( #39671 ), #48662, .T. ) ;
#14805=CARTESIAN_POINT ( 'NONE',  ( 204.6539576904058606, 293.9636489450775230, 0.000000000000000000 ) ) ;
#14807=FACE_OUTER_BOUND ( 'NONE', #30810, .T. ) ;
#14810=DIRECTION ( 'NONE',  ( 0.8786741093294601068, 0.000000000000000000, 0.4774220455677345987 ) ) ;
#14811=CARTESIAN_POINT ( 'NONE',  ( 157.3397966316789507, 16.44589409474725272, -9.145321187104729077 ) ) ;
#14820=AXIS2_PLACEMENT_3D ( 'NONE', #10486, #1536, #38446 ) ;
#14834=VERTEX_POINT ( 'NONE', #18390 ) ;
#14838=FACE_OUTER_BOUND ( 'NONE', #91034, .T. ) ;
#14856=VERTEX_POINT ( 'NONE', #69993 ) ;
#14859=VERTEX_POINT ( 'NONE', #4191 ) ;
#14883=EDGE_LOOP ( 'NONE', ( #16371, #71606, #28625, #60726 ) ) ;
#14886=ORIENTED_EDGE ( 'NONE', *, *, #6237, .F. ) ;
#14906=CARTESIAN_POINT ( 'NONE',  ( 155.1244896729743061, 20.04296953158445405, 14.86678859757276427 ) ) ;
#14921=ADVANCED_FACE ( 'NONE', ( #39209 ), #68123, .T. ) ;
#14946=AXIS2_PLACEMENT_3D ( 'NONE', #47120, #76968, #63261 ) ;
#14982=ORIENTED_EDGE ( 'NONE', *, *, #50431, .F. ) ;
#14984=CARTESIAN_POINT ( 'NONE',  ( 196.8928068234201021, 24.78327594025822478, 12.47839767815188061 ) ) ;
#14997=CYLINDRICAL_SURFACE ( 'NONE', #27789, 3.842139515347647638 ) ;
#15001=ADVANCED_FACE ( 'NONE', ( #75684 ), #5133, .F. ) ;
#15011=CARTESIAN_POINT ( 'NONE',  ( 196.1162889029012319, 19.88370459728183448, 13.75220701793647926 ) ) ;
#15026=DIRECTION ( 'NONE',  ( 0.000000000000000000, 0.000000000000000000, 1.000000000000000000 ) ) ;
#15031=EDGE_CURVE ( 'NONE', #44024, #2170, #86844, .T. ) ;
#15049=EDGE_LOOP ( 'NONE', ( #44650, #53933, #77996, #3449 ) ) ;
#15050=CARTESIAN_POINT ( 'NONE',  ( 197.7152286749091559, 70.58179843880969884, 11.36775530991498506 ) ) ;
#15061=ORIENTED_EDGE ( 'NONE', *, *, #67975, .F. ) ;
#15062=DIRECTION ( 'NONE',  ( 1.000000000000000000, 0.000000000000000000, -0.000000000000000000 ) ) ;
#15074=FACE_OUTER_BOUND ( 'NONE', #6233, .T. ) ;
#15079=VERTEX_POINT ( 'NONE', #25951 ) ;
#15094=EDGE_CURVE ( 'NONE', #82861, #24854, #33525, .T. ) ;
#15096=CARTESIAN_POINT ( 'NONE',  ( 156.8306019976938046, 250.3431421874260252, 16.89650703080528515 ) ) ;
#15109=EDGE_LOOP ( 'NONE', ( #64586, #69446, #34865, #39805 ) ) ;
#15110=B_SPLINE_CURVE_WITH_KNOTS ( 'NONE', 3,
 ( #24954, #18304, #17848, #33439, #54744, #46241 ),
 .UNSPECIFIED., .F., .F.,
 ( 4, 2, 4 ),
 ( 0.000000000000000000, 0.001028964506245427356, 0.002057929012490854713 ),
 .UNSPECIFIED. ) ;
#15139=CARTESIAN_POINT ( 'NONE',  ( 219.8344101925596021, 0.000000000000000000, -9.000000000000001776 ) ) ;
#15141=AXIS2_PLACEMENT_3D ( 'NONE', #47856, #69653, #53581 ) ;
#15142=CARTESIAN_POINT ( 'NONE',  ( 200.4738562182569694, 293.9636489450776367, -44.00000000000000000 ) ) ;
#15152=CARTESIAN_POINT ( 'NONE',  ( 192.9623460957494956, 276.0000000000000568, 16.90571646082668522 ) ) ;
#15156=CARTESIAN_POINT ( 'NONE',  ( 198.0747767758275870, 67.35440902555335185, -11.09512694806112698 ) ) ;
#15157=DIRECTION ( 'NONE',  ( -0.000000000000000000, -1.000000000000000000, -0.000000000000000000 ) ) ;
#15166=VERTEX_POINT ( 'NONE', #77091 ) ;
#15167=CARTESIAN_POINT ( 'NONE',  ( 201.2849759805909571, 65.05171340438639049, -7.254661561165801409 ) ) ;
#15169=DIRECTION ( 'NONE',  ( 0.000000000000000000, -0.000000000000000000, 1.000000000000000000 ) ) ;
#15179=VERTEX_POINT ( 'NONE', #19793 ) ;
#15183=DIRECTION ( 'NONE',  ( -1.000000000000000000, 0.000000000000000000, 0.000000000000000000 ) ) ;
#15201=VECTOR ( 'NONE', #29265, 1000.000000000000000 ) ;
#15203=EDGE_LOOP ( 'NONE', ( #142, #22664, #47855, #3328, #71908 ) ) ;
#15224=CARTESIAN_POINT ( 'NONE',  ( 194.9478318536113477, 25.16799831920036823, 13.68273651490584975 ) ) ;
#15247=CARTESIAN_POINT ( 'NONE',  ( 170.2296700125738198, 215.0000000000000568, -24.97289011430693151 ) ) ;
#15255=CARTESIAN_POINT ( 'NONE',  ( 201.2104617360081704, 25.32700003806617772, 9.999999999999998224 ) ) ;
#15258=DIRECTION ( 'NONE',  ( 0.000000000000000000, 0.000000000000000000, 1.000000000000000000 ) ) ;
#15267=EDGE_CURVE ( 'NONE', #13153, #64177, #50151, .T. ) ;
#15269=ORIENTED_EDGE ( 'NONE', *, *, #56521, .F. ) ;
#15272=AXIS2_PLACEMENT_3D ( 'NONE', #57470, #44149, #78768 ) ;
#15274=CARTESIAN_POINT ( 'NONE',  ( 197.0527519259912879, 24.77614581236855074, 12.20486921435629846 ) ) ;
#15278=VECTOR ( 'NONE', #9930, 1000.000000000000000 ) ;
#15289=CARTESIAN_POINT ( 'NONE',  ( 200.7454649163835541, 299.8601228333361632, -5.413818927456778951 ) ) ;
#15292=DIRECTION ( 'NONE',  ( -1.000000000000000000, 0.000000000000000000, 0.000000000000000000 ) ) ;
#15306=ORIENTED_EDGE ( 'NONE', *, *, #8208, .F. ) ;
#15328=EDGE_CURVE ( 'NONE', #65802, #1567, #77399, .T. ) ;
#15340=ORIENTED_EDGE ( 'NONE', *, *, #68145, .T. ) ;
#15371=DIRECTION ( 'NONE',  ( -1.000000000000000000, 0.000000000000000000, 0.000000000000000000 ) ) ;
#15403=AXIS2_PLACEMENT_3D ( 'NONE', #23490, #80310, #90086 ) ;
#15405=AXIS2_PLACEMENT_3D ( 'NONE', #72555, #1502, #37476 ) ;
#15423=EDGE_CURVE ( 'NONE', #71244, #74736, #57744, .T. ) ;
#15426=DIRECTION ( 'NONE',  ( 0.6056179655966483777, -0.7957555401921979632, -1.840554422280015381E-15 ) ) ;
#15433=ADVANCED_FACE ( 'NONE', ( #50064 ), #34479, .F. ) ;
#15442=ORIENTED_EDGE ( 'NONE', *, *, #82641, .T. ) ;
#15443=CARTESIAN_POINT ( 'NONE',  ( 208.4306832106271088, -74.55766379199613425, 0.000000000000000000 ) ) ;
#15448=CARTESIAN_POINT ( 'NONE',  ( 160.5350683151633291, 250.0000000000000568, 20.22542485937379908 ) ) ;
#15449=CYLINDRICAL_SURFACE ( 'NONE', #59273, 4.025000000000000355 ) ;
#15454=CARTESIAN_POINT ( 'NONE',  ( 199.9517221346984002, 40.04024871352131498, 9.062294003318640989 ) ) ;
#15462=AXIS2_PLACEMENT_3D ( 'NONE', #12551, #55177, #69370 ) ;
#15471=TOROIDAL_SURFACE ( 'NONE', #86492, 5.603083949679977138, 0.5000000000000000000 ) ;
#15478=CARTESIAN_POINT ( 'NONE',  ( 154.5625123364531817, 249.5000000000000568, -13.15740740740742076 ) ) ;
#15492=CARTESIAN_POINT ( 'NONE',  ( 210.7238915819278589, 32.98517505407394168, 12.09245862095555601 ) ) ;
#15507=EDGE_LOOP ( 'NONE', ( #32884, #10721, #24627, #68792 ) ) ;
#15508=CARTESIAN_POINT ( 'NONE',  ( 199.8761955117210221, 66.90278937422385752, 8.069515584579029621 ) ) ;
#15520=CARTESIAN_POINT ( 'NONE',  ( 220.4471435719830197, 34.91984470236808136, -9.000000000000001776 ) ) ;
#15525=EDGE_CURVE ( 'NONE', #75506, #6373, #36562, .T. ) ;
#15538=ORIENTED_EDGE ( 'NONE', *, *, #46974, .T. ) ;
#15556=EDGE_CURVE ( 'NONE', #48224, #74021, #36715, .T. ) ;
#15558=CARTESIAN_POINT ( 'NONE',  ( 175.2296996224749250, 215.0000000000000568, -24.99999999999999289 ) ) ;
#15567=CARTESIAN_POINT ( 'NONE',  ( 198.8656410362497695, 68.63459961102830675, -9.310658723936024117 ) ) ;
#15572=ORIENTED_EDGE ( 'NONE', *, *, #30621, .T. ) ;
#15573=VERTEX_POINT ( 'NONE', #49147 ) ;
#15574=CARTESIAN_POINT ( 'NONE',  ( 195.7540919006722504, 41.65591105122726390, 14.27491332538345148 ) ) ;
#15597=AXIS2_PLACEMENT_3D ( 'NONE', #49250, #460, #51104 ) ;
#15599=DIRECTION ( 'NONE',  ( 0.000000000000000000, 0.000000000000000000, -1.000000000000000000 ) ) ;
#15612=AXIS2_PLACEMENT_3D ( 'NONE', #15955, #2213, #45730 ) ;
#15616=CYLINDRICAL_SURFACE ( 'NONE', #14361, 5.999999999999998224 ) ;
#15627=AXIS2_PLACEMENT_3D ( 'NONE', #21779, #42119, #79989 ) ;
#15630=FACE_OUTER_BOUND ( 'NONE', #33085, .T. ) ;
#15639=VERTEX_POINT ( 'NONE', #42974 ) ;
#15647=DIRECTION ( 'NONE',  ( 0.000000000000000000, 1.000000000000000000, 0.000000000000000000 ) ) ;
#15656=ORIENTED_EDGE ( 'NONE', *, *, #1219, .T. ) ;
#15662=EDGE_CURVE ( 'NONE', #15179, #89341, #7449, .T. ) ;
#15663=EDGE_CURVE ( 'NONE', #50862, #35587, #64334, .T. ) ;
#15666=ORIENTED_EDGE ( 'NONE', *, *, #32210, .T. ) ;
#15667=CIRCLE ( 'NONE', #53445, 24.50000000000000355 ) ;
#15669=VECTOR ( 'NONE', #21636, 1000.000000000000000 ) ;
#15675=DIRECTION ( 'NONE',  ( -0.9693563597868452009, -0.2456588035076220644, -3.046750416192724932E-15 ) ) ;
#15691=AXIS2_PLACEMENT_3D ( 'NONE', #6767, #14343, #21419 ) ;
#15701=CARTESIAN_POINT ( 'NONE',  ( 222.8344101925596306, 36.73669859915801794, 10.00000000000000000 ) ) ;
#15709=ORIENTED_EDGE ( 'NONE', *, *, #51565, .F. ) ;
#15716=B_SPLINE_CURVE_WITH_KNOTS ( 'NONE', 3,
 ( #52129, #9023, #24170, #52582 ),
 .UNSPECIFIED., .F., .F.,
 ( 4, 4 ),
 ( 0.000000000000000000, 0.0008009674008373282583 ),
 .UNSPECIFIED. ) ;
#15717=FACE_OUTER_BOUND ( 'NONE', #81090, .T. ) ;
#15725=DIRECTION ( 'NONE',  ( 0.000000000000000000, 0.000000000000000000, 1.000000000000000000 ) ) ;
#15728=CARTESIAN_POINT ( 'NONE',  ( 196.8803347170859865, 24.42324672360809856, 12.49999999999999289 ) ) ;
#15739=B_SPLINE_CURVE_WITH_KNOTS ( 'NONE', 3,
 ( #10300, #9844, #39626, #17891, #2294, #61912 ),
 .UNSPECIFIED., .F., .F.,
 ( 4, 2, 4 ),
 ( -4.472146915497830869E-06, 0.0004206930844425595313, 0.0008458583158006168900 ),
 .UNSPECIFIED. ) ;
#15741=TOROIDAL_SURFACE ( 'NONE', #42980, 2.500000000000007994, 0.5000000000000000000 ) ;
#15745=CARTESIAN_POINT ( 'NONE',  ( 189.9243309297870610, 249.5000000000000568, 20.22542485937349355 ) ) ;
#15759=AXIS2_PLACEMENT_3D ( 'NONE', #12406, #6247, #63570 ) ;
#15760=DIRECTION ( 'NONE',  ( -0.000000000000000000, -0.000000000000000000, -1.000000000000000000 ) ) ;
#15778=VERTEX_POINT ( 'NONE', #64790 ) ;
#15781=EDGE_LOOP ( 'NONE', ( #13494, #40545, #58785, #75929 ) ) ;
#15791=VERTEX_POINT ( 'NONE', #28773 ) ;
#15802=ORIENTED_EDGE ( 'NONE', *, *, #55196, .F. ) ;
#15807=ADVANCED_FACE ( 'NONE', ( #92216 ), #57656, .F. ) ;
#15810=ORIENTED_EDGE ( 'NONE', *, *, #20342, .T. ) ;
#15830=CARTESIAN_POINT ( 'NONE',  ( 175.2296996224750103, 247.0000000000001137, 0.000000000000000000 ) ) ;
#15837=DIRECTION ( 'NONE',  ( 0.000000000000000000, 0.000000000000000000, 1.000000000000000000 ) ) ;
#15840=DIRECTION ( 'NONE',  ( -0.000000000000000000, -1.000000000000000000, -0.000000000000000000 ) ) ;
#15844=CARTESIAN_POINT ( 'NONE',  ( 180.5131398354828320, 275.5000000000000568, -23.92352941176473635 ) ) ;
#15848=CARTESIAN_POINT ( 'NONE',  ( 201.2104617360081704, 60.19600395700749829, -10.00000000000000000 ) ) ;
#15859=CARTESIAN_POINT ( 'NONE',  ( 169.9358031814915080, 214.6007075219706621, -24.43326837773184934 ) ) ;
#15864=EDGE_CURVE ( 'NONE', #4269, #52800, #42738, .T. ) ;
#15867=CIRCLE ( 'NONE', #80874, 4.999999999999984013 ) ;
#15897=AXIS2_PLACEMENT_3D ( 'NONE', #76173, #2803, #39220 ) ;
#15904=DIRECTION ( 'NONE',  ( -0.000000000000000000, -1.000000000000000000, 0.000000000000000000 ) ) ;
#15914=AXIS2_PLACEMENT_3D ( 'NONE', #17430, #69018, #74720 ) ;
#15921=LINE ( 'NONE', #8336, #88543 ) ;
#15923=B_SPLINE_CURVE_WITH_KNOTS ( 'NONE', 3,
 ( #23125, #52935, #45826, #68090 ),
 .UNSPECIFIED., .F., .F.,
 ( 4, 4 ),
 ( 0.000000000000000000, 0.001074155171061463854 ),
 .UNSPECIFIED. ) ;
#15927=CARTESIAN_POINT ( 'NONE',  ( 209.4952545125645145, 27.94237698917519452, 13.96055292456872898 ) ) ;
#15928=DIRECTION ( 'NONE',  ( -0.000000000000000000, 1.000000000000000000, -0.000000000000000000 ) ) ;
#15933=ORIENTED_EDGE ( 'NONE', *, *, #37438, .T. ) ;
#15934=DIRECTION ( 'NONE',  ( -0.8660254037844410391, 0.000000000000000000, -0.4999999999999960032 ) ) ;
#15946=CARTESIAN_POINT ( 'NONE',  ( 196.7383257810085979, 24.47698789593438917, 11.00000000000000000 ) ) ;
#15955=CARTESIAN_POINT ( 'NONE',  ( 197.2116943569230330, 250.5000000000000568, -12.92446933126074882 ) ) ;
#15960=CARTESIAN_POINT ( 'NONE',  ( 175.2296996224749250, 275.5000000000000568, -24.99999999999999289 ) ) ;
#15963=DIRECTION ( 'NONE',  ( 0.000000000000000000, -1.000000000000000000, 0.000000000000000000 ) ) ;
#15969=CARTESIAN_POINT ( 'NONE',  ( 150.6539576904058606, 293.9636489450775230, 0.000000000000000000 ) ) ;
#15987=VERTEX_POINT ( 'NONE', #73265 ) ;
#15988=CARTESIAN_POINT ( 'NONE',  ( 198.9432932128748632, 67.99483610340296025, 10.39078689545250711 ) ) ;
#15999=ORIENTED_EDGE ( 'NONE', *, *, #11999, .T. ) ;
#16000=CARTESIAN_POINT ( 'NONE',  ( 195.4987509559167904, 41.28370916884458808, 12.85659709285176611 ) ) ;
#16010=CARTESIAN_POINT ( 'NONE',  ( 202.9738562182569694, 293.9636489450776367, -54.00000000000000000 ) ) ;
#16011=DIRECTION ( 'NONE',  ( -0.000000000000000000, -1.000000000000000000, -0.000000000000000000 ) ) ;
#16041=CARTESIAN_POINT ( 'NONE',  ( 199.3803347170859865, 17.19615242270662847, 9.999999999999996447 ) ) ;
#16043=CIRCLE ( 'NONE', #75048, 1.999999999999988454 ) ;
#16048=CARTESIAN_POINT ( 'NONE',  ( 200.7741138073446621, 15.52361751443386950, -10.00000000000000178 ) ) ;
#16062=LINE ( 'NONE', #2779, #64023 ) ;
#16074=EDGE_CURVE ( 'NONE', #23459, #55526, #38030, .T. ) ;
#16075=LINE ( 'NONE', #30744, #38434 ) ;
#16085=CARTESIAN_POINT ( 'NONE',  ( 154.7659666677267580, 19.56018909072085066, 12.94946946941272437 ) ) ;
#16095=EDGE_CURVE ( 'NONE', #35594, #57506, #9303, .T. ) ;
#16102=DIRECTION ( 'NONE',  ( 0.000000000000000000, 1.000000000000000000, 0.000000000000000000 ) ) ;
#16112=VERTEX_POINT ( 'NONE', #23977 ) ;
#16116=DIRECTION ( 'NONE',  ( -0.9693563597868444237, -0.2456588035076248677, 0.000000000000000000 ) ) ;
#16119=FACE_OUTER_BOUND ( 'NONE', #93470, .T. ) ;
#16134=ORIENTED_EDGE ( 'NONE', *, *, #58215, .F. ) ;
#16141=CARTESIAN_POINT ( 'NONE',  ( 197.5379522065468052, 275.5000000000000568, -11.97918851819043873 ) ) ;
#16153=AXIS2_PLACEMENT_3D ( 'NONE', #89926, #25082, #53956 ) ;
#16163=CARTESIAN_POINT ( 'NONE',  ( 209.2250871165752244, 35.77521060175700995, 15.12480380946217728 ) ) ;
#16183=FACE_OUTER_BOUND ( 'NONE', #49908, .T. ) ;
#16185=CARTESIAN_POINT ( 'NONE',  ( 175.2296996224750103, 21.00000000000000000, 0.000000000000000000 ) ) ;
#16198=ADVANCED_FACE ( 'NONE', ( #59989 ), #48651, .F. ) ;
#16201=ORIENTED_EDGE ( 'NONE', *, *, #67721, .F. ) ;
#16217=CARTESIAN_POINT ( 'NONE',  ( 164.7123623445222904, 2.999999999999999112, 9.000000000000001776 ) ) ;
#16220=CARTESIAN_POINT ( 'NONE',  ( 198.1329898669367253, 69.92583464099142532, -8.330337636095675791 ) ) ;
#16237=ORIENTED_EDGE ( 'NONE', *, *, #26328, .F. ) ;
#16257=ORIENTED_EDGE ( 'NONE', *, *, #63294, .T. ) ;
#16264=VERTEX_POINT ( 'NONE', #72781 ) ;
#16265=FACE_BOUND ( 'NONE', #80655, .T. ) ;
#16269=VERTEX_POINT ( 'NONE', #74646 ) ;
#16285=CARTESIAN_POINT ( 'NONE',  ( 208.8440659120965108, 36.55262022383305975, 14.73366904486404572 ) ) ;
#16299=DIRECTION ( 'NONE',  ( -0.3994899938747897283, 0.000000000000000000, 0.9167375550253848981 ) ) ;
#16303=CARTESIAN_POINT ( 'NONE',  ( 200.4816938276917995, 61.72811464988816965, -9.999999999999998224 ) ) ;
#16315=CARTESIAN_POINT ( 'NONE',  ( 189.9243309297870610, 275.5000000000000568, 20.22542485937349355 ) ) ;
#16325=EDGE_CURVE ( 'NONE', #71428, #12480, #67085, .T. ) ;
#16334=EDGE_CURVE ( 'NONE', #22603, #68073, #41056, .T. ) ;
#16356=AXIS2_PLACEMENT_3D ( 'NONE', #64007, #51607, #50705 ) ;
#16358=CARTESIAN_POINT ( 'NONE',  ( 138.6539576904058606, 275.5000000000000568, -10.49999999999999822 ) ) ;
#16371=ORIENTED_EDGE ( 'NONE', *, *, #47694, .T. ) ;
#16372=CARTESIAN_POINT ( 'NONE',  ( 186.6539576904058890, 293.9636489450775230, 0.000000000000000000 ) ) ;
#16375=B_SPLINE_CURVE_WITH_KNOTS ( 'NONE', 3,
 ( #17516, #46367, #75269, #10383, #39251, #68166, #17971, #61542 ),
 .UNSPECIFIED., .F., .F.,
 ( 4, 2, 2, 4 ),
 ( -4.472612521061044141E-06, 0.0004667749420422289872, 0.0007023987193238740313, 0.0009380224966055190211 ),
 .UNSPECIFIED. ) ;
#16379=DIRECTION ( 'NONE',  ( 0.000000000000000000, 0.000000000000000000, 1.000000000000000000 ) ) ;
#16386=CARTESIAN_POINT ( 'NONE',  ( 197.8233505269066370, 40.71551520756617037, 11.52974254711199364 ) ) ;
#16399=CARTESIAN_POINT ( 'NONE',  ( 211.1232656141943949, 1.000000000000000000, -7.000000000000000888 ) ) ;
#16408=DIRECTION ( 'NONE',  ( 1.000000000000000000, 0.000000000000000000, 0.000000000000000000 ) ) ;
#16409=CARTESIAN_POINT ( 'NONE',  ( 175.2296996224750103, 15.00000000000000000, -15.00000000000000000 ) ) ;
#16417=DIRECTION ( 'NONE',  ( 0.5000000000000032196, -0.8660254037844368202, 0.000000000000000000 ) ) ;
#16418=AXIS2_PLACEMENT_3D ( 'NONE', #54705, #5002, #26307 ) ;
#16442=CARTESIAN_POINT ( 'NONE',  ( 199.1087447750284980, 64.61450673763174279, 10.46317447812566392 ) ) ;
#16444=LINE ( 'NONE', #9318, #70127 ) ;
#16453=ORIENTED_EDGE ( 'NONE', *, *, #88447, .F. ) ;
#16485=CARTESIAN_POINT ( 'NONE',  ( 150.4957602436334412, 20.99999999999998934, 3.637614988394418880 ) ) ;
#16487=LINE ( 'NONE', #80886, #41179 ) ;
#16496=EDGE_CURVE ( 'NONE', #16264, #51979, #10861, .T. ) ;
#16497=CARTESIAN_POINT ( 'NONE',  ( 207.2816333161762543, 35.50654163870040492, 14.49999997652496475 ) ) ;
#16502=ORIENTED_EDGE ( 'NONE', *, *, #67573, .T. ) ;
#16503=CARTESIAN_POINT ( 'NONE',  ( 196.2760846862214805, 19.11198087481130514, -12.12215979492470552 ) ) ;
#16517=CARTESIAN_POINT ( 'NONE',  ( 196.7806748523260012, 214.5000000000000568, -12.67104836398113576 ) ) ;
#16541=DIRECTION ( 'NONE',  ( 0.000000000000000000, 0.000000000000000000, -1.000000000000000000 ) ) ;
#16549=AXIS2_PLACEMENT_3D ( 'NONE', #92578, #13541, #18767 ) ;
#16552=EDGE_LOOP ( 'NONE', ( #48242, #79857, #31588, #59612 ) ) ;
#16553=CARTESIAN_POINT ( 'NONE',  ( 203.5977283565847529, 62.01285785379746329, -9.999999999999998224 ) ) ;
#16566=ORIENTED_EDGE ( 'NONE', *, *, #40929, .T. ) ;
#16570=CARTESIAN_POINT ( 'NONE',  ( 196.7672805984238096, 69.63494095281957641, 10.95706626401136141 ) ) ;
#16581=EDGE_LOOP ( 'NONE', ( #87257, #17416, #90395, #69752, #9102 ) ) ;
#16586=ADVANCED_FACE ( 'NONE', ( #24439 ), #21427, .T. ) ;
#16590=VERTEX_POINT ( 'NONE', #67551 ) ;
#16598=CARTESIAN_POINT ( 'NONE',  ( 208.9422428205583344, 36.81742993605089964, 13.19543921975815692 ) ) ;
#16602=ADVANCED_FACE ( 'NONE', ( #87432 ), #82205, .T. ) ;
#16622=AXIS2_PLACEMENT_3D ( 'NONE', #76693, #61108, #4254 ) ;
#16639=CYLINDRICAL_SURFACE ( 'NONE', #27507, 4.999999999999986677 ) ;
#16641=CARTESIAN_POINT ( 'NONE',  ( 197.8939195897753223, 25.00231265943466497, 11.19330938564888100 ) ) ;
#16644=CARTESIAN_POINT ( 'NONE',  ( 200.1223792991399364, 214.7033776542919270, -2.619521892235705973 ) ) ;
#16654=ORIENTED_EDGE ( 'NONE', *, *, #82838, .F. ) ;
#16670=CARTESIAN_POINT ( 'NONE',  ( 158.9078607026168868, 16.88031981475927878, 10.36078569760431201 ) ) ;
#16672=VECTOR ( 'NONE', #88753, 1000.000000000000114 ) ;
#16676=AXIS2_PLACEMENT_3D ( 'NONE', #6426, #35301, #19223 ) ;
#16688=ORIENTED_EDGE ( 'NONE', *, *, #47145, .T. ) ;
#16712=ORIENTED_EDGE ( 'NONE', *, *, #44600, .T. ) ;
#16719=EDGE_LOOP ( 'NONE', ( #73303, #35182, #69696, #45107, #41644 ) ) ;
#16720=CARTESIAN_POINT ( 'NONE',  ( 157.3189109369757546, 16.43186977800927906, 7.221609175748572973 ) ) ;
#16723=EDGE_CURVE ( 'NONE', #24735, #4620, #27515, .T. ) ;
#16726=VERTEX_POINT ( 'NONE', #82666 ) ;
#16740=FACE_OUTER_BOUND ( 'NONE', #82408, .T. ) ;
#16745=( BOUNDED_SURFACE ( )  B_SPLINE_SURFACE ( 3, 2, ( 
 ( #36205, #29106, #65123 ),
 ( #58000, #86856, #22012 ),
 ( #50882, #14906, #43762 ),
 ( #72662, #703, #44694 ),
 ( #82069, #30497, #23402 ),
 ( #9162, #87769, #66495 ) ),
 .UNSPECIFIED., .F., .F., .F. ) 
 B_SPLINE_SURFACE_WITH_KNOTS ( ( 4, 2, 4 ),
 ( 3, 3 ),
 ( 0.000000000000000000, 0.001526582434089618920, 0.003053164868179237840 ),
 ( 0.000000000000000000, 1.000000000000000000 ),
 .UNSPECIFIED. ) 
 GEOMETRIC_REPRESENTATION_ITEM ( )  RATIONAL_B_SPLINE_SURFACE ( (
 ( 1.000000000000000000, 0.7071067811865475727, 1.000000000000000000),
 ( 1.000000000000000000, 0.7219865977747690344, 1.000000000000000000),
 ( 1.000000000000000000, 0.7353530398652478040, 1.000000000000000000),
 ( 1.000000000000000000, 0.7593109839642017134, 1.000000000000000000),
 ( 1.000000000000000000, 0.7699014431358252031, 1.000000000000000000),
 ( 1.000000000000000000, 0.7791885400064315625, 1.000000000000000000) ) ) 
 REPRESENTATION_ITEM ( '' )  SURFACE ( )  );
#16752=CARTESIAN_POINT ( 'NONE',  ( 194.7272697300732887, 19.95005744978422157, 14.17304058800352884 ) ) ;
#16756=CARTESIAN_POINT ( 'NONE',  ( 195.2310442527411567, 19.79200657291019283, 13.55662862596270557 ) ) ;
#16760=FACE_OUTER_BOUND ( 'NONE', #43472, .T. ) ;
#16775=CARTESIAN_POINT ( 'NONE',  ( 165.2494399300530290, 8.542400036368780647, 25.74970488511327815 ) ) ;
#16778=DIRECTION ( 'NONE',  ( 0.000000000000000000, 0.000000000000000000, 1.000000000000000000 ) ) ;
#16797=CARTESIAN_POINT ( 'NONE',  ( 184.7149167944524493, 8.542400036368780647, 9.000000000000001776 ) ) ;
#16822=VECTOR ( 'NONE', #52194, 1000.000000000000000 ) ;
#16833=VERTEX_POINT ( 'NONE', #62309 ) ;
#16834=CARTESIAN_POINT ( 'NONE',  ( 198.6353741166566920, 66.99406408877143804, -8.405752120499668578 ) ) ;
#16836=ADVANCED_FACE ( 'NONE', ( #48073 ), #84065, .F. ) ;
#16841=CARTESIAN_POINT ( 'NONE',  ( 159.4851178187871312, 15.00000000000000000, -10.00000000000000000 ) ) ;
#16847=CARTESIAN_POINT ( 'NONE',  ( 196.5738014817347334, 41.11195847892594202, 11.18394375856346556 ) ) ;
#16862=CARTESIAN_POINT ( 'NONE',  ( 199.4767649826798674, 24.99747890858082044, 8.999999999999998224 ) ) ;
#16871=CARTESIAN_POINT ( 'NONE',  ( 201.2104617360081704, 15.00000000000000000, 9.000000000000001776 ) ) ;
#16872=FACE_OUTER_BOUND ( 'NONE', #14287, .T. ) ;
#16877=DIRECTION ( 'NONE',  ( 0.000000000000000000, 0.000000000000000000, 1.000000000000000000 ) ) ;
#16880=LINE ( 'NONE', #44817, #38249 ) ;
#16883=CIRCLE ( 'NONE', #15403, 4.003189038634634045 ) ;
#16885=VECTOR ( 'NONE', #65285, 1000.000000000000000 ) ;
#16894=AXIS2_PLACEMENT_3D ( 'NONE', #14111, #43433, #70477 ) ;
#16907=ORIENTED_EDGE ( 'NONE', *, *, #19092, .T. ) ;
#16920=DIRECTION ( 'NONE',  ( 1.110223024625156343E-15, 0.000000000000000000, 1.000000000000000000 ) ) ;
#16934=EDGE_LOOP ( 'NONE', ( #71702, #31600, #15810, #82519 ) ) ;
#16950=CARTESIAN_POINT ( 'NONE',  ( 156.5440870305766055, 214.9910457053126720, 17.21343741151179429 ) ) ;
#16951=AXIS2_PLACEMENT_3D ( 'NONE', #37573, #10094, #53666 ) ;
#16952=DIRECTION ( 'NONE',  ( 1.000000000000000000, -0.000000000000000000, -0.000000000000000000 ) ) ;
#16953=CIRCLE ( 'NONE', #71386, 0.5000000000000004441 ) ;
#16961=DIRECTION ( 'NONE',  ( 0.000000000000000000, 0.000000000000000000, -1.000000000000000000 ) ) ;
#16962=CIRCLE ( 'NONE', #45663, 1.000000000000009104 ) ;
#16965=ORIENTED_EDGE ( 'NONE', *, *, #73478, .F. ) ;
#16970=EDGE_CURVE ( 'NONE', #52528, #68989, #68235, .T. ) ;
#16983=DIRECTION ( 'NONE',  ( -0.000000000000000000, -0.000000000000000000, 1.000000000000000000 ) ) ;
#16991=CARTESIAN_POINT ( 'NONE',  ( 154.5816620007682047, 19.45641339818851279, 12.71868198592549781 ) ) ;
#17007=DIRECTION ( 'NONE',  ( 0.8620390091940267618, 0.000000000000000000, -0.5068419345592672931 ) ) ;
#17016=CIRCLE ( 'NONE', #1944, 2.000000000000001776 ) ;
#17019=CARTESIAN_POINT ( 'NONE',  ( 199.7648473163356186, 63.23516263142278859, -10.15923027031813675 ) ) ;
#17023=CARTESIAN_POINT ( 'NONE',  ( 160.5350683151633291, 276.0000000000000568, 20.22542485937379908 ) ) ;
#17026=EDGE_CURVE ( 'NONE', #55975, #12630, #24456, .T. ) ;
#17040=CARTESIAN_POINT ( 'NONE',  ( 197.4232884941380632, 67.42303550333971884, 10.33355363093519408 ) ) ;
#17043=DIRECTION ( 'NONE',  ( 0.000000000000000000, 0.000000000000000000, 1.000000000000000000 ) ) ;
#17051=CIRCLE ( 'NONE', #82062, 0.5000000000000016653 ) ;
#17066=DIRECTION ( 'NONE',  ( 1.000000000000000000, -0.000000000000000000, -0.000000000000000000 ) ) ;
#17078=DIRECTION ( 'NONE',  ( 0.000000000000000000, 0.000000000000000000, 1.000000000000000000 ) ) ;
#17080=AXIS2_PLACEMENT_3D ( 'NONE', #35976, #49707, #71037 ) ;
#17089=CARTESIAN_POINT ( 'NONE',  ( 208.9648513981561564, 35.82080690278420576, 15.11414978972049106 ) ) ;
#17090=CIRCLE ( 'NONE', #41249, 24.00000000000000355 ) ;
#17094=CIRCLE ( 'NONE', #35213, 0.5000000000000004441 ) ;
#17103=CARTESIAN_POINT ( 'NONE',  ( 139.1539576904058606, 276.0000000000000568, 10.50000000000000000 ) ) ;
#17105=FACE_OUTER_BOUND ( 'NONE', #78446, .T. ) ;
#17108=AXIS2_PLACEMENT_3D ( 'NONE', #24442, #52854, #44357 ) ;
#17115=CIRCLE ( 'NONE', #51908, 24.00000000000000000 ) ;
#17116=PLANE ( 'NONE',  #12022 ) ;
#17119=DIRECTION ( 'NONE',  ( -0.000000000000000000, -1.000000000000000000, -0.000000000000000000 ) ) ;
#17129=CARTESIAN_POINT ( 'NONE',  ( 160.5350683151633575, 275.5000000000000568, -11.99999999999998934 ) ) ;
#17135=EDGE_CURVE ( 'NONE', #77618, #3669, #65394, .T. ) ;
#17145=CARTESIAN_POINT ( 'NONE',  ( 185.8445586754484964, 214.9970011440365454, 23.11617803653495784 ) ) ;
#17149=STYLED_ITEM('',(#93738),#26626);
#17151=AXIS2_PLACEMENT_3D ( 'NONE', #8568, #60647, #53533 ) ;
#17159=AXIS2_PLACEMENT_3D ( 'NONE', #33889, #48068, #18270 ) ;
#17165=VERTEX_POINT ( 'NONE', #83591 ) ;
#17168=VERTEX_POINT ( 'NONE', #75571 ) ;
#17174=DIRECTION ( 'NONE',  ( -1.000000000000000000, 0.000000000000000000, 0.000000000000000000 ) ) ;
#17179=ORIENTED_EDGE ( 'NONE', *, *, #38393, .T. ) ;
#17182=CIRCLE ( 'NONE', #42930, 9.103929867429224387 ) ;
#17186=DIRECTION ( 'NONE',  ( -1.000000000000000000, 0.000000000000000000, 0.000000000000000000 ) ) ;
#17192=ORIENTED_EDGE ( 'NONE', *, *, #38171, .T. ) ;
#17199=ORIENTED_EDGE ( 'NONE', *, *, #78108, .F. ) ;
#17204=ORIENTED_EDGE ( 'NONE', *, *, #5180, .F. ) ;
#17215=DIRECTION ( 'NONE',  ( 0.000000000000000000, -1.000000000000000000, 0.000000000000000000 ) ) ;
#17220=DIRECTION ( 'NONE',  ( -0.000000000000000000, 1.000000000000000000, 0.000000000000000000 ) ) ;
#17226=DIRECTION ( 'NONE',  ( 0.000000000000000000, 0.000000000000000000, -1.000000000000000000 ) ) ;
#17228=AXIS2_PLACEMENT_3D ( 'NONE', #67978, #76009, #31987 ) ;
#17231=CARTESIAN_POINT ( 'NONE',  ( 156.5250797092530206, 214.9970011440365454, 17.23862273017120117 ) ) ;
#17235=CARTESIAN_POINT ( 'NONE',  ( 209.2568086740256206, 34.98978593258856051, 12.00000000000000000 ) ) ;
#17245=TOROIDAL_SURFACE ( 'NONE', #61130, 4.499999999999990230, 0.5000000000000000000 ) ;
#17248=EDGE_CURVE ( 'NONE', #71446, #25460, #33894, .T. ) ;
#17252=AXIS2_PLACEMENT_3D ( 'NONE', #4859, #56477, #48398 ) ;
#17255=DIRECTION ( 'NONE',  ( -0.000000000000000000, -1.000000000000000000, -0.000000000000000000 ) ) ;
#17258=CARTESIAN_POINT ( 'NONE',  ( 155.0231696494769835, 19.71747416578156020, -13.29925684040344969 ) ) ;
#17278=CARTESIAN_POINT ( 'NONE',  ( 197.7051530045995094, 41.80213891112347824, 12.00000000000000000 ) ) ;
#17291=EDGE_CURVE ( 'NONE', #49791, #74853, #10653, .T. ) ;
#17308=AXIS2_PLACEMENT_3D ( 'NONE', #75229, #52046, #80930 ) ;
#17309=( BOUNDED_CURVE ( )  B_SPLINE_CURVE ( 3, ( #31440, #88247, #59870, #87313 ),
 .UNSPECIFIED., .F., .F. ) 
 B_SPLINE_CURVE_WITH_KNOTS ( ( 4, 4 ),
 ( 2.029441677703989200, 3.141592653589793116 ),
 .UNSPECIFIED. ) 
 CURVE ( )  GEOMETRIC_REPRESENTATION_ITEM ( )  RATIONAL_B_SPLINE_CURVE ( ( 1.000000000000000000, 0.8995554851227761661, 0.8995554851227761661, 1.000000000000000000 ) ) 
 REPRESENTATION_ITEM ( '' )  );
#17316=( BOUNDED_CURVE ( )  B_SPLINE_CURVE ( 3, ( #27493, #69177, #25605, #33653 ),
 .UNSPECIFIED., .F., .F. ) 
 B_SPLINE_CURVE_WITH_KNOTS ( ( 4, 4 ),
 ( 0.000000000000000000, 1.112150975885804360 ),
 .UNSPECIFIED. ) 
 CURVE ( )  GEOMETRIC_REPRESENTATION_ITEM ( )  RATIONAL_B_SPLINE_CURVE ( ( 1.000000000000000000, 0.8995554851227760551, 0.8995554851227760551, 1.000000000000000000 ) ) 
 REPRESENTATION_ITEM ( '' )  );
#17320=CIRCLE ( 'NONE', #30697, 4.999999999999993783 ) ;
#17327=AXIS2_PLACEMENT_3D ( 'NONE', #88982, #67702, #37406 ) ;
#17331=CARTESIAN_POINT ( 'NONE',  ( 185.4166944662832179, 249.5000000000000568, 23.37680765314684095 ) ) ;
#17344=CARTESIAN_POINT ( 'NONE',  ( 151.9231709899832197, 19.99481412879373821, 6.233581502755908943 ) ) ;
#17353=CARTESIAN_POINT ( 'NONE',  ( 175.2296996224750103, 158.6892791692949629, -24.00000000000001066 ) ) ;
#17361=EDGE_CURVE ( 'NONE', #49216, #4620, #18600, .T. ) ;
#17363=DIRECTION ( 'NONE',  ( 0.000000000000000000, 1.000000000000000000, 0.000000000000000000 ) ) ;
#17383=CIRCLE ( 'NONE', #27947, 7.999911143031724237 ) ;
#17385=EDGE_CURVE ( 'NONE', #19715, #23354, #68404, .T. ) ;
#17389=ORIENTED_EDGE ( 'NONE', *, *, #79781, .F. ) ;
#17392=DIRECTION ( 'NONE',  ( 0.000000000000000000, 0.000000000000000000, 1.000000000000000000 ) ) ;
#17400=AXIS2_PLACEMENT_3D ( 'NONE', #66682, #44426, #1809 ) ;
#17402=VERTEX_POINT ( 'NONE', #66391 ) ;
#17412=DIRECTION ( 'NONE',  ( 0.000000000000000000, 1.000000000000000000, 0.000000000000000000 ) ) ;
#17413=DIRECTION ( 'NONE',  ( -0.000000000000000000, -0.000000000000000000, 1.000000000000000000 ) ) ;
#17416=ORIENTED_EDGE ( 'NONE', *, *, #33617, .T. ) ;
#17430=CARTESIAN_POINT ( 'NONE',  ( 179.7289557593406357, 250.5000000000000568, -24.91818181818184641 ) ) ;
#17433=CARTESIAN_POINT ( 'NONE',  ( 139.1539576904058606, 275.5000000000000568, 10.50000000000000000 ) ) ;
#17442=CARTESIAN_POINT ( 'NONE',  ( 207.6662022560304024, 36.29800326561213808, 14.90057469441954119 ) ) ;
#17446=CARTESIAN_POINT ( 'NONE',  ( 196.7071296363291140, 19.50333209967902448, -12.79999999999991722 ) ) ;
#17448=EDGE_CURVE ( 'NONE', #68064, #74899, #8150, .T. ) ;
#17461=DIRECTION ( 'NONE',  ( -0.000000000000000000, -0.000000000000000000, -1.000000000000000000 ) ) ;
#17462=CARTESIAN_POINT ( 'NONE',  ( 185.8264795993290477, 214.9910457053126720, 23.09031830825835385 ) ) ;
#17475=FACE_OUTER_BOUND ( 'NONE', #12518, .T. ) ;
#17477=CARTESIAN_POINT ( 'NONE',  ( 195.7212220663432163, 20.45996914382524423, 12.49744573203606279 ) ) ;
#17486=FACE_OUTER_BOUND ( 'NONE', #25314, .T. ) ;
#17497=DIRECTION ( 'NONE',  ( -0.000000000000000000, -0.000000000000000000, -1.000000000000000000 ) ) ;
#17507=EDGE_CURVE ( 'NONE', #13368, #48925, #16962, .T. ) ;
#17509=ORIENTED_EDGE ( 'NONE', *, *, #43641, .F. ) ;
#17514=EDGE_CURVE ( 'NONE', #14181, #28861, #78734, .T. ) ;
#17516=CARTESIAN_POINT ( 'NONE',  ( 157.4970531492008661, 276.0000000000000568, 16.90571646082702983 ) ) ;
#17517=EDGE_LOOP ( 'NONE', ( #26631, #61006, #2763, #67395, #61105, #14033, #29296 ) ) ;
#17520=CARTESIAN_POINT ( 'NONE',  ( 204.6539576904058606, 287.9062406767683910, 3.999999999999991562 ) ) ;
#17521=DIRECTION ( 'NONE',  ( 0.000000000000000000, 0.000000000000000000, 1.000000000000000000 ) ) ;
#17544=CARTESIAN_POINT ( 'NONE',  ( 165.7865175155837676, 3.000000000000000000, -9.000000000000001776 ) ) ;
#17555=EDGE_LOOP ( 'NONE', ( #44898, #18549, #33954, #20594 ) ) ;
#17563=B_SPLINE_CURVE_WITH_KNOTS ( 'NONE', 3,
 ( #91433, #76776, #92364, #27526, #39822, #11903, #62589, #20429 ),
 .UNSPECIFIED., .F., .F.,
 ( 4, 2, 2, 4 ),
 ( 4.336808689942017736E-19, 0.004152702846877201481, 0.006229054270315790079, 0.008305405693754378676 ),
 .UNSPECIFIED. ) ;
#17570=EDGE_CURVE ( 'NONE', #50020, #14856, #86341, .T. ) ;
#17571=EDGE_CURVE ( 'NONE', #77857, #31, #27591, .T. ) ;
#17580=CARTESIAN_POINT ( 'NONE',  ( 194.4805735913283229, 26.12542652888812356, 14.33214477299284795 ) ) ;
#17589=CARTESIAN_POINT ( 'NONE',  ( 197.9510393857643180, 24.58358384448226630, 11.14414497126373860 ) ) ;
#17592=DIRECTION ( 'NONE',  ( -0.000000000000000000, -1.000000000000000000, -0.000000000000000000 ) ) ;
#17593=DIRECTION ( 'NONE',  ( -0.000000000000000000, 1.000000000000000000, -0.000000000000000000 ) ) ;
#17602=EDGE_LOOP ( 'NONE', ( #44775, #13136, #57697 ) ) ;
#17606=CARTESIAN_POINT ( 'NONE',  ( 197.2116943569230330, 275.0000000000000568, -12.42446933126074882 ) ) ;
#17617=CARTESIAN_POINT ( 'NONE',  ( 159.2635086430408080, 16.19322481500758215, 10.13850573484278783 ) ) ;
#17620=DIRECTION ( 'NONE',  ( -0.000000000000000000, -0.000000000000000000, 1.000000000000000000 ) ) ;
#17632=EDGE_CURVE ( 'NONE', #23012, #9431, #50213, .T. ) ;
#17638=ORIENTED_EDGE ( 'NONE', *, *, #39759, .T. ) ;
#17649=VERTEX_POINT ( 'NONE', #29482 ) ;
#17660=ORIENTED_EDGE ( 'NONE', *, *, #291, .T. ) ;
#17667=ORIENTED_EDGE ( 'NONE', *, *, #54326, .F. ) ;
#17668=CARTESIAN_POINT ( 'NONE',  ( 139.6539576904058606, 132.0000000000000568, -10.49999999999999822 ) ) ;
#17672=ORIENTED_EDGE ( 'NONE', *, *, #6263, .F. ) ;
#17677=ADVANCED_FACE ( 'NONE', ( #93395 ), #60842, .T. ) ;
#17686=EDGE_CURVE ( 'NONE', #16590, #63583, #35149, .T. ) ;
#17688=EDGE_CURVE ( 'NONE', #59928, #3752, #18439, .T. ) ;
#17690=CARTESIAN_POINT ( 'NONE',  ( 206.6110850237746490, 1.019348808636641568, -7.290232558141295449 ) ) ;
#17695=CARTESIAN_POINT ( 'NONE',  ( 209.3504981911156335, 1.050453206927881578, 7.446924052135294403 ) ) ;
#17696=CARTESIAN_POINT ( 'NONE',  ( 156.4217629211117355, 119.0463968525363327, 7.000000000000000000 ) ) ;
#17699=PLANE ( 'NONE',  #30210 ) ;
#17701=CARTESIAN_POINT ( 'NONE',  ( 200.4871970924806419, 61.71654497095076408, 9.999999999999998224 ) ) ;
#17718=FACE_OUTER_BOUND ( 'NONE', #70423, .T. ) ;
#17720=ORIENTED_EDGE ( 'NONE', *, *, #60067, .F. ) ;
#17722=CARTESIAN_POINT ( 'NONE',  ( 197.3534831049100831, 70.40830473911788090, 11.81087581402289466 ) ) ;
#17751=ORIENTED_EDGE ( 'NONE', *, *, #67910, .T. ) ;
#17753=VERTEX_POINT ( 'NONE', #29007 ) ;
#17769=VERTEX_POINT ( 'NONE', #72560 ) ;
#17774=EDGE_LOOP ( 'NONE', ( #964, #51053, #54340, #34403 ) ) ;
#17776=ADVANCED_FACE ( 'NONE', ( #51231 ), #36636, .T. ) ;
#17782=ADVANCED_FACE ( 'NONE', ( #32255 ), #38099, .T. ) ;
#17788=LINE ( 'NONE', #3576, #29340 ) ;
#17801=CARTESIAN_POINT ( 'NONE',  ( 201.2104617360081704, 25.32700003806615996, 10.00000000000000000 ) ) ;
#17809=CARTESIAN_POINT ( 'NONE',  ( 197.4288403404171959, 41.88980437486001307, 11.72798125285450332 ) ) ;
#17821=ORIENTED_EDGE ( 'NONE', *, *, #291, .F. ) ;
#17827=EDGE_CURVE ( 'NONE', #26935, #52628, #88604, .T. ) ;
#17845=ORIENTED_EDGE ( 'NONE', *, *, #17507, .T. ) ;
#17848=CARTESIAN_POINT ( 'NONE',  ( 208.8901450372919442, 29.13786557026924839, 13.14640446942321539 ) ) ;
#17859=FACE_OUTER_BOUND ( 'NONE', #80476, .T. ) ;
#17873=VERTEX_POINT ( 'NONE', #23752 ) ;
#17882=ORIENTED_EDGE ( 'NONE', *, *, #17917, .T. ) ;
#17890=ADVANCED_FACE ( 'NONE', ( #75344 ), #20364, .F. ) ;
#17891=CARTESIAN_POINT ( 'NONE',  ( 180.2835393005426283, 214.8829713991971744, -24.64732457002850552 ) ) ;
#17900=CARTESIAN_POINT ( 'NONE',  ( 138.6539576904058606, 132.0000000000000568, 12.50000000000000000 ) ) ;
#17902=ORIENTED_EDGE ( 'NONE', *, *, #41688, .T. ) ;
#17903=CARTESIAN_POINT ( 'NONE',  ( 199.3270723581583468, 16.88338937786772931, 10.34008960743410377 ) ) ;
#17906=EDGE_CURVE ( 'NONE', #60755, #75996, #91005, .T. ) ;
#17911=VECTOR ( 'NONE', #55668, 1000.000000000000000 ) ;
#17917=EDGE_CURVE ( 'NONE', #70030, #36590, #12928, .T. ) ;
#17934=CARTESIAN_POINT ( 'NONE',  ( 192.9182251362765328, 250.0000000000000568, 16.22085278731030300 ) ) ;
#17953=ORIENTED_EDGE ( 'NONE', *, *, #5504, .F. ) ;
#17954=CYLINDRICAL_SURFACE ( 'NONE', #37823, 2.999999999999993783 ) ;
#17956=CYLINDRICAL_SURFACE ( 'NONE', #36783, 4.999999999999978684 ) ;
#17964=ORIENTED_EDGE ( 'NONE', *, *, #18823, .F. ) ;
#17971=CARTESIAN_POINT ( 'NONE',  ( 156.8041522122653646, 275.5797763526087465, 16.89672165344857646 ) ) ;
#17973=CIRCLE ( 'NONE', #70910, 2.842139515347646750 ) ;
#17985=VERTEX_POINT ( 'NONE', #30393 ) ;
#17993=ADVANCED_FACE ( 'NONE', ( #31332 ), #26004, .F. ) ;
#18002=DIRECTION ( 'NONE',  ( 0.000000000000000000, 1.000000000000000000, 0.000000000000000000 ) ) ;
#18018=EDGE_CURVE ( 'NONE', #79410, #34882, #30550, .T. ) ;
#18023=CARTESIAN_POINT ( 'NONE',  ( 209.7064572754727010, 36.40703279031868789, 14.69807322781338854 ) ) ;
#18035=CARTESIAN_POINT ( 'NONE',  ( 152.4536156746142410, 249.5000000000000568, -12.50000000000000000 ) ) ;
#18037=CONICAL_SURFACE ( 'NONE', #33170, 24.00000000000001066, 0.7853981633974361776 ) ;
#18038=CARTESIAN_POINT ( 'NONE',  ( 208.8930925782355530, 0.04008605884692667543, 7.489252814170929362 ) ) ;
#18045=CARTESIAN_POINT ( 'NONE',  ( 152.4536156746142410, 129.7208004331680797, -12.50000000000000000 ) ) ;
#18047=CARTESIAN_POINT ( 'NONE',  ( 0.000000000000000000, 15.00000000000000000, 15.00000000000000000 ) ) ;
#18049=DIRECTION ( 'NONE',  ( 0.000000000000000000, 1.000000000000000000, 0.000000000000000000 ) ) ;
#18061=DIRECTION ( 'NONE',  ( 0.000000000000000000, 1.000000000000000000, 0.000000000000000000 ) ) ;
#18064=DIRECTION ( 'NONE',  ( 0.000000000000000000, 0.000000000000000000, 1.000000000000000000 ) ) ;
#18075=CARTESIAN_POINT ( 'NONE',  ( 156.2095471516454950, 16.65459343288105742, 7.440913067426849992 ) ) ;
#18090=ORIENTED_EDGE ( 'NONE', *, *, #16334, .T. ) ;
#18104=EDGE_LOOP ( 'NONE', ( #62633, #43175, #23249, #18216 ) ) ;
#18107=AXIS2_PLACEMENT_3D ( 'NONE', #47010, #18621, #46551 ) ;
#18112=DIRECTION ( 'NONE',  ( 0.000000000000000000, 0.000000000000000000, 1.000000000000000000 ) ) ;
#18117=ORIENTED_EDGE ( 'NONE', *, *, #84467, .F. ) ;
#18135=DIRECTION ( 'NONE',  ( 0.000000000000000000, 1.000000000000000000, 0.000000000000000000 ) ) ;
#18146=CARTESIAN_POINT ( 'NONE',  ( 204.6539576904058606, 293.9636489450775230, 7.999911143031724237 ) ) ;
#18149=ADVANCED_FACE ( 'NONE', ( #74889 ), #24686, .F. ) ;
#18152=CARTESIAN_POINT ( 'NONE',  ( 210.2502813974796538, 1.019348808636640458, 7.290232558141290120 ) ) ;
#18153=DIRECTION ( 'NONE',  ( 0.9452808130703180822, -1.131934301928085161E-15, -0.3262578496237575343 ) ) ;
#18156=CARTESIAN_POINT ( 'NONE',  ( 209.7513585654923816, 282.2246705312486483, 13.99999999999999112 ) ) ;
#18159=CARTESIAN_POINT ( 'NONE',  ( 156.4851178187871312, 15.00000000000000178, -7.000000000000000888 ) ) ;
#18161=DIRECTION ( 'NONE',  ( -1.110223024625156146E-15, 0.000000000000000000, 1.000000000000000000 ) ) ;
#18173=CIRCLE ( 'NONE', #62043, 1.999999999999988454 ) ;
#18175=ORIENTED_EDGE ( 'NONE', *, *, #82436, .T. ) ;
#18177=AXIS2_PLACEMENT_3D ( 'NONE', #78572, #78113, #64865 ) ;
#18198=CARTESIAN_POINT ( 'NONE',  ( 188.7149167944524493, 8.542400036368780647, -9.000000000000001776 ) ) ;
#18216=ORIENTED_EDGE ( 'NONE', *, *, #5917, .T. ) ;
#18238=EDGE_LOOP ( 'NONE', ( #8585, #89004, #88207, #7750, #55105, #35384 ) ) ;
#18245=CARTESIAN_POINT ( 'NONE',  ( 175.2296996224750103, 250.0000000000000568, 0.000000000000000000 ) ) ;
#18257=CARTESIAN_POINT ( 'NONE',  ( 153.2628468892384319, 20.37991841447902530, -11.93555113919326693 ) ) ;
#18262=DIRECTION ( 'NONE',  ( 1.000000000000000000, 0.000000000000000000, 0.000000000000000000 ) ) ;
#18266=DIRECTION ( 'NONE',  ( -0.000000000000000000, -0.000000000000000000, 1.000000000000000000 ) ) ;
#18269=CARTESIAN_POINT ( 'NONE',  ( 185.4166944662832179, 249.5000000000000568, 22.87680765314684095 ) ) ;
#18270=DIRECTION ( 'NONE',  ( 1.000000000000000000, 0.000000000000000000, 0.000000000000000000 ) ) ;
#18285=DIRECTION ( 'NONE',  ( 0.000000000000000000, 1.000000000000000000, 0.000000000000000000 ) ) ;
#18288=CARTESIAN_POINT ( 'NONE',  ( 140.6539576904058606, 250.5000000000000568, 12.00000000000000000 ) ) ;
#18304=CARTESIAN_POINT ( 'NONE',  ( 209.2251716680733580, 29.17473719793202847, 13.08022668053246385 ) ) ;
#18305=AXIS2_PLACEMENT_3D ( 'NONE', #9560, #9087, #60251 ) ;
#18317=ORIENTED_EDGE ( 'NONE', *, *, #17688, .T. ) ;
#18336=B_SPLINE_CURVE_WITH_KNOTS ( 'NONE', 3,
 ( #30186, #52421, #87918, #7474, #43460, #23069, #51947, #74198 ),
 .UNSPECIFIED., .F., .F.,
 ( 4, 2, 2, 4 ),
 ( 0.000000000000000000, 0.004220890787215657823, 0.006331336180823474158, 0.008441781574431289625 ),
 .UNSPECIFIED. ) ;
#18341=EDGE_LOOP ( 'NONE', ( #58411, #43498, #17821, #33436 ) ) ;
#18349=DIRECTION ( 'NONE',  ( 0.000000000000000000, -0.000000000000000000, 1.000000000000000000 ) ) ;
#18350=CARTESIAN_POINT ( 'NONE',  ( 196.3886764727502054, 69.83403101108301314, 15.08154681515735440 ) ) ;
#18360=EDGE_LOOP ( 'NONE', ( #51758, #45305, #36181, #89373, #22755, #67260 ) ) ;
#18361=CARTESIAN_POINT ( 'NONE',  ( 198.3325868694606129, 18.45344983985999576, 10.88803913699904058 ) ) ;
#18390=CARTESIAN_POINT ( 'NONE',  ( 175.2296996224750103, 246.0000000000001137, 9.550761578869391144 ) ) ;
#18411=CARTESIAN_POINT ( 'NONE',  ( 205.7381008070598227, 0.000000000000000000, -7.000000000000000888 ) ) ;
#18424=CARTESIAN_POINT ( 'NONE',  ( 197.0359635097977389, 71.72764050497774235, -10.24344765926147893 ) ) ;
#18428=EDGE_LOOP ( 'NONE', ( #18645, #81540, #84775, #63444 ) ) ;
#18431=LINE ( 'NONE', #12270, #89616 ) ;
#18432=CIRCLE ( 'NONE', #24447, 1.000000000000000000 ) ;
#18433=CARTESIAN_POINT ( 'NONE',  ( 195.9492931686500583, 25.28061950067115404, 13.99099524138373418 ) ) ;
#18439=CIRCLE ( 'NONE', #9375, 0.9999999999999977796 ) ;
#18442=EDGE_CURVE ( 'NONE', #60346, #70318, #88042, .T. ) ;
#18457=CARTESIAN_POINT ( 'NONE',  ( 164.7123623445222904, 3.000000000000000000, -9.000000000000001776 ) ) ;
#18468=ORIENTED_EDGE ( 'NONE', *, *, #44642, .F. ) ;
#18469=CARTESIAN_POINT ( 'NONE',  ( 158.6539576904058606, 293.9636489450775230, 9.103929867429224387 ) ) ;
#18477=DIRECTION ( 'NONE',  ( 1.000000000000000000, 0.000000000000000000, 0.000000000000000000 ) ) ;
#18491=AXIS2_PLACEMENT_3D ( 'NONE', #43749, #1146, #8244 ) ;
#18499=AXIS2_PLACEMENT_3D ( 'NONE', #2212, #30616, #60906 ) ;
#18501=CARTESIAN_POINT ( 'NONE',  ( 165.2688068684385883, 275.0000000000000568, 21.83530662808711398 ) ) ;
#18506=CARTESIAN_POINT ( 'NONE',  ( 160.5350683151633291, 250.5000000000000568, 20.22542485937379908 ) ) ;
#18516=EDGE_CURVE ( 'NONE', #78809, #49098, #81957, .T. ) ;
#18519=CARTESIAN_POINT ( 'NONE',  ( 175.2296996224750103, 149.6461846693799487, 0.000000000000000000 ) ) ;
#18535=CARTESIAN_POINT ( 'NONE',  ( 139.6539576904058606, 132.0000000000000568, 12.50000000000000000 ) ) ;
#18549=ORIENTED_EDGE ( 'NONE', *, *, #73250, .T. ) ;
#18551=VERTEX_POINT ( 'NONE', #78166 ) ;
#18555=EDGE_CURVE ( 'NONE', #27314, #15179, #70130, .T. ) ;
#18562=ORIENTED_EDGE ( 'NONE', *, *, #56142, .T. ) ;
#18563=VECTOR ( 'NONE', #55539, 1000.000000000000000 ) ;
#18566=AXIS2_PLACEMENT_3D ( 'NONE', #91481, #12420, #70209 ) ;
#18572=AXIS2_PLACEMENT_3D ( 'NONE', #52616, #60220, #600 ) ;
#18577=ORIENTED_EDGE ( 'NONE', *, *, #34294, .F. ) ;
#18586=DIRECTION ( 'NONE',  ( 0.000000000000000000, 1.000000000000000000, 0.000000000000000000 ) ) ;
#18591=ORIENTED_EDGE ( 'NONE', *, *, #88682, .T. ) ;
#18598=CARTESIAN_POINT ( 'NONE',  ( 155.3778607292159961, 21.00000000000000000, 15.20506116941399277 ) ) ;
#18600=B_SPLINE_CURVE_WITH_KNOTS ( 'NONE', 3,
 ( #46211, #21910, #87667, #43665, #80119, #49837, #36567, #22817 ),
 .UNSPECIFIED., .F., .F.,
 ( 4, 2, 2, 4 ),
 ( 0.000000000000000000, 0.0004362529587405823499, 0.0008725059174811646999, 0.001745011834962329400 ),
 .UNSPECIFIED. ) ;
#18611=PLANE ( 'NONE',  #12787 ) ;
#18618=FACE_OUTER_BOUND ( 'NONE', #12059, .T. ) ;
#18621=DIRECTION ( 'NONE',  ( 0.000000000000000000, -0.000000000000000000, 1.000000000000000000 ) ) ;
#18624=CARTESIAN_POINT ( 'NONE',  ( 156.2095471516448413, 16.65459343288320682, -7.440913067427157301 ) ) ;
#18626=CARTESIAN_POINT ( 'NONE',  ( 206.6398282674434483, 29.68967932838811663, 13.90950695095619771 ) ) ;
#18629=CARTESIAN_POINT ( 'NONE',  ( 157.1249521815083483, 17.17215575532036453, -9.360165637272727324 ) ) ;
#18640=AXIS2_PLACEMENT_3D ( 'NONE', #87630, #36527, #89 ) ;
#18645=ORIENTED_EDGE ( 'NONE', *, *, #24497, .F. ) ;
#18650=AXIS2_PLACEMENT_3D ( 'NONE', #61297, #39934, #10600 ) ;
#18678=ADVANCED_FACE ( 'NONE', ( #85253 ), #15471, .F. ) ;
#18680=ORIENTED_EDGE ( 'NONE', *, *, #32302, .T. ) ;
#18686=EDGE_CURVE ( 'NONE', #56456, #53974, #17316, .T. ) ;
#18705=EDGE_LOOP ( 'NONE', ( #38783, #28105, #56712, #32557 ) ) ;
#18708=EDGE_LOOP ( 'NONE', ( #40335, #8615, #61420, #89935 ) ) ;
#18710=CIRCLE ( 'NONE', #71658, 7.910944475430059519 ) ;
#18716=FACE_OUTER_BOUND ( 'NONE', #67744, .T. ) ;
#18718=CIRCLE ( 'NONE', #30825, 1.500000000000003997 ) ;
#18721=FACE_BOUND ( 'NONE', #88914, .T. ) ;
#18724=VECTOR ( 'NONE', #42905, 1000.000000000000000 ) ;
#18733=AXIS2_PLACEMENT_3D ( 'NONE', #32125, #54819, #77077 ) ;
#18737=EDGE_CURVE ( 'NONE', #69962, #62086, #26483, .T. ) ;
#18738=EDGE_CURVE ( 'NONE', #79497, #45087, #4868, .T. ) ;
#18739=CARTESIAN_POINT ( 'NONE',  ( 197.2081551558208048, 68.08088840871901937, 10.51999689724803311 ) ) ;
#18742=AXIS2_PLACEMENT_3D ( 'NONE', #93644, #28342, #57232 ) ;
#18745=CARTESIAN_POINT ( 'NONE',  ( 152.4536156746142410, 276.0000000000000568, -14.50000000000000000 ) ) ;
#18749=DIRECTION ( 'NONE',  ( 0.7957555401921962979, 0.6056179655966504871, 0.000000000000000000 ) ) ;
#18754=CARTESIAN_POINT ( 'NONE',  ( 186.6539576904058890, 276.0000000000000568, -11.60392986742922439 ) ) ;
#18767=DIRECTION ( 'NONE',  ( 0.000000000000000000, 0.000000000000000000, -1.000000000000000000 ) ) ;
#18780=ORIENTED_EDGE ( 'NONE', *, *, #34635, .T. ) ;
#18782=CIRCLE ( 'NONE', #62674, 24.00000000000000355 ) ;
#18784=DIRECTION ( 'NONE',  ( 0.000000000000000000, 1.000000000000000000, 0.000000000000000000 ) ) ;
#18796=ORIENTED_EDGE ( 'NONE', *, *, #92268, .T. ) ;
#18807=CARTESIAN_POINT ( 'NONE',  ( 219.8344101925596021, 35.72494958537217968, 9.000000000000001776 ) ) ;
#18809=DIRECTION ( 'NONE',  ( -0.000000000000000000, -1.000000000000000000, -0.000000000000000000 ) ) ;
#18823=EDGE_CURVE ( 'NONE', #64042, #13568, #12443, .T. ) ;
#18824=ORIENTED_EDGE ( 'NONE', *, *, #90373, .F. ) ;
#18841=CARTESIAN_POINT ( 'NONE',  ( 195.6084660501286692, 42.25382305297375041, 12.67848964989311611 ) ) ;
#18858=CARTESIAN_POINT ( 'NONE',  ( 189.9243309297870610, 276.0000000000000568, 20.22542485937349355 ) ) ;
#18859=EDGE_CURVE ( 'NONE', #34447, #8082, #86565, .T. ) ;
#18860=CARTESIAN_POINT ( 'NONE',  ( 196.2494062209129027, 40.89692782860188913, 13.06344435505938861 ) ) ;
#18871=VECTOR ( 'NONE', #8555, 1000.000000000000000 ) ;
#18880=CIRCLE ( 'NONE', #91651, 24.50000000000000355 ) ;
#18883=TOROIDAL_SURFACE ( 'NONE', #71832, 24.49999999999999645, 0.5000000000000000000 ) ;
#18885=CARTESIAN_POINT ( 'NONE',  ( 195.2312239546291437, 39.36132622696000283, 15.00000000000000000 ) ) ;
#18893=ORIENTED_EDGE ( 'NONE', *, *, #58679, .T. ) ;
#18894=DIRECTION ( 'NONE',  ( 0.6056179655966488218, -0.7957555401921976301, 0.000000000000000000 ) ) ;
#18896=DIRECTION ( 'NONE',  ( 1.000000000000000000, -0.000000000000000000, -0.000000000000000000 ) ) ;
#18916=CARTESIAN_POINT ( 'NONE',  ( 197.4878715644970555, 25.93102243561465414, 12.00000000000000000 ) ) ;
#18917=DIRECTION ( 'NONE',  ( 1.000000000000000000, 0.000000000000000000, 0.000000000000000000 ) ) ;
#18935=EDGE_LOOP ( 'NONE', ( #11356, #72469, #85648, #15340 ) ) ;
#18936=LINE ( 'NONE', #82845, #65058 ) ;
#18940=AXIS2_PLACEMENT_3D ( 'NONE', #90959, #40773, #33703 ) ;
#18949=CIRCLE ( 'NONE', #15914, 0.4999999999999922839 ) ;
#18954=CARTESIAN_POINT ( 'NONE',  ( 157.7238125175271648, 18.72892514816273746, -11.10081581328746658 ) ) ;
#18958=EDGE_CURVE ( 'NONE', #17649, #1470, #47369, .T. ) ;
#18976=EDGE_CURVE ( 'NONE', #9610, #66586, #59424, .T. ) ;
#18978=CARTESIAN_POINT ( 'NONE',  ( 200.2296996224750103, 68.12454877777268791, 0.000000000000000000 ) ) ;
#18988=CARTESIAN_POINT ( 'NONE',  ( 152.8344704311132602, 129.4968913933752503, -12.52864452723162003 ) ) ;
#18990=CARTESIAN_POINT ( 'NONE',  ( 197.2116943569230330, 275.5000000000000568, -12.92446933126074882 ) ) ;
#18992=DIRECTION ( 'NONE',  ( -1.000000000000000000, 0.000000000000000000, 0.000000000000000000 ) ) ;
#19003=DIRECTION ( 'NONE',  ( 0.000000000000000000, 0.000000000000000000, -1.000000000000000000 ) ) ;
#19019=LINE ( 'NONE', #18535, #8770 ) ;
#19033=VERTEX_POINT ( 'NONE', #11874 ) ;
#19040=CARTESIAN_POINT ( 'NONE',  ( 194.7453183674700199, 20.99999999999999645, -15.62499999999999112 ) ) ;
#19052=CARTESIAN_POINT ( 'NONE',  ( 200.4644824113734671, 275.5000000000000568, -2.942835885954290021 ) ) ;
#19065=EDGE_LOOP ( 'NONE', ( #32265, #90845, #27665, #39578 ) ) ;
#19070=ORIENTED_EDGE ( 'NONE', *, *, #85278, .F. ) ;
#19071=ADVANCED_FACE ( 'NONE', ( #21324 ), #62400, .T. ) ;
#19078=CARTESIAN_POINT ( 'NONE',  ( 199.5417009657504650, 26.45151344826108897, 10.49999999999999645 ) ) ;
#19087=AXIS2_PLACEMENT_3D ( 'NONE', #32553, #38696, #32069 ) ;
#19092=EDGE_CURVE ( 'NONE', #13829, #67504, #44253, .T. ) ;
#19103=CARTESIAN_POINT ( 'NONE',  ( 207.5863589332323329, 29.28491128719180026, 13.57731244650625513 ) ) ;
#19115=EDGE_LOOP ( 'NONE', ( #13220, #39488, #26158, #13808 ) ) ;
#19118=CARTESIAN_POINT ( 'NONE',  ( 206.8376799756172204, 36.39179024836181497, 13.90950695095621015 ) ) ;
#19136=DIRECTION ( 'NONE',  ( 0.000000000000000000, 0.000000000000000000, 1.000000000000000000 ) ) ;
#19143=CARTESIAN_POINT ( 'NONE',  ( 209.5027106082920056, 29.50523358103493621, 14.69807322781335479 ) ) ;
#19150=ORIENTED_EDGE ( 'NONE', *, *, #47379, .F. ) ;
#19155=EDGE_CURVE ( 'NONE', #65802, #26035, #36698, .T. ) ;
#19174=ORIENTED_EDGE ( 'NONE', *, *, #63351, .T. ) ;
#19182=CARTESIAN_POINT ( 'NONE',  ( 209.7513585654922679, 305.7026273589066818, -40.00000000000000711 ) ) ;
#19187=CARTESIAN_POINT ( 'NONE',  ( 160.5350683151633291, 275.0000000000000568, 20.22542485937379908 ) ) ;
#19195=CARTESIAN_POINT ( 'NONE',  ( 153.8597781956983113, 19.40377396060713266, -11.71176238812795134 ) ) ;
#19200=CARTESIAN_POINT ( 'NONE',  ( 140.6539576904058606, 130.0000000000000568, -12.50000000000000000 ) ) ;
#19203=EDGE_CURVE ( 'NONE', #91332, #93704, #7129, .T. ) ;
#19205=FACE_OUTER_BOUND ( 'NONE', #69708, .T. ) ;
#19208=CARTESIAN_POINT ( 'NONE',  ( 197.1656530321902494, 41.90019538913895758, 12.64285714285713169 ) ) ;
#19209=CARTESIAN_POINT ( 'NONE',  ( 197.2304840627181477, 41.97094794048064870, 11.95796701298976572 ) ) ;
#19215=CARTESIAN_POINT ( 'NONE',  ( 152.6878565075764413, 20.88255170682893080, -8.268021619243398845 ) ) ;
#19223=DIRECTION ( 'NONE',  ( 0.000000000000000000, 0.000000000000000000, 1.000000000000000000 ) ) ;
#19247=FACE_OUTER_BOUND ( 'NONE', #50322, .T. ) ;
#19257=ORIENTED_EDGE ( 'NONE', *, *, #18859, .F. ) ;
#19267=CARTESIAN_POINT ( 'NONE',  ( 175.2296996224750103, 20.99999999999998934, 0.000000000000000000 ) ) ;
#19268=CARTESIAN_POINT ( 'NONE',  ( 151.2975037349263800, 130.0000000000000568, 12.50000000000000000 ) ) ;
#19272=ORIENTED_EDGE ( 'NONE', *, *, #31803, .F. ) ;
#19281=EDGE_LOOP ( 'NONE', ( #22757, #40417, #70408, #8547 ) ) ;
#19286=DIRECTION ( 'NONE',  ( 1.000000000000000000, 0.000000000000000000, -0.000000000000000000 ) ) ;
#19295=DIRECTION ( 'NONE',  ( 0.6056179655966478226, -0.7957555401921982963, -0.000000000000000000 ) ) ;
#19297=LINE ( 'NONE', #17900, #33505 ) ;
#19299=ORIENTED_EDGE ( 'NONE', *, *, #85804, .F. ) ;
#19300=CARTESIAN_POINT ( 'NONE',  ( 200.3378311594553622, 16.04715669186171922, 10.05743975622762498 ) ) ;
#19315=CARTESIAN_POINT ( 'NONE',  ( 154.0637704119390037, 19.72112694978656577, -13.30738029212319162 ) ) ;
#19339=CARTESIAN_POINT ( 'NONE',  ( 196.9624057960931509, 41.89407144457039323, 12.94963709701906751 ) ) ;
#19348=CARTESIAN_POINT ( 'NONE',  ( 201.2509219215139922, 65.09645894978946501, 0.000000000000000000 ) ) ;
#19361=DIRECTION ( 'NONE',  ( 0.000000000000000000, 0.000000000000000000, 1.000000000000000000 ) ) ;
#19365=CARTESIAN_POINT ( 'NONE',  ( 199.2296996224018812, 66.10105075032893751, -2.340466192624005792 ) ) ;
#19371=CARTESIAN_POINT ( 'NONE',  ( 204.6539576904058606, 291.1800221208779931, -7.500000000000000000 ) ) ;
#19372=CYLINDRICAL_SURFACE ( 'NONE', #25030, 2.000000000000000000 ) ;
#19373=CARTESIAN_POINT ( 'NONE',  ( 197.2116943569230045, 249.5000000000000568, -12.42446933126075592 ) ) ;
#19377=ADVANCED_FACE ( 'NONE', ( #79098 ), #26989, .T. ) ;
#19380=EDGE_CURVE ( 'NONE', #67504, #13829, #71466, .T. ) ;
#19395=VERTEX_POINT ( 'NONE', #49730 ) ;
#19396=AXIS2_PLACEMENT_3D ( 'NONE', #21830, #50223, #79127 ) ;
#19419=B_SPLINE_CURVE_WITH_KNOTS ( 'NONE', 3,
 ( #40560, #83665, #40102, #55282 ),
 .UNSPECIFIED., .F., .F.,
 ( 4, 4 ),
 ( -4.472146915501929662E-06, 0.0002823611672359634833 ),
 .UNSPECIFIED. ) ;
#19446=CARTESIAN_POINT ( 'NONE',  ( 203.6821298523975088, 287.7126147091306620, -4.992670775290489971 ) ) ;
#19459=VERTEX_POINT ( 'NONE', #33490 ) ;
#19473=DIRECTION ( 'NONE',  ( 0.000000000000000000, 0.000000000000000000, 1.000000000000000000 ) ) ;
#19474=CARTESIAN_POINT ( 'NONE',  ( 160.5350683151633291, 215.0000000000000568, 25.22542485937379197 ) ) ;
#19481=EDGE_CURVE ( 'NONE', #15179, #56456, #30608, .T. ) ;
#19489=ORIENTED_EDGE ( 'NONE', *, *, #5821, .T. ) ;
#19491=EDGE_LOOP ( 'NONE', ( #51142, #74444, #26389, #9344 ) ) ;
#19500=VERTEX_POINT ( 'NONE', #48624 ) ;
#19507=DIRECTION ( 'NONE',  ( 0.000000000000000000, 1.000000000000000000, 0.000000000000000000 ) ) ;
#19520=DIRECTION ( 'NONE',  ( 0.9167375550253826777, 5.544037366339495023E-15, 0.3994899938747948354 ) ) ;
#19526=CIRCLE ( 'NONE', #28604, 4.999999999999990230 ) ;
#19532=CYLINDRICAL_SURFACE ( 'NONE', #17252, 2.500000000000002220 ) ;
#19537=CARTESIAN_POINT ( 'NONE',  ( 207.9918764980109813, 30.19551755111683633, 15.05517478741770532 ) ) ;
#19548=DIRECTION ( 'NONE',  ( -0.2456588035076310295, 0.9693563597868428694, 0.000000000000000000 ) ) ;
#19549=CYLINDRICAL_SURFACE ( 'NONE', #47351, 1.999999999999996003 ) ;
#19554=CARTESIAN_POINT ( 'NONE',  ( 193.6552470326849402, 250.5000000000000568, 16.89672165344822119 ) ) ;
#19556=CARTESIAN_POINT ( 'NONE',  ( 208.3418117619747818, 38.42745601219717599, 11.99999999999999822 ) ) ;
#19571=VERTEX_POINT ( 'NONE', #61921 ) ;
#19578=DIRECTION ( 'NONE',  ( 0.000000000000000000, 0.000000000000000000, 1.000000000000000000 ) ) ;
#19590=EDGE_CURVE ( 'NONE', #78809, #200, #42457, .T. ) ;
#19609=ORIENTED_EDGE ( 'NONE', *, *, #77208, .T. ) ;
#19612=EDGE_LOOP ( 'NONE', ( #67245, #6383, #77532, #48990 ) ) ;
#19615=EDGE_CURVE ( 'NONE', #17985, #89903, #91071, .T. ) ;
#19644=DIRECTION ( 'NONE',  ( 0.000000000000000000, 0.000000000000000000, 1.000000000000000000 ) ) ;
#19656=FACE_OUTER_BOUND ( 'NONE', #47790, .T. ) ;
#19659=VECTOR ( 'NONE', #27927, 1000.000000000000000 ) ;
#19662=CARTESIAN_POINT ( 'NONE',  ( 196.3789471156757713, 71.92880008233049693, 11.42127566691390683 ) ) ;
#19666=CARTESIAN_POINT ( 'NONE',  ( 198.1329898669366969, 69.92583464099143953, 8.330337636095686449 ) ) ;
#19669=CARTESIAN_POINT ( 'NONE',  ( 195.4781563537916043, 39.36132622696000283, 15.00000000000000000 ) ) ;
#19673=EDGE_CURVE ( 'NONE', #4825, #65856, #7967, .T. ) ;
#19686=CARTESIAN_POINT ( 'NONE',  ( 200.4738562182569694, 293.9636489450776367, -44.00000000000000000 ) ) ;
#19699=EDGE_CURVE ( 'NONE', #33474, #34201, #91715, .T. ) ;
#19714=VERTEX_POINT ( 'NONE', #26868 ) ;
#19715=VERTEX_POINT ( 'NONE', #49112 ) ;
#19724=AXIS2_PLACEMENT_3D ( 'NONE', #25062, #24581, #53469 ) ;
#19730=AXIS2_PLACEMENT_3D ( 'NONE', #46573, #17255, #75017 ) ;
#19733=VERTEX_POINT ( 'NONE', #71368 ) ;
#19746=ORIENTED_EDGE ( 'NONE', *, *, #67912, .F. ) ;
#19748=CARTESIAN_POINT ( 'NONE',  ( 152.4536156746142410, 0.000000000000000000, -12.50000000000000000 ) ) ;
#19750=EDGE_CURVE ( 'NONE', #30016, #53974, #10520, .T. ) ;
#19757=CARTESIAN_POINT ( 'NONE',  ( 175.2296996224750103, 142.2541816238762920, -24.00000000000001066 ) ) ;
#19759=CARTESIAN_POINT ( 'NONE',  ( 194.3811518219889649, 40.34787838408796290, 14.46471776229852679 ) ) ;
#19777=FACE_OUTER_BOUND ( 'NONE', #4816, .T. ) ;
#19778=CARTESIAN_POINT ( 'NONE',  ( 195.9119638496091227, 40.72287714413864990, 13.40410220951428855 ) ) ;
#19780=( BOUNDED_SURFACE ( )  B_SPLINE_SURFACE ( 3, 2, ( 
 ( #46821, #83280, #48699 ),
 ( #70517, #76201, #18424 ),
 ( #5644, #40640, #54407 ),
 ( #12754, #27412, #61540 ),
 ( #63426, #19365, #25528 ),
 ( #92255, #75723, #82817 ) ),
 .UNSPECIFIED., .F., .F., .F. ) 
 B_SPLINE_SURFACE_WITH_KNOTS ( ( 4, 2, 4 ),
 ( 3, 3 ),
 ( 5.756444938927698374, 6.019815123053642303, 6.283185307179586232 ),
 ( 0.000000000000000000, 1.000000000000000000 ),
 .UNSPECIFIED. ) 
 GEOMETRIC_REPRESENTATION_ITEM ( )  RATIONAL_B_SPLINE_SURFACE ( (
 ( 1.000000000000000000, 0.9186651033962672797, 1.000000000000000000),
 ( 1.000000000000000000, 0.9282241625911038518, 1.000000000000000000),
 ( 1.000000000000000000, 0.9354614375524440417, 1.000000000000000000),
 ( 1.000000000000000000, 0.9451322790882566993, 1.000000000000000000),
 ( 1.000000000000000000, 0.9475658968924186576, 1.000000000000000000),
 ( 1.000000000000000000, 0.9475641245298915827, 1.000000000000000000) ) ) 
 REPRESENTATION_ITEM ( '' )  SURFACE ( )  );
#19789=( BOUNDED_CURVE ( )  B_SPLINE_CURVE ( 3, ( #1518, #2467, #23301, #67336 ),
 .UNSPECIFIED., .F., .F. ) 
 B_SPLINE_CURVE_WITH_KNOTS ( ( 4, 4 ),
 ( 0.000000000000000000, 0.2609887789853130857 ),
 .UNSPECIFIED. ) 
 CURVE ( )  GEOMETRIC_REPRESENTATION_ITEM ( )  RATIONAL_B_SPLINE_CURVE ( ( 1.000000000000000000, 0.9943317885200935180, 0.9943317885200935180, 1.000000000000000000 ) ) 
 REPRESENTATION_ITEM ( '' )  );
#19793=CARTESIAN_POINT ( 'NONE',  ( 159.4851178187871312, 15.00000000000000000, 9.000000000000000000 ) ) ;
#19800=CIRCLE ( 'NONE', #62184, 25.00000000000000355 ) ;
#19806=CARTESIAN_POINT ( 'NONE',  ( 196.5083371989332761, 41.97678070738544420, 13.12846593433875775 ) ) ;
#19815=EDGE_LOOP ( 'NONE', ( #91912, #51590, #66215, #10760 ) ) ;
#19816=DIRECTION ( 'NONE',  ( -0.4999999999999952260, -0.8660254037844413721, 0.000000000000000000 ) ) ;
#19829=LINE ( 'NONE', #49645, #69747 ) ;
#19834=VERTEX_POINT ( 'NONE', #19757 ) ;
#19852=ORIENTED_EDGE ( 'NONE', *, *, #89992, .T. ) ;
#19863=AXIS2_PLACEMENT_3D ( 'NONE', #10737, #39137, #25417 ) ;
#19878=CARTESIAN_POINT ( 'NONE',  ( 193.9646936176702070, 20.00000000000000000, -15.00000000000000000 ) ) ;
#19899=CARTESIAN_POINT ( 'NONE',  ( 197.5277731217616122, 69.98851376390391010, 11.59179972292087513 ) ) ;
#19901=CYLINDRICAL_SURFACE ( 'NONE', #3577, 7.500000000000013323 ) ;
#19910=EDGE_CURVE ( 'NONE', #610, #39726, #77526, .T. ) ;
#19927=AXIS2_PLACEMENT_3D ( 'NONE', #3842, #32724, #45979 ) ;
#19942=CARTESIAN_POINT ( 'NONE',  ( 140.6539576904058606, 132.0000000000000568, 12.50000000000000000 ) ) ;
#19956=ORIENTED_EDGE ( 'NONE', *, *, #18018, .F. ) ;
#19958=ORIENTED_EDGE ( 'NONE', *, *, #81715, .T. ) ;
#19972=DIRECTION ( 'NONE',  ( 0.5068419345592570791, -2.990798612913347986E-15, 0.8620390091940327570 ) ) ;
#19978=ORIENTED_EDGE ( 'NONE', *, *, #133, .T. ) ;
#19985=EDGE_LOOP ( 'NONE', ( #73401, #27034, #84613, #64021, #93116, #2375 ) ) ;
#19986=CYLINDRICAL_SURFACE ( 'NONE', #4993, 0.5000000000000004441 ) ;
#19994=AXIS2_PLACEMENT_3D ( 'NONE', #58455, #65112, #57988 ) ;
#19997=CARTESIAN_POINT ( 'NONE',  ( 200.4644824113734387, 215.0000000000000568, -2.942835885954282471 ) ) ;
#20006=AXIS2_PLACEMENT_3D ( 'NONE', #87884, #37701, #16408 ) ;
#20008=AXIS2_PLACEMENT_3D ( 'NONE', #59763, #68243, #10459 ) ;
#20016=DIRECTION ( 'NONE',  ( 0.000000000000000000, 0.000000000000000000, 1.000000000000000000 ) ) ;
#20022=ADVANCED_FACE ( 'NONE', ( #85085 ), #36662, .T. ) ;
#20027=FACE_OUTER_BOUND ( 'NONE', #63093, .T. ) ;
#20030=CARTESIAN_POINT ( 'NONE',  ( 159.3464669004307268, 16.14910309755065398, -9.103988188768896705 ) ) ;
#20043=CARTESIAN_POINT ( 'NONE',  ( 207.2445280759194475, 36.58490166922437226, 13.79342392267524708 ) ) ;
#20045=ORIENTED_EDGE ( 'NONE', *, *, #16723, .T. ) ;
#20047=DIRECTION ( 'NONE',  ( -0.5877852522924802425, 0.000000000000000000, -0.8090169943749422332 ) ) ;
#20060=DIRECTION ( 'NONE',  ( -0.6056179655966478226, 0.7957555401921982963, 0.000000000000000000 ) ) ;
#20061=AXIS2_PLACEMENT_3D ( 'NONE', #49937, #79764, #93493 ) ;
#20069=VECTOR ( 'NONE', #53406, 1000.000000000000000 ) ;
#20071=CARTESIAN_POINT ( 'NONE',  ( 152.4536156746142410, 275.5000000000000568, -11.99999999999999289 ) ) ;
#20100=ORIENTED_EDGE ( 'NONE', *, *, #27543, .T. ) ;
#20103=AXIS2_PLACEMENT_3D ( 'NONE', #3381, #32269, #61175 ) ;
#20107=ORIENTED_EDGE ( 'NONE', *, *, #20400, .T. ) ;
#20122=AXIS2_PLACEMENT_3D ( 'NONE', #33052, #11740, #12700 ) ;
#20124=ADVANCED_FACE ( 'NONE', ( #50508 ), #58096, .F. ) ;
#20130=DIRECTION ( 'NONE',  ( 0.000000000000000000, 0.000000000000000000, 1.000000000000000000 ) ) ;
#20131=AXIS2_PLACEMENT_3D ( 'NONE', #56969, #79998, #20016 ) ;
#20134=VECTOR ( 'NONE', #69604, 1000.000000000000000 ) ;
#20137=AXIS2_PLACEMENT_3D ( 'NONE', #72293, #42937, #64756 ) ;
#20140=AXIS2_PLACEMENT_3D ( 'NONE', #65711, #24433, #67079 ) ;
#20142=CARTESIAN_POINT ( 'NONE',  ( 209.6287663260175975, 29.00782453271232697, 15.00000000000000000 ) ) ;
#20145=CARTESIAN_POINT ( 'NONE',  ( 196.1720347589760252, 41.44788071521509210, 14.04783121195910844 ) ) ;
#20146=LINE ( 'NONE', #6889, #54936 ) ;
#20149=CIRCLE ( 'NONE', #50573, 0.5000000000000004441 ) ;
#20160=LINE ( 'NONE', #40960, #69616 ) ;
#20161=CARTESIAN_POINT ( 'NONE',  ( 208.3427284608899868, 37.37804188714573428, 12.00000001296747598 ) ) ;
#20167=VECTOR ( 'NONE', #30776, 1000.000000000000000 ) ;
#20181=CARTESIAN_POINT ( 'NONE',  ( 180.2288731078812702, 275.0000000000000568, -24.90909090909093848 ) ) ;
#20205=VECTOR ( 'NONE', #63356, 1000.000000000000000 ) ;
#20210=EDGE_LOOP ( 'NONE', ( #40575, #9184, #70666, #77033, #40304, #39033 ) ) ;
#20220=ORIENTED_EDGE ( 'NONE', *, *, #32641, .T. ) ;
#20225=LINE ( 'NONE', #78001, #61348 ) ;
#20226=CARTESIAN_POINT ( 'NONE',  ( 180.6209651459523968, 249.5000000000000568, -24.41176470588237635 ) ) ;
#20227=AXIS2_PLACEMENT_3D ( 'NONE', #53558, #45971, #74877 ) ;
#20228=CYLINDRICAL_SURFACE ( 'NONE', #63967, 9.103929867429224387 ) ;
#20229=AXIS2_PLACEMENT_3D ( 'NONE', #63371, #71865, #28759 ) ;
#20235=DIRECTION ( 'NONE',  ( 0.000000000000000000, 0.000000000000000000, 1.000000000000000000 ) ) ;
#20236=CYLINDRICAL_SURFACE ( 'NONE', #50205, 9.550761578869391144 ) ;
#20238=ORIENTED_EDGE ( 'NONE', *, *, #18555, .T. ) ;
#20239=ORIENTED_EDGE ( 'NONE', *, *, #12108, .F. ) ;
#20240=DIRECTION ( 'NONE',  ( 0.000000000000000000, 1.000000000000000000, -0.000000000000000000 ) ) ;
#20244=EDGE_CURVE ( 'NONE', #11198, #46065, #82036, .T. ) ;
#20256=DIRECTION ( 'NONE',  ( 0.3024135303179589229, 0.9531768234071938961, 0.000000000000000000 ) ) ;
#20257=CYLINDRICAL_SURFACE ( 'NONE', #76085, 2.999999999999993783 ) ;
#20287=CIRCLE ( 'NONE', #86766, 2.046895004029262832 ) ;
#20289=CARTESIAN_POINT ( 'NONE',  ( 196.2170728810764615, 41.80684193227733658, 13.58578709450668320 ) ) ;
#20296=AXIS2_PLACEMENT_3D ( 'NONE', #30105, #72724, #45209 ) ;
#20300=CARTESIAN_POINT ( 'NONE',  ( 151.7270317713838210, 20.05858947365256739, 8.551724154028896407 ) ) ;
#20302=CARTESIAN_POINT ( 'NONE',  ( 208.3233536746733989, 28.67700077860474295, 12.92477606492824904 ) ) ;
#20311=AXIS2_PLACEMENT_3D ( 'NONE', #80602, #29513, #50811 ) ;
#20313=ORIENTED_EDGE ( 'NONE', *, *, #45978, .T. ) ;
#20314=CARTESIAN_POINT ( 'NONE',  ( 194.7788884907710099, 40.12874951497173015, 13.93756309559030981 ) ) ;
#20317=CARTESIAN_POINT ( 'NONE',  ( 180.6209651459523968, 214.5000000000000568, -24.41176470588237635 ) ) ;
#20319=ORIENTED_EDGE ( 'NONE', *, *, #48884, .T. ) ;
#20326=CARTESIAN_POINT ( 'NONE',  ( 196.0143093133015384, 73.40565171261609123, -11.99999999999998046 ) ) ;
#20327=DIRECTION ( 'NONE',  ( -0.9565177946839406031, 0.000000000000000000, 0.2916739763039735700 ) ) ;
#20342=EDGE_CURVE ( 'NONE', #10872, #68845, #23103, .T. ) ;
#20356=( BOUNDED_SURFACE ( )  B_SPLINE_SURFACE ( 3, 2, ( 
 ( #25654, #67832, #61215 ),
 ( #10976, #47896, #32775 ),
 ( #38923, #90495, #76798 ),
 ( #25202, #11924, #55019 ),
 ( #26606, #74943, #76334 ),
 ( #40311, #39381, #19040 ) ),
 .UNSPECIFIED., .F., .F., .F. ) 
 B_SPLINE_SURFACE_WITH_KNOTS ( ( 4, 2, 4 ),
 ( 3, 3 ),
 ( -7.034303695085952768E-16, 0.001865377553711360711, 0.003730755107423424852 ),
 ( 0.000000000000000000, 1.000000000000000000 ),
 .UNSPECIFIED. ) 
 GEOMETRIC_REPRESENTATION_ITEM ( )  RATIONAL_B_SPLINE_SURFACE ( (
 ( 1.000000000000000000, 0.7905694150420948807, 1.000000000000000000),
 ( 1.000000000000000000, 0.7808937784651016623, 1.000000000000000000),
 ( 1.000000000000000000, 0.7692487437979422804, 1.000000000000000000),
 ( 1.000000000000000000, 0.7414446453488179323, 1.000000000000000000),
 ( 1.000000000000000000, 0.7251800859724746307, 1.000000000000000000),
 ( 1.000000000000000000, 0.7071067811865491270, 1.000000000000000000) ) ) 
 REPRESENTATION_ITEM ( '' )  SURFACE ( )  );
#20361=ORIENTED_EDGE ( 'NONE', *, *, #8476, .F. ) ;
#20362=CARTESIAN_POINT ( 'NONE',  ( 156.5440870305766055, 214.9910457053126720, 17.21343741151179429 ) ) ;
#20364=( BOUNDED_SURFACE ( )  B_SPLINE_SURFACE ( 3, 2, ( 
 ( #74400, #60682, #59285 ),
 ( #89997, #82444, #82893 ),
 ( #30869, #9530, #46901 ),
 ( #66843, #25152, #54026 ),
 ( #38415, #10000, #23289 ),
 ( #52162, #39794, #81045 ) ),
 .UNSPECIFIED., .F., .F., .F. ) 
 B_SPLINE_SURFACE_WITH_KNOTS ( ( 4, 2, 4 ),
 ( 3, 3 ),
 ( 3.871320309816757899, 4.291854645100723786, 4.712388980384689674 ),
 ( 0.000000000000000000, 1.000000000000000000 ),
 .UNSPECIFIED. ) 
 GEOMETRIC_REPRESENTATION_ITEM ( )  RATIONAL_B_SPLINE_SURFACE ( (
 ( 1.000000000000000000, 0.7827533893364964079, 1.000000000000000000),
 ( 1.000000000000000000, 0.7737378266087827638, 1.000000000000000000),
 ( 1.000000000000000000, 0.7623946665074067264, 1.000000000000000000),
 ( 1.000000000000000000, 0.7365781863258152873, 1.000000000000000000),
 ( 1.000000000000000000, 0.7221049970984646516, 1.000000000000000000),
 ( 1.000000000000000000, 0.7071067811865487940, 1.000000000000000000) ) ) 
 REPRESENTATION_ITEM ( '' )  SURFACE ( )  );
#20366=AXIS2_PLACEMENT_3D ( 'NONE', #74111, #15426, #29173 ) ;
#20379=CARTESIAN_POINT ( 'NONE',  ( 207.5108682301385272, 1.050453206927881578, -7.446924052135294403 ) ) ;
#20387=CARTESIAN_POINT ( 'NONE',  ( 208.6208076322478746, 32.98517505407394168, 10.00000000000000000 ) ) ;
#20389=LINE ( 'NONE', #76271, #80699 ) ;
#20398=DIRECTION ( 'NONE',  ( 0.000000000000000000, 0.000000000000000000, -1.000000000000000000 ) ) ;
#20400=EDGE_CURVE ( 'NONE', #40555, #65034, #12510, .T. ) ;
#20401=CARTESIAN_POINT ( 'NONE',  ( 208.6208076322478746, 32.98517505407394168, 10.50000000000000000 ) ) ;
#20413=CYLINDRICAL_SURFACE ( 'NONE', #84660, 0.5000000000000004441 ) ;
#20427=VECTOR ( 'NONE', #9899, 1000.000000000000000 ) ;
#20429=CARTESIAN_POINT ( 'NONE',  ( 153.6987871352711181, 19.48326534539917887, -11.45812909362560639 ) ) ;
#20432=AXIS2_PLACEMENT_3D ( 'NONE', #14044, #26375, #34415 ) ;
#20440=CIRCLE ( 'NONE', #67344, 24.00000000000001066 ) ;
#20443=ORIENTED_EDGE ( 'NONE', *, *, #15864, .F. ) ;
#20445=VERTEX_POINT ( 'NONE', #51884 ) ;
#20461=CARTESIAN_POINT ( 'NONE',  ( 175.2296996224750103, 214.5000000000000568, 0.000000000000000000 ) ) ;
#20466=ADVANCED_FACE ( 'NONE', ( #42936 ), #57170, .F. ) ;
#20468=ORIENTED_EDGE ( 'NONE', *, *, #43976, .T. ) ;
#20475=VERTEX_POINT ( 'NONE', #71845 ) ;
#20476=DIRECTION ( 'NONE',  ( -0.3994899938747922263, 0.000000000000000000, 0.9167375550253837879 ) ) ;
#20487=FACE_OUTER_BOUND ( 'NONE', #74806, .T. ) ;
#20508=CARTESIAN_POINT ( 'NONE',  ( 200.2296996224750103, 66.43830042146294090, -4.834471782559336933E-14 ) ) ;
#20515=VECTOR ( 'NONE', #70891, 1000.000000000000000 ) ;
#20516=CARTESIAN_POINT ( 'NONE',  ( 197.2126074028028313, 40.90928511441033777, 12.12147092472265264 ) ) ;
#20519=CARTESIAN_POINT ( 'NONE',  ( 159.4572718888341569, 15.57755555264324521, -9.020884447463142664 ) ) ;
#20529=ORIENTED_EDGE ( 'NONE', *, *, #44158, .F. ) ;
#20532=DIRECTION ( 'NONE',  ( 0.9531768234072897084, -0.3024135303176576084, 0.000000000000000000 ) ) ;
#20540=EDGE_CURVE ( 'NONE', #23299, #135, #53306, .T. ) ;
#20564=ORIENTED_EDGE ( 'NONE', *, *, #13930, .T. ) ;
#20567=ORIENTED_EDGE ( 'NONE', *, *, #34464, .F. ) ;
#20581=ADVANCED_FACE ( 'NONE', ( #66580 ), #1700, .F. ) ;
#20586=ORIENTED_EDGE ( 'NONE', *, *, #2931, .F. ) ;
#20592=EDGE_LOOP ( 'NONE', ( #29508, #68190, #59002, #61897 ) ) ;
#20594=ORIENTED_EDGE ( 'NONE', *, *, #66162, .F. ) ;
#20613=DIRECTION ( 'NONE',  ( 1.000000000000000000, -0.000000000000000000, 0.000000000000000000 ) ) ;
#20665=EDGE_LOOP ( 'NONE', ( #9105, #11929, #43855, #60477 ) ) ;
#20670=ADVANCED_FACE ( 'NONE', ( #23941 ), #53283, .T. ) ;
#20676=CARTESIAN_POINT ( 'NONE',  ( 222.2216768131362130, 37.54180348216212337, 10.00000000000000000 ) ) ;
#20680=ORIENTED_EDGE ( 'NONE', *, *, #23679, .T. ) ;
#20685=EDGE_CURVE ( 'NONE', #87609, #47159, #1482, .T. ) ;
#20690=ORIENTED_EDGE ( 'NONE', *, *, #26705, .T. ) ;
#20694=ORIENTED_EDGE ( 'NONE', *, *, #62216, .T. ) ;
#20697=CYLINDRICAL_SURFACE ( 'NONE', #54855, 2.500000000000002220 ) ;
#20704=DIRECTION ( 'NONE',  ( -0.2456588035076310295, 0.9693563597868428694, 1.734723475976805517E-15 ) ) ;
#20708=CARTESIAN_POINT ( 'NONE',  ( 140.6539576904058606, 275.5000000000000568, -10.49999999999999822 ) ) ;
#20722=DIRECTION ( 'NONE',  ( 0.000000000000000000, 0.000000000000000000, 1.000000000000000000 ) ) ;
#20723=CARTESIAN_POINT ( 'NONE',  ( 154.1407330040854333, 275.0000000000000568, -13.42592592592594158 ) ) ;
#20738=DIRECTION ( 'NONE',  ( -0.000000000000000000, -0.000000000000000000, -1.000000000000000000 ) ) ;
#20751=CARTESIAN_POINT ( 'NONE',  ( 197.1656530321902494, 41.90019538913896469, 12.64285714285713524 ) ) ;
#20760=ORIENTED_EDGE ( 'NONE', *, *, #67389, .F. ) ;
#20761=CARTESIAN_POINT ( 'NONE',  ( 151.0528680457221355, 20.99319481056636505, 6.529293081340417082 ) ) ;
#20763=CARTESIAN_POINT ( 'NONE',  ( 209.3197381339219874, 28.92950916896207048, 12.09245862089610490 ) ) ;
#20773=FACE_OUTER_BOUND ( 'NONE', #32634, .T. ) ;
#20778=EDGE_CURVE ( 'NONE', #42785, #15573, #74387, .T. ) ;
#20779=ORIENTED_EDGE ( 'NONE', *, *, #85278, .T. ) ;
#20786=CARTESIAN_POINT ( 'NONE',  ( 221.4259212729440094, 36.93618551656547311, 7.000000000000000000 ) ) ;
#20787=CARTESIAN_POINT ( 'NONE',  ( 140.6539576904058606, 130.0000000000000568, 12.50000000000000000 ) ) ;
#20790=VERTEX_POINT ( 'NONE', #52813 ) ;
#20796=ORIENTED_EDGE ( 'NONE', *, *, #29441, .F. ) ;
#20806=DIRECTION ( 'NONE',  ( 0.6056179655966478226, -0.7957555401921982963, 0.000000000000000000 ) ) ;
#20809=EDGE_CURVE ( 'NONE', #61882, #75307, #3098, .T. ) ;
#20821=ORIENTED_EDGE ( 'NONE', *, *, #70919, .T. ) ;
#20823=CARTESIAN_POINT ( 'NONE',  ( 209.0105194359445875, 28.85114552632395046, 12.07126757350762603 ) ) ;
#20846=DIRECTION ( 'NONE',  ( 0.000000000000000000, 0.000000000000000000, 1.000000000000000000 ) ) ;
#20848=CARTESIAN_POINT ( 'NONE',  ( 196.6877655503061533, 293.9636489450775230, -7.999911143031724237 ) ) ;
#20859=DIRECTION ( 'NONE',  ( 0.000000000000000000, 0.000000000000000000, 1.000000000000000000 ) ) ;
#20867=EDGE_CURVE ( 'NONE', #63636, #10890, #45652, .T. ) ;
#20870=ORIENTED_EDGE ( 'NONE', *, *, #54992, .F. ) ;
#20871=CARTESIAN_POINT ( 'NONE',  ( 180.5131398354828320, 250.0000000000000568, -23.92352941176473635 ) ) ;
#20873=CARTESIAN_POINT ( 'NONE',  ( 175.2296996224750103, 161.0000000000000853, 0.000000000000000000 ) ) ;
#20886=PLANE ( 'NONE',  #19396 ) ;
#20889=TOROIDAL_SURFACE ( 'NONE', #45050, 5.603083949679977138, 1.500000000000000000 ) ;
#20903=( BOUNDED_CURVE ( )  B_SPLINE_CURVE ( 3, ( #22789, #50273, #21885, #42700 ),
 .UNSPECIFIED., .F., .F. ) 
 B_SPLINE_CURVE_WITH_KNOTS ( ( 4, 4 ),
 ( 1.570796326794896780, 3.141592653589793116 ),
 .UNSPECIFIED. ) 
 CURVE ( )  GEOMETRIC_REPRESENTATION_ITEM ( )  RATIONAL_B_SPLINE_CURVE ( ( 1.000000000000000000, 0.8047378541243650485, 0.8047378541243650485, 1.000000000000000000 ) ) 
 REPRESENTATION_ITEM ( '' )  );
#20917=DIRECTION ( 'NONE',  ( 0.000000000000000000, 1.000000000000000000, 0.000000000000000000 ) ) ;
#20922=VERTEX_POINT ( 'NONE', #16841 ) ;
#20929=VERTEX_POINT ( 'NONE', #38130 ) ;
#20930=CARTESIAN_POINT ( 'NONE',  ( 196.7536206669780086, 25.83949066589314469, 12.63456096898028669 ) ) ;
#20933=ADVANCED_FACE ( 'NONE', ( #67971 ), #23394, .T. ) ;
#20950=ORIENTED_EDGE ( 'NONE', *, *, #74672, .T. ) ;
#20957=AXIS2_PLACEMENT_3D ( 'NONE', #28197, #21538, #66051 ) ;
#20958=CARTESIAN_POINT ( 'NONE',  ( 154.5853110399403931, 19.45846805016676484, 12.72325134073231112 ) ) ;
#20965=CARTESIAN_POINT ( 'NONE',  ( 210.1640492649781322, 37.84931640281058662, 13.95110425196124027 ) ) ;
#20967=CARTESIAN_POINT ( 'NONE',  ( 175.2296996224750103, 247.0000000000001137, 0.000000000000000000 ) ) ;
#20970=DIRECTION ( 'NONE',  ( -1.000000000000000000, -0.000000000000000000, 0.000000000000000000 ) ) ;
#20971=PLANE ( 'NONE',  #57870 ) ;
#20981=ORIENTED_EDGE ( 'NONE', *, *, #93067, .F. ) ;
#20984=CARTESIAN_POINT ( 'NONE',  ( 197.3474984796250169, 24.88324032512257844, 12.41094495000513298 ) ) ;
#20986=ORIENTED_EDGE ( 'NONE', *, *, #13330, .T. ) ;
#20997=VERTEX_POINT ( 'NONE', #48999 ) ;
#21003=FACE_OUTER_BOUND ( 'NONE', #74970, .T. ) ;
#21011=DIRECTION ( 'NONE',  ( 1.000000000000000000, -0.000000000000000000, 0.000000000000000000 ) ) ;
#21018=VERTEX_POINT ( 'NONE', #77898 ) ;
#21027=AXIS2_PLACEMENT_3D ( 'NONE', #5836, #78276, #49834 ) ;
#21040=ORIENTED_EDGE ( 'NONE', *, *, #91063, .T. ) ;
#21046=ORIENTED_EDGE ( 'NONE', *, *, #89041, .F. ) ;
#21048=EDGE_CURVE ( 'NONE', #83682, #21221, #10913, .T. ) ;
#21049=ORIENTED_EDGE ( 'NONE', *, *, #5869, .T. ) ;
#21068=FACE_OUTER_BOUND ( 'NONE', #68565, .T. ) ;
#21072=CARTESIAN_POINT ( 'NONE',  ( 208.4306832106271088, 0.04196010845015941959, 7.500000000000013323 ) ) ;
#21079=DIRECTION ( 'NONE',  ( 0.4988042400434494761, -0.06911816301596634959, -0.8639542867860402486 ) ) ;
#21086=CIRCLE ( 'NONE', #90590, 0.4999999999999989453 ) ;
#21092=CARTESIAN_POINT ( 'NONE',  ( 156.5191989162425727, 249.5000000000000568, 16.58062614384861178 ) ) ;
#21097=EDGE_CURVE ( 'NONE', #82136, #26035, #39627, .T. ) ;
#21123=EDGE_LOOP ( 'NONE', ( #33789, #34515, #77819 ) ) ;
#21133=CARTESIAN_POINT ( 'NONE',  ( 209.2568086740256206, 34.98978593258856051, 15.00000000000000000 ) ) ;
#21134=CARTESIAN_POINT ( 'NONE',  ( 153.8801639287781029, 129.5385997557426379, -11.85807839311486234 ) ) ;
#21138=ORIENTED_EDGE ( 'NONE', *, *, #65268, .F. ) ;
#21151=CARTESIAN_POINT ( 'NONE',  ( 155.7140808774800007, 20.99999999999998934, -15.62500000000000711 ) ) ;
#21152=VECTOR ( 'NONE', #92349, 1000.000000000000000 ) ;
#21153=DIRECTION ( 'NONE',  ( 1.000000000000000000, 0.000000000000000000, 0.000000000000000000 ) ) ;
#21163=CARTESIAN_POINT ( 'NONE',  ( 164.6329196456214277, 214.9910457053126720, 23.09031830825856346 ) ) ;
#21179=CARTESIAN_POINT ( 'NONE',  ( 195.4562561984918148, 27.35676323194514126, 13.99999999999999822 ) ) ;
#21180=CARTESIAN_POINT ( 'NONE',  ( 199.0061125298537377, 275.5000000000000568, -7.725424859374024678 ) ) ;
#21206=CARTESIAN_POINT ( 'NONE',  ( 221.8344101925596306, 1.000000000000000222, 7.000000000000000000 ) ) ;
#21210=DIRECTION ( 'NONE',  ( 0.000000000000000000, 1.000000000000000000, 0.000000000000000000 ) ) ;
#21218=AXIS2_PLACEMENT_3D ( 'NONE', #53725, #23899, #2603 ) ;
#21221=VERTEX_POINT ( 'NONE', #34795 ) ;
#21235=CARTESIAN_POINT ( 'NONE',  ( 184.1778392089217107, 3.000000000000000444, -9.000000000000001776 ) ) ;
#21241=ORIENTED_EDGE ( 'NONE', *, *, #43478, .T. ) ;
#21247=CARTESIAN_POINT ( 'NONE',  ( 197.2083993959316786, 68.08024695722009767, -10.51981418967019799 ) ) ;
#21268=DIRECTION ( 'NONE',  ( 0.000000000000000000, 1.000000000000000000, 0.000000000000000000 ) ) ;
#21283=ORIENTED_EDGE ( 'NONE', *, *, #37042, .T. ) ;
#21284=CARTESIAN_POINT ( 'NONE',  ( 160.5350683151633291, 275.0000000000000568, 15.22542485937381329 ) ) ;
#21300=CARTESIAN_POINT ( 'NONE',  ( 200.2296996224750103, 66.43830042153604154, -2.389358538587389003 ) ) ;
#21301=CARTESIAN_POINT ( 'NONE',  ( 153.4750402936816727, 20.31599870471568536, -12.32002737771801115 ) ) ;
#21310=EDGE_CURVE ( 'NONE', #14641, #24267, #85453, .T. ) ;
#21311=DIRECTION ( 'NONE',  ( 0.000000000000000000, 0.000000000000000000, 1.000000000000000000 ) ) ;
#21322=FACE_OUTER_BOUND ( 'NONE', #40387, .T. ) ;
#21324=FACE_OUTER_BOUND ( 'NONE', #91996, .T. ) ;
#21333=EDGE_CURVE ( 'NONE', #41136, #13227, #24515, .T. ) ;
#21336=ORIENTED_EDGE ( 'NONE', *, *, #74127, .T. ) ;
#21339=LINE ( 'NONE', #36015, #2055 ) ;
#21351=CARTESIAN_POINT ( 'NONE',  ( 199.4757856505700886, 63.23505538068435783, -9.191047964625935762 ) ) ;
#21352=DIRECTION ( 'NONE',  ( 0.000000000000000000, 0.000000000000000000, 1.000000000000000000 ) ) ;
#21355=AXIS2_PLACEMENT_3D ( 'NONE', #30423, #15292, #79245 ) ;
#21359=VECTOR ( 'NONE', #21011, 1000.000000000000000 ) ;
#21372=VERTEX_POINT ( 'NONE', #91604 ) ;
#21401=CARTESIAN_POINT ( 'NONE',  ( 175.2296996224750103, 275.5000000000000568, 0.000000000000000000 ) ) ;
#21416=ADVANCED_FACE ( 'NONE', ( #84037 ), #63240, .T. ) ;
#21419=DIRECTION ( 'NONE',  ( 0.000000000000000000, 0.000000000000000000, 1.000000000000000000 ) ) ;
#21421=AXIS2_PLACEMENT_3D ( 'NONE', #50587, #6104, #7042 ) ;
#21426=CARTESIAN_POINT ( 'NONE',  ( 209.7912073884560300, 37.96760760058285200, 13.96055292456829378 ) ) ;
#21427=TOROIDAL_SURFACE ( 'NONE', #12362, 1.500000000000000888, 0.5000000000000000000 ) ;
#21429=DIRECTION ( 'NONE',  ( -1.000000000000000000, 0.000000000000000000, 0.000000000000000000 ) ) ;
#21432=CARTESIAN_POINT ( 'NONE',  ( 195.2901672131851285, 26.10222097264500363, 14.91929003175754964 ) ) ;
#21442=ADVANCED_FACE ( 'NONE', ( #61808 ), #91056, .F. ) ;
#21444=ORIENTED_EDGE ( 'NONE', *, *, #67159, .T. ) ;
#21464=FACE_OUTER_BOUND ( 'NONE', #2720, .T. ) ;
#21489=AXIS2_PLACEMENT_3D ( 'NONE', #50509, #35380, #57171 ) ;
#21492=AXIS2_PLACEMENT_3D ( 'NONE', #76742, #26069, #4766 ) ;
#21500=ORIENTED_EDGE ( 'NONE', *, *, #50606, .F. ) ;
#21502=AXIS2_PLACEMENT_3D ( 'NONE', #77215, #33184, #41680 ) ;
#21508=EDGE_LOOP ( 'NONE', ( #30650, #10628, #37549, #77600 ) ) ;
#21510=EDGE_CURVE ( 'NONE', #68845, #36747, #56113, .T. ) ;
#21511=ORIENTED_EDGE ( 'NONE', *, *, #12254, .F. ) ;
#21531=CARTESIAN_POINT ( 'NONE',  ( 175.2296996224750103, 133.0000000000000000, 0.000000000000000000 ) ) ;
#21535=CARTESIAN_POINT ( 'NONE',  ( 202.9738562182569694, 293.9636489450776367, 3.999999999999991562 ) ) ;
#21538=DIRECTION ( 'NONE',  ( -0.000000000000000000, -1.000000000000000000, -0.000000000000000000 ) ) ;
#21549=VECTOR ( 'NONE', #57524, 1000.000000000000000 ) ;
#21551=CIRCLE ( 'NONE', #7887, 1.000000000000000888 ) ;
#21555=DIRECTION ( 'NONE',  ( 0.000000000000000000, 1.000000000000000000, 0.000000000000000000 ) ) ;
#21561=AXIS2_PLACEMENT_3D ( 'NONE', #62397, #92648, #20235 ) ;
#21564=ADVANCED_FACE ( 'NONE', ( #18716 ), #90640, .T. ) ;
#21572=EDGE_CURVE ( 'NONE', #46575, #87978, #80475, .T. ) ;
#21584=AXIS2_PLACEMENT_3D ( 'NONE', #8531, #53494, #51610 ) ;
#21588=AXIS2_PLACEMENT_3D ( 'NONE', #46917, #90463, #90923 ) ;
#21599=CARTESIAN_POINT ( 'NONE',  ( 164.2231345125756263, 300.2961574867697436, -7.500000000000000000 ) ) ;
#21613=VERTEX_POINT ( 'NONE', #36193 ) ;
#21614=DIRECTION ( 'NONE',  ( -0.000000000000000000, -0.000000000000000000, -1.000000000000000000 ) ) ;
#21615=DIRECTION ( 'NONE',  ( 0.000000000000000000, 0.000000000000000000, -1.000000000000000000 ) ) ;
#21616=VECTOR ( 'NONE', #55650, 1000.000000000000000 ) ;
#21619=LINE ( 'NONE', #51766, #71526 ) ;
#21620=AXIS2_PLACEMENT_3D ( 'NONE', #42450, #56218, #78003 ) ;
#21626=EDGE_CURVE ( 'NONE', #61882, #14772, #29574, .T. ) ;
#21627=VECTOR ( 'NONE', #85369, 1000.000000000000000 ) ;
#21628=CARTESIAN_POINT ( 'NONE',  ( 209.1333812278717517, 27.85066937593108705, 13.99694255476963889 ) ) ;
#21631=VECTOR ( 'NONE', #90132, 1000.000000000000000 ) ;
#21633=LINE ( 'NONE', #50512, #74654 ) ;
#21635=EDGE_LOOP ( 'NONE', ( #52239, #23343, #38946, #51175, #34146 ) ) ;
#21636=DIRECTION ( 'NONE',  ( -0.000000000000000000, -1.000000000000000000, -0.000000000000000000 ) ) ;
#21652=CARTESIAN_POINT ( 'NONE',  ( 197.8594331107396727, 290.2795092986285113, -7.113038391050248599 ) ) ;
#21653=CYLINDRICAL_SURFACE ( 'NONE', #70087, 0.5000000000000004441 ) ;
#21655=AXIS2_PLACEMENT_3D ( 'NONE', #78179, #13317, #43574 ) ;
#21667=DIRECTION ( 'NONE',  ( 0.000000000000000000, 0.000000000000000000, 1.000000000000000000 ) ) ;
#21676=CARTESIAN_POINT ( 'NONE',  ( 196.4656634449348473, 42.34360782803825174, 11.30484575918238299 ) ) ;
#21679=CARTESIAN_POINT ( 'NONE',  ( 206.6166011988532887, 1.019566348684629364, 7.291626467228960351 ) ) ;
#21683=LINE ( 'NONE', #50080, #44320 ) ;
#21692=AXIS2_PLACEMENT_3D ( 'NONE', #47005, #75909, #3008 ) ;
#21695=CARTESIAN_POINT ( 'NONE',  ( 196.8803347170859865, 73.40565171261611965, 12.50000000000000711 ) ) ;
#21696=TOROIDAL_SURFACE ( 'NONE', #17151, 1.000000000000000000, 0.5000000000000000000 ) ;
#21698=CYLINDRICAL_SURFACE ( 'NONE', #42939, 3.000000000000002665 ) ;
#21708=ADVANCED_FACE ( 'NONE', ( #7771, #44210 ), #50398, .F. ) ;
#21710=ORIENTED_EDGE ( 'NONE', *, *, #44275, .T. ) ;
#21711=CARTESIAN_POINT ( 'NONE',  ( 195.2722580762363123, 41.12091610201859027, 13.20958711401371133 ) ) ;
#21718=ORIENTED_EDGE ( 'NONE', *, *, #85032, .F. ) ;
#21724=DIRECTION ( 'NONE',  ( 0.000000000000000000, 1.000000000000000000, 0.000000000000000000 ) ) ;
#21725=AXIS2_PLACEMENT_3D ( 'NONE', #18990, #69175, #83354 ) ;
#21726=LINE ( 'NONE', #87480, #79584 ) ;
#21727=CARTESIAN_POINT ( 'NONE',  ( 140.6539576904058606, 130.0000000000000568, -12.50000000000000000 ) ) ;
#21730=ORIENTED_EDGE ( 'NONE', *, *, #29582, .T. ) ;
#21734=ADVANCED_FACE ( 'NONE', ( #29095 ), #35261, .F. ) ;
#21762=ORIENTED_EDGE ( 'NONE', *, *, #17448, .T. ) ;
#21763=ORIENTED_EDGE ( 'NONE', *, *, #80495, .T. ) ;
#21764=FACE_OUTER_BOUND ( 'NONE', #30880, .T. ) ;
#21773=VECTOR ( 'NONE', #37231, 1000.000000000000000 ) ;
#21779=CARTESIAN_POINT ( 'NONE',  ( 200.6103193995254230, 249.5000000000000568, -2.464576988612307229 ) ) ;
#21780=DIRECTION ( 'NONE',  ( 0.000000000000000000, 1.000000000000000000, 0.000000000000000000 ) ) ;
#21781=AXIS2_PLACEMENT_3D ( 'NONE', #78153, #13757, #14233 ) ;
#21791=DIRECTION ( 'NONE',  ( 0.000000000000000000, 1.000000000000000000, 0.000000000000000000 ) ) ;
#21793=DIRECTION ( 'NONE',  ( -1.000000000000000000, 0.000000000000000000, 0.000000000000000000 ) ) ;
#21796=TOROIDAL_SURFACE ( 'NONE', #39927, 4.499999999999990230, 0.5000000000000000000 ) ;
#21802=DIRECTION ( 'NONE',  ( -0.000000000000000000, -0.000000000000000000, -1.000000000000000000 ) ) ;
#21803=CIRCLE ( 'NONE', #18742, 4.999999999999976907 ) ;
#21806=CARTESIAN_POINT ( 'NONE',  ( 200.5815643859950228, 65.97596549932491428, -9.780880230328993008 ) ) ;
#21807=FACE_OUTER_BOUND ( 'NONE', #12067, .T. ) ;
#21814=ORIENTED_EDGE ( 'NONE', *, *, #7026, .T. ) ;
#21815=CARTESIAN_POINT ( 'NONE',  ( 197.3133474189782248, 42.36571313990103960, 12.74999999999998757 ) ) ;
#21817=CARTESIAN_POINT ( 'NONE',  ( 156.4851178187871312, 0.000000000000000000, 10.00000000000000000 ) ) ;
#21829=CARTESIAN_POINT ( 'NONE',  ( 199.4392256788250677, 65.82574266882505754, -7.741079165001061746 ) ) ;
#21830=CARTESIAN_POINT ( 'NONE',  ( 0.000000000000000000, 0.000000000000000000, 7.500000000000000000 ) ) ;
#21833=AXIS2_PLACEMENT_3D ( 'NONE', #14450, #49006, #72202 ) ;
#21842=EDGE_LOOP ( 'NONE', ( #28374, #48829, #8511, #62270 ) ) ;
#21848=EDGE_CURVE ( 'NONE', #35960, #64853, #49924, .T. ) ;
#21852=VERTEX_POINT ( 'NONE', #78361 ) ;
#21860=DIRECTION ( 'NONE',  ( 2.220446049250312686E-15, 0.000000000000000000, 1.000000000000000000 ) ) ;
#21868=VECTOR ( 'NONE', #57358, 1000.000000000000000 ) ;
#21872=ORIENTED_EDGE ( 'NONE', *, *, #74020, .F. ) ;
#21877=EDGE_CURVE ( 'NONE', #33695, #78809, #50871, .T. ) ;
#21885=CARTESIAN_POINT ( 'NONE',  ( 222.8344101925596306, 6.488953147413177264E-16, 8.757359312880714342 ) ) ;
#21905=CARTESIAN_POINT ( 'NONE',  ( 209.5564680870925258, 38.04208312189877006, 12.07105558346621343 ) ) ;
#21910=CARTESIAN_POINT ( 'NONE',  ( 209.3407208048348878, 35.73852361108345121, 14.26380412667040432 ) ) ;
#21911=CARTESIAN_POINT ( 'NONE',  ( 208.6208076322478746, 32.98517505407394168, 13.99999999999999822 ) ) ;
#21923=CARTESIAN_POINT ( 'NONE',  ( 197.5281361355225442, 24.90961411280150983, 12.19683234139332839 ) ) ;
#21939=CARTESIAN_POINT ( 'NONE',  ( 196.6877655503061533, 293.9636489450775230, -7.999911143031724237 ) ) ;
#21942=CARTESIAN_POINT ( 'NONE',  ( 175.2296996224750103, 275.0000000000000568, 0.000000000000000000 ) ) ;
#21978=EDGE_LOOP ( 'NONE', ( #78101, #67174, #65868 ) ) ;
#21985=EDGE_LOOP ( 'NONE', ( #35558, #87329, #78928, #11679, #84705 ) ) ;
#21988=EDGE_CURVE ( 'NONE', #76803, #59473, #41112, .T. ) ;
#21995=EDGE_CURVE ( 'NONE', #35701, #42443, #74828, .T. ) ;
#22000=CARTESIAN_POINT ( 'NONE',  ( 169.2494399300530290, 8.542400036368780647, 10.00000000000000000 ) ) ;
#22012=CARTESIAN_POINT ( 'NONE',  ( 156.1711927057164644, 20.00000000000000000, 14.66327707481057629 ) ) ;
#22016=DIRECTION ( 'NONE',  ( 0.000000000000000000, 0.000000000000000000, -1.000000000000000000 ) ) ;
#22050=EDGE_CURVE ( 'NONE', #13346, #59473, #9429, .T. ) ;
#22064=TOROIDAL_SURFACE ( 'NONE', #56829, 24.50000000000000000, 0.5000000000000000000 ) ;
#22089=ORIENTED_EDGE ( 'NONE', *, *, #83847, .T. ) ;
#22090=CARTESIAN_POINT ( 'NONE',  ( 193.9646936176702070, 20.00000000000000000, 15.00000000000000000 ) ) ;
#22091=CARTESIAN_POINT ( 'NONE',  ( 196.9879731654527006, 24.91455852016545691, 12.95191548363261447 ) ) ;
#22097=DIRECTION ( 'NONE',  ( -1.000000000000000000, 0.000000000000000000, -0.000000000000000000 ) ) ;
#22098=CARTESIAN_POINT ( 'NONE',  ( 203.5977283565847813, 62.01285785379744198, -7.000000000000000888 ) ) ;
#22100=ADVANCED_FACE ( 'NONE', ( #86369 ), #71262, .T. ) ;
#22104=DIRECTION ( 'NONE',  ( 0.000000000000000000, 0.000000000000000000, -1.000000000000000000 ) ) ;
#22107=EDGE_CURVE ( 'NONE', #6460, #25984, #88030, .T. ) ;
#22117=CARTESIAN_POINT ( 'NONE',  ( 198.9668273763369370, 289.1149190245543537, -6.365503232778033649 ) ) ;
#22132=DIRECTION ( 'NONE',  ( -0.000000000000000000, -1.000000000000000000, -0.000000000000000000 ) ) ;
#22140=CARTESIAN_POINT ( 'NONE',  ( 196.3782803251243649, 41.22862212338403509, 11.42719184255257225 ) ) ;
#22143=CARTESIAN_POINT ( 'NONE',  ( 206.1702601134498991, 0.9999999999999995559, 7.166232077703399206 ) ) ;
#22156=ORIENTED_EDGE ( 'NONE', *, *, #57669, .T. ) ;
#22157=CARTESIAN_POINT ( 'NONE',  ( 198.7993789751180316, 65.26489576793395031, 10.60649040369606944 ) ) ;
#22159=CARTESIAN_POINT ( 'NONE',  ( 208.3931580544659710, 28.69469092964787293, 12.02378101520651299 ) ) ;
#22201=CARTESIAN_POINT ( 'NONE',  ( 156.8041522122653930, 250.5000000000000568, 16.89672165344857646 ) ) ;
#22214=VERTEX_POINT ( 'NONE', #37125 ) ;
#22215=EDGE_LOOP ( 'NONE', ( #69686, #82964, #67372, #46849, #21336 ) ) ;
#22221=EDGE_CURVE ( 'NONE', #69835, #14641, #66033, .T. ) ;
#22233=LINE ( 'NONE', #79990, #88158 ) ;
#22247=CARTESIAN_POINT ( 'NONE',  ( 201.8074164583845800, 62.71404347882092623, 8.782170572792690422 ) ) ;
#22267=ORIENTED_EDGE ( 'NONE', *, *, #25637, .F. ) ;
#22268=DIRECTION ( 'NONE',  ( 1.000000000000000000, 0.000000000000000000, 0.000000000000000000 ) ) ;
#22270=DIRECTION ( 'NONE',  ( 1.000000000000000000, 0.000000000000000000, 0.000000000000000000 ) ) ;
#22273=EDGE_CURVE ( 'NONE', #36583, #19033, #43300, .T. ) ;
#22274=EDGE_CURVE ( 'NONE', #3784, #82379, #72922, .T. ) ;
#22284=CARTESIAN_POINT ( 'NONE',  ( 200.3424981855932003, 61.71662552180350758, -9.000000000000000000 ) ) ;
#22310=DIRECTION ( 'NONE',  ( 0.000000000000000000, 0.000000000000000000, -1.000000000000000000 ) ) ;
#22322=ORIENTED_EDGE ( 'NONE', *, *, #58173, .F. ) ;
#22346=CARTESIAN_POINT ( 'NONE',  ( 154.0367246112803628, 19.37030481724588427, 11.97322993578355721 ) ) ;
#22352=DIRECTION ( 'NONE',  ( 0.000000000000000000, 0.000000000000000000, 1.000000000000000000 ) ) ;
#22357=DIRECTION ( 'NONE',  ( -0.4646852846009911220, 0.2294442726657859866, 0.8552326654286331875 ) ) ;
#22358=CYLINDRICAL_SURFACE ( 'NONE', #77592, 2.000000000000000000 ) ;
#22367=EDGE_LOOP ( 'NONE', ( #75508, #11117, #70015, #54411 ) ) ;
#22368=CARTESIAN_POINT ( 'NONE',  ( 201.2104617360081704, 60.19600395700752671, -6.999999999999999112 ) ) ;
#22381=ORIENTED_EDGE ( 'NONE', *, *, #90122, .T. ) ;
#22386=CARTESIAN_POINT ( 'NONE',  ( 153.9445672679061374, 19.37982107814384847, 11.06488088131597713 ) ) ;
#22389=CARTESIAN_POINT ( 'NONE',  ( 197.2116943569230045, 249.5000000000000568, -12.92446933126075592 ) ) ;
#22403=ORIENTED_EDGE ( 'NONE', *, *, #58734, .T. ) ;
#22411=B_SPLINE_CURVE_WITH_KNOTS ( 'NONE', 3,
 ( #71971, #85675, #20823, #49693, #78588, #35961 ),
 .UNSPECIFIED., .F., .F.,
 ( 4, 2, 4 ),
 ( 0.000000000000000000, 0.0009570384287224865559, 0.001914076857444973112 ),
 .UNSPECIFIED. ) ;
#22433=ORIENTED_EDGE ( 'NONE', *, *, #46209, .F. ) ;
#22445=DIRECTION ( 'NONE',  ( 0.000000000000000000, 0.000000000000000000, 1.000000000000000000 ) ) ;
#22451=CYLINDRICAL_SURFACE ( 'NONE', #79297, 2.000000000000001776 ) ;
#22457=CARTESIAN_POINT ( 'NONE',  ( 197.8563597697584839, 42.27872732282708057, 12.00000000000000355 ) ) ;
#22460=CARTESIAN_POINT ( 'NONE',  ( 222.2216768131362130, 37.54180348216212337, 7.000000000000000000 ) ) ;
#22462=B_SPLINE_CURVE_WITH_KNOTS ( 'NONE', 3,
 ( #76881, #32855, #12008, #89654, #53707, #82574, #17722, #46577, #61744, #90576, #5401, #92003 ),
 .UNSPECIFIED., .F., .F.,
 ( 4, 2, 2, 2, 2, 4 ),
 ( 0.000000000000000000, 0.002326201313189183318, 0.004652402626378366636, 0.006978603939567550388, 0.008141704596162134891, 0.009304805252756721129 ),
 .UNSPECIFIED. ) ;
#22499=EDGE_CURVE ( 'NONE', #31059, #10831, #51780, .T. ) ;
#22501=AXIS2_PLACEMENT_3D ( 'NONE', #35283, #65132, #13985 ) ;
#22538=ORIENTED_EDGE ( 'NONE', *, *, #71792, .T. ) ;
#22546=CARTESIAN_POINT ( 'NONE',  ( 153.9133111279453203, 20.47222690886559704, 13.06183683676577267 ) ) ;
#22550=ORIENTED_EDGE ( 'NONE', *, *, #31259, .F. ) ;
#22551=CARTESIAN_POINT ( 'NONE',  ( 199.4955644831718189, 40.18497343027721769, 10.63455718547475648 ) ) ;
#22557=AXIS2_PLACEMENT_3D ( 'NONE', #8601, #37931, #89519 ) ;
#22603=VERTEX_POINT ( 'NONE', #81589 ) ;
#22604=CARTESIAN_POINT ( 'NONE',  ( 196.8803347170859865, 73.40565171261611965, 12.50000000000000711 ) ) ;
#22615=ORIENTED_EDGE ( 'NONE', *, *, #10809, .F. ) ;
#22620=EDGE_CURVE ( 'NONE', #11326, #69004, #33570, .T. ) ;
#22625=CIRCLE ( 'NONE', #87635, 5.603083949679982467 ) ;
#22628=CARTESIAN_POINT ( 'NONE',  ( 159.6810783670777880, 8.542400036368780647, 25.74970488511327815 ) ) ;
#22631=AXIS2_PLACEMENT_3D ( 'NONE', #21535, #56131, #63727 ) ;
#22648=DIRECTION ( 'NONE',  ( 0.000000000000000000, 0.000000000000000000, 1.000000000000000000 ) ) ;
#22651=PLANE ( 'NONE',  #33949 ) ;
#22664=ORIENTED_EDGE ( 'NONE', *, *, #70808, .T. ) ;
#22665=ORIENTED_EDGE ( 'NONE', *, *, #69734, .F. ) ;
#22666=CARTESIAN_POINT ( 'NONE',  ( 197.7570118961458263, 17.87787486654844571, -10.88803913699953974 ) ) ;
#22669=ADVANCED_FACE ( 'NONE', ( #38962 ), #2547, .F. ) ;
#22681=CARTESIAN_POINT ( 'NONE',  ( 153.8044938463029041, 20.39556813534549207, -12.88425144204669870 ) ) ;
#22689=CARTESIAN_POINT ( 'NONE',  ( 159.4851178187871312, 0.000000000000000000, 7.000000000000000000 ) ) ;
#22692=DIRECTION ( 'NONE',  ( 0.000000000000000000, 1.000000000000000000, 0.000000000000000000 ) ) ;
#22694=AXIS2_PLACEMENT_3D ( 'NONE', #54742, #24952, #90700 ) ;
#22715=ORIENTED_EDGE ( 'NONE', *, *, #17571, .F. ) ;
#22716=DIRECTION ( 'NONE',  ( -0.000000000000000000, 0.000000000000000000, -1.000000000000000000 ) ) ;
#22719=DIRECTION ( 'NONE',  ( 0.000000000000000000, 0.000000000000000000, 1.000000000000000000 ) ) ;
#22726=EDGE_CURVE ( 'NONE', #77887, #19714, #29065, .T. ) ;
#22729=ORIENTED_EDGE ( 'NONE', *, *, #20778, .F. ) ;
#22733=EDGE_CURVE ( 'NONE', #1023, #39404, #23389, .T. ) ;
#22734=CARTESIAN_POINT ( 'NONE',  ( 154.5625123364532101, 250.0000000000000568, -13.15740740740742254 ) ) ;
#22737=LINE ( 'NONE', #53013, #72289 ) ;
#22746=EDGE_LOOP ( 'NONE', ( #86948, #66806, #23375, #26118, #46624, #65669, #90761, #62261, #88767, #91310, #67034, #88180, #77501, #91529, #62950, #37446, #69460, #12242, #82626, #64739, #73863, #64050, #59671, #38606, #42216 ) ) ;
#22753=CIRCLE ( 'NONE', #27305, 0.5000000000000022204 ) ;
#22755=ORIENTED_EDGE ( 'NONE', *, *, #65290, .T. ) ;
#22757=ORIENTED_EDGE ( 'NONE', *, *, #67229, .T. ) ;
#22759=CIRCLE ( 'NONE', #84741, 1.999999999999998002 ) ;
#22766=CARTESIAN_POINT ( 'NONE',  ( 154.5625123364532101, 275.5000000000000568, 13.15740740740740833 ) ) ;
#22772=ORIENTED_EDGE ( 'NONE', *, *, #49942, .F. ) ;
#22779=ORIENTED_EDGE ( 'NONE', *, *, #29447, .T. ) ;
#22780=CARTESIAN_POINT ( 'NONE',  ( 193.9402003287077605, 249.5000000000000568, 16.58062614384823874 ) ) ;
#22789=CARTESIAN_POINT ( 'NONE',  ( 219.8344101925596021, 3.000000000000000000, 10.00000000000000000 ) ) ;
#22798=VERTEX_POINT ( 'NONE', #32356 ) ;
#22813=( BOUNDED_CURVE ( )  B_SPLINE_CURVE ( 3, ( #20787, #49659, #77615, #64387 ),
 .UNSPECIFIED., .F., .F. ) 
 B_SPLINE_CURVE_WITH_KNOTS ( ( 4, 4 ),
 ( 0.000000000000000000, 1.570796326794896558 ),
 .UNSPECIFIED. ) 
 CURVE ( )  GEOMETRIC_REPRESENTATION_ITEM ( )  RATIONAL_B_SPLINE_CURVE ( ( 1.000000000000000000, 0.8047378541243649375, 0.8047378541243649375, 1.000000000000000000 ) ) 
 REPRESENTATION_ITEM ( '' )  );
#22814=CARTESIAN_POINT ( 'NONE',  ( 199.8090428943486643, 25.00736135706073426, 10.14950798392827558 ) ) ;
#22817=CARTESIAN_POINT ( 'NONE',  ( 207.7761861081325776, 35.69891260691534285, 14.41714557868295010 ) ) ;
#22828=ORIENTED_EDGE ( 'NONE', *, *, #81728, .F. ) ;
#22829=DIRECTION ( 'NONE',  ( 0.000000000000000000, 0.000000000000000000, 1.000000000000000000 ) ) ;
#22837=VECTOR ( 'NONE', #38804, 1000.000000000000000 ) ;
#22846=CARTESIAN_POINT ( 'NONE',  ( 196.9883954656811227, 295.9476850007761186, -7.765551635011542331 ) ) ;
#22850=DIRECTION ( 'NONE',  ( -1.000000000000000000, 0.000000000000000000, 0.000000000000000000 ) ) ;
#22888=ORIENTED_EDGE ( 'NONE', *, *, #81666, .F. ) ;
#22895=ORIENTED_EDGE ( 'NONE', *, *, #55843, .F. ) ;
#22898=ORIENTED_EDGE ( 'NONE', *, *, #86333, .F. ) ;
#22905=VECTOR ( 'NONE', #10267, 1000.000000000000000 ) ;
#22915=CARTESIAN_POINT ( 'NONE',  ( 160.5350683151633291, 215.0000000000000568, 20.22542485937379908 ) ) ;
#22921=CARTESIAN_POINT ( 'NONE',  ( 207.6662022560301182, 36.29800326561209545, 14.90057469441957316 ) ) ;
#22932=CARTESIAN_POINT ( 'NONE',  ( 208.3418117619747818, 38.42745601219718310, 12.00000000000000000 ) ) ;
#23000=ORIENTED_EDGE ( 'NONE', *, *, #15663, .F. ) ;
#23002=ADVANCED_FACE ( 'NONE', ( #9627 ), #30034, .T. ) ;
#23007=FACE_OUTER_BOUND ( 'NONE', #80080, .T. ) ;
#23012=VERTEX_POINT ( 'NONE', #11502 ) ;
#23013=CARTESIAN_POINT ( 'NONE',  ( 196.7383257810085695, 42.27872732282709478, 11.00000000000001066 ) ) ;
#23022=AXIS2_PLACEMENT_3D ( 'NONE', #25341, #2180, #16379 ) ;
#23038=FACE_OUTER_BOUND ( 'NONE', #44851, .T. ) ;
#23046=FACE_OUTER_BOUND ( 'NONE', #44420, .T. ) ;
#23052=CARTESIAN_POINT ( 'NONE',  ( 207.7836171167862460, 29.58337601776884540, 14.84040491829734165 ) ) ;
#23055=CARTESIAN_POINT ( 'NONE',  ( 175.2296996224749250, 250.5000000000000568, -24.99999999999999289 ) ) ;
#23069=CARTESIAN_POINT ( 'NONE',  ( 153.5035891336125360, 20.65792664182377791, 10.22121553831927088 ) ) ;
#23081=LINE ( 'NONE', #51038, #72787 ) ;
#23092=CARTESIAN_POINT ( 'NONE',  ( 196.0143093133015384, 73.40565171261611965, -12.00000000000000355 ) ) ;
#23103=CIRCLE ( 'NONE', #57872, 0.5000000000000004441 ) ;
#23116=CARTESIAN_POINT ( 'NONE',  ( 157.4970531492008661, 250.0000000000000568, 16.90571646082702983 ) ) ;
#23125=CARTESIAN_POINT ( 'NONE',  ( 184.1778392089217107, 3.000000000000000444, -9.000000000000001776 ) ) ;
#23128=VECTOR ( 'NONE', #89073, 1000.000000000000000 ) ;
#23130=ORIENTED_EDGE ( 'NONE', *, *, #30936, .T. ) ;
#23131=ORIENTED_EDGE ( 'NONE', *, *, #41338, .T. ) ;
#23132=CARTESIAN_POINT ( 'NONE',  ( 175.2296996224750103, 250.0000000000000568, 0.000000000000000000 ) ) ;
#23136=EDGE_CURVE ( 'NONE', #62353, #19834, #53298, .T. ) ;
#23148=CARTESIAN_POINT ( 'NONE',  ( 209.1374487190023501, 30.94653725228601360, 15.00000000000000000 ) ) ;
#23149=DIRECTION ( 'NONE',  ( 1.000000000000000000, 0.000000000000000000, 0.000000000000000000 ) ) ;
#23165=AXIS2_PLACEMENT_3D ( 'NONE', #59866, #2088, #29587 ) ;
#23189=EDGE_LOOP ( 'NONE', ( #49311, #35729, #36887, #56042, #64760, #52363, #3857 ) ) ;
#23190=LINE ( 'NONE', #52072, #27235 ) ;
#23191=VECTOR ( 'NONE', #25027, 1000.000000000000000 ) ;
#23209=CARTESIAN_POINT ( 'NONE',  ( 197.1856756230095868, 68.15307035998191054, 10.54037349550492664 ) ) ;
#23212=CARTESIAN_POINT ( 'NONE',  ( 222.8344101925596306, 35.72494958537217968, -7.000000000000000888 ) ) ;
#23220=ORIENTED_EDGE ( 'NONE', *, *, #44799, .T. ) ;
#23228=EDGE_LOOP ( 'NONE', ( #90608, #34429, #49692, #89140, #61656, #12006 ) ) ;
#23236=DIRECTION ( 'NONE',  ( -1.000000000000000000, 0.000000000000000000, 0.000000000000000000 ) ) ;
#23249=ORIENTED_EDGE ( 'NONE', *, *, #79144, .T. ) ;
#23276=DIRECTION ( 'NONE',  ( -1.387778780781440785E-14, 0.000000000000000000, 1.000000000000000000 ) ) ;
#23283=B_SPLINE_CURVE_WITH_KNOTS ( 'NONE', 3,
 ( #60500, #82717, #68999, #4130, #85529, #91687, #62853, #78442, #5544, #56682 ),
 .UNSPECIFIED., .F., .F.,
 ( 4, 2, 2, 2, 4 ),
 ( -1.807859651496474836E-05, 0.002330337966246291345, 0.004678754529007548082, 0.007027171091768803952, 0.009375587654530059822 ),
 .UNSPECIFIED. ) ;
#23284=DIRECTION ( 'NONE',  ( 0.000000000000000000, 1.000000000000000000, 0.000000000000000000 ) ) ;
#23286=CARTESIAN_POINT ( 'NONE',  ( 198.4595007507759021, 25.14564487145584692, 10.76846978260893195 ) ) ;
#23289=CARTESIAN_POINT ( 'NONE',  ( 200.4283040947223640, 40.93816728012065909, 10.50000000000114753 ) ) ;
#23290=CARTESIAN_POINT ( 'NONE',  ( 157.4851178187871312, 1.000000000000001332, 7.000000000000000000 ) ) ;
#23299=VERTEX_POINT ( 'NONE', #26171 ) ;
#23300=AXIS2_PLACEMENT_3D ( 'NONE', #22915, #45600, #65581 ) ;
#23301=CARTESIAN_POINT ( 'NONE',  ( 200.1145890159574208, 64.93834475843401322, 5.212391550061751921 ) ) ;
#23309=AXIS2_PLACEMENT_3D ( 'NONE', #81845, #73377, #88009 ) ;
#23317=AXIS2_PLACEMENT_3D ( 'NONE', #76162, #11295, #11754 ) ;
#23320=CARTESIAN_POINT ( 'NONE',  ( 185.8821869067168393, 215.0000000000000568, 23.16839473634431101 ) ) ;
#23325=AXIS2_PLACEMENT_3D ( 'NONE', #5807, #28063, #56953 ) ;
#23340=ORIENTED_EDGE ( 'NONE', *, *, #10248, .T. ) ;
#23343=ORIENTED_EDGE ( 'NONE', *, *, #51125, .F. ) ;
#23350=EDGE_CURVE ( 'NONE', #36174, #7661, #70224, .T. ) ;
#23354=VERTEX_POINT ( 'NONE', #41773 ) ;
#23364=VERTEX_POINT ( 'NONE', #3940 ) ;
#23375=ORIENTED_EDGE ( 'NONE', *, *, #85804, .T. ) ;
#23389=B_SPLINE_CURVE_WITH_KNOTS ( 'NONE', 3,
 ( #24302, #31426, #82058, #38027, #81136, #68338 ),
 .UNSPECIFIED., .F., .F.,
 ( 4, 2, 4 ),
 ( 0.000000000000000000, 0.0004262108901887199383, 0.0008524217803774398767 ),
 .UNSPECIFIED. ) ;
#23390=( BOUNDED_CURVE ( )  B_SPLINE_CURVE ( 3, ( #43445, #64803, #79452, #72793 ),
 .UNSPECIFIED., .F., .F. ) 
 B_SPLINE_CURVE_WITH_KNOTS ( ( 4, 4 ),
 ( 0.000000000000000000, 1.112150975886356141 ),
 .UNSPECIFIED. ) 
 CURVE ( )  GEOMETRIC_REPRESENTATION_ITEM ( )  RATIONAL_B_SPLINE_CURVE ( ( 1.000000000000000000, 0.8995554851226789106, 0.8995554851226789106, 1.000000000000000000 ) ) 
 REPRESENTATION_ITEM ( '' )  );
#23393=FACE_OUTER_BOUND ( 'NONE', #25682, .T. ) ;
#23394=( BOUNDED_SURFACE ( )  B_SPLINE_SURFACE ( 3, 2, ( 
 ( #46635, #24885, #90193 ),
 ( #2647, #32459, #61359 ),
 ( #60413, #54221, #76947 ),
 ( #41879, #62277, #77413 ),
 ( #4500, #47097, #26760 ),
 ( #76004, #27225, #84498 ),
 ( #70336, #92535, #11607 ),
 ( #26281, #33378, #40922 ) ),
 .UNSPECIFIED., .F., .F., .F. ) 
 B_SPLINE_SURFACE_WITH_KNOTS ( ( 4, 2, 2, 4 ),
 ( 3, 3 ),
 ( 1.734723475976807094E-18, 0.004223792520783738701, 0.006335688781175607617, 0.008447585041567475667 ),
 ( 0.000000000000000000, 1.000000000000000000 ),
 .UNSPECIFIED. ) 
 GEOMETRIC_REPRESENTATION_ITEM ( )  RATIONAL_B_SPLINE_SURFACE ( (
 ( 1.000000000000000000, 0.7071067811865475727, 1.000000000000000000),
 ( 1.000000000000000000, 0.7191403781184192434, 1.000000000000000000),
 ( 1.000000000000000000, 0.7377564866452818171, 1.000000000000000000),
 ( 1.000000000000000000, 0.7710512730017622385, 1.000000000000000000),
 ( 1.000000000000000000, 0.7830816923593137968, 1.000000000000000000),
 ( 1.000000000000000000, 0.8079768302254115575, 1.000000000000000000),
 ( 1.000000000000000000, 0.8207366415440850993, 1.000000000000000000),
 ( 1.000000000000000000, 0.8333723006562868685, 1.000000000000000000) ) ) 
 REPRESENTATION_ITEM ( '' )  SURFACE ( )  );
#23396=AXIS2_PLACEMENT_3D ( 'NONE', #37435, #67277, #50734 ) ;
#23402=CARTESIAN_POINT ( 'NONE',  ( 155.0193286407022981, 19.71512530817699016, 13.29403319965802410 ) ) ;
#23405=CARTESIAN_POINT ( 'NONE',  ( 152.4536156746142410, 275.0000000000000568, -11.50000000000000355 ) ) ;
#23429=CARTESIAN_POINT ( 'NONE',  ( 209.5571421737558353, 36.99274597021241107, 12.09245862095555601 ) ) ;
#23459=VERTEX_POINT ( 'NONE', #31539 ) ;
#23462=AXIS2_PLACEMENT_3D ( 'NONE', #75697, #46338, #67677 ) ;
#23477=AXIS2_PLACEMENT_3D ( 'NONE', #91322, #84226, #18917 ) ;
#23482=EDGE_LOOP ( 'NONE', ( #60303, #81125, #60140, #63694, #79397, #69219 ) ) ;
#23489=CARTESIAN_POINT ( 'NONE',  ( 196.2715852227941866, 71.88751843463604985, -11.58297462746890538 ) ) ;
#23490=CARTESIAN_POINT ( 'NONE',  ( 175.2296996224750103, 154.6894116713782807, 24.16304133878946558 ) ) ;
#23495=ORIENTED_EDGE ( 'NONE', *, *, #2023, .T. ) ;
#23496=CARTESIAN_POINT ( 'NONE',  ( 197.2991535282351379, 42.14527734682575755, 10.37297551676668839 ) ) ;
#23508=DIRECTION ( 'NONE',  ( -1.000000000000000000, 0.000000000000000000, 0.000000000000000000 ) ) ;
#23513=DIRECTION ( 'NONE',  ( 0.000000000000000000, 1.000000000000000000, 0.000000000000000000 ) ) ;
#23517=CARTESIAN_POINT ( 'NONE',  ( 221.8344101925596021, 1.000000000000000444, 8.171572875253808377 ) ) ;
#23526=LINE ( 'NONE', #87893, #47358 ) ;
#23536=DIRECTION ( 'NONE',  ( -0.000000000000000000, -1.000000000000000000, -0.000000000000000000 ) ) ;
#23538=AXIS2_PLACEMENT_3D ( 'NONE', #16372, #44776, #308 ) ;
#23552=CARTESIAN_POINT ( 'NONE',  ( 196.9829714441682427, 72.62824309771482945, 12.32222797397095704 ) ) ;
#23564=ORIENTED_EDGE ( 'NONE', *, *, #31692, .T. ) ;
#23575=CARTESIAN_POINT ( 'NONE',  ( 196.0143093133015384, 73.40565171261611965, -12.00000000000000355 ) ) ;
#23576=CARTESIAN_POINT ( 'NONE',  ( 196.0143093133015384, 250.0000000000000568, 11.99999999999998757 ) ) ;
#23580=VERTEX_POINT ( 'NONE', #38627 ) ;
#23605=LINE ( 'NONE', #74251, #20069 ) ;
#23610=ORIENTED_EDGE ( 'NONE', *, *, #52972, .T. ) ;
#23612=CARTESIAN_POINT ( 'NONE',  ( 197.7323754217837006, 18.47808631420720715, -11.36704352365809889 ) ) ;
#23625=CARTESIAN_POINT ( 'NONE',  ( 195.4781563537916043, 27.48493576247232895, 15.50000000000000000 ) ) ;
#23639=PLANE ( 'NONE',  #92853 ) ;
#23641=CYLINDRICAL_SURFACE ( 'NONE', #58087, 2.000000000000000000 ) ;
#23651=CARTESIAN_POINT ( 'NONE',  ( 206.6195589736935005, 30.30844190587211884, 15.00000000000000178 ) ) ;
#23662=VERTEX_POINT ( 'NONE', #54695 ) ;
#23663=CARTESIAN_POINT ( 'NONE',  ( 189.9243309297870610, 250.5000000000000568, 20.22542485937349355 ) ) ;
#23675=ORIENTED_EDGE ( 'NONE', *, *, #75724, .F. ) ;
#23678=CARTESIAN_POINT ( 'NONE',  ( 180.7287904564219332, 275.5000000000000568, -24.90000000000003411 ) ) ;
#23679=EDGE_CURVE ( 'NONE', #19395, #43024, #91126, .T. ) ;
#23684=LINE ( 'NONE', #2383, #70805 ) ;
#23700=VERTEX_POINT ( 'NONE', #26297 ) ;
#23707=CARTESIAN_POINT ( 'NONE',  ( 196.1963538710215857, 305.7026273589066250, -40.00000000000000711 ) ) ;
#23718=EDGE_LOOP ( 'NONE', ( #79138, #28168, #36998, #1237 ) ) ;
#23728=DIRECTION ( 'NONE',  ( -0.000000000000000000, 0.000000000000000000, -1.000000000000000000 ) ) ;
#23739=CARTESIAN_POINT ( 'NONE',  ( 206.0205385567603571, 30.15663536185482485, 14.00000000000000000 ) ) ;
#23747=DIRECTION ( 'NONE',  ( 1.000000000000000000, 0.000000000000000000, 0.000000000000000000 ) ) ;
#23749=DIRECTION ( 'NONE',  ( 0.000000000000000000, 0.000000000000000000, 1.000000000000000000 ) ) ;
#23752=CARTESIAN_POINT ( 'NONE',  ( 200.1126601882106968, 275.5000000000000568, -2.416251949619912409 ) ) ;
#23761=ADVANCED_FACE ( 'NONE', ( #61373 ), #56031, .T. ) ;
#23762=ORIENTED_EDGE ( 'NONE', *, *, #89138, .F. ) ;
#23766=CARTESIAN_POINT ( 'NONE',  ( 195.5540042012145818, 26.59710438755789141, 14.87405783778811852 ) ) ;
#23778=CARTESIAN_POINT ( 'NONE',  ( 156.4851178187871312, 14.99999999999999645, 10.00000000000000178 ) ) ;
#23779=EDGE_CURVE ( 'NONE', #37492, #79467, #400, .T. ) ;
#23799=VERTEX_POINT ( 'NONE', #69855 ) ;
#23802=EDGE_CURVE ( 'NONE', #40445, #93104, #27936, .T. ) ;
#23810=EDGE_LOOP ( 'NONE', ( #67824, #53642, #34446, #61347 ) ) ;
#23845=CARTESIAN_POINT ( 'NONE',  ( 186.6539576904058890, 276.0000000000000568, 11.60392986742922616 ) ) ;
#23860=CARTESIAN_POINT ( 'NONE',  ( 154.3564990690631191, 19.12150670424431098, -10.40578999957124040 ) ) ;
#23862=DIRECTION ( 'NONE',  ( 0.9167375550253848981, 0.000000000000000000, 0.3994899938747897283 ) ) ;
#23866=LINE ( 'NONE', #58477, #42917 ) ;
#23878=CARTESIAN_POINT ( 'NONE',  ( 180.2288731078812702, 249.5000000000000568, -24.90909090909092782 ) ) ;
#23899=DIRECTION ( 'NONE',  ( 0.000000000000000000, -1.000000000000000000, 0.000000000000000000 ) ) ;
#23911=ORIENTED_EDGE ( 'NONE', *, *, #33481, .F. ) ;
#23916=ADVANCED_FACE ( 'NONE', ( #19656 ), #48525, .T. ) ;
#23935=CARTESIAN_POINT ( 'NONE',  ( 196.5477508190182903, 71.74599609987329529, -11.11079997048496892 ) ) ;
#23941=FACE_OUTER_BOUND ( 'NONE', #78985, .T. ) ;
#23947=DIRECTION ( 'NONE',  ( 0.000000000000000000, 1.000000000000000000, 0.000000000000000000 ) ) ;
#23960=EDGE_CURVE ( 'NONE', #23364, #35701, #5475, .T. ) ;
#23962=CARTESIAN_POINT ( 'NONE',  ( 208.4306832106271656, 1.063508326895939327, -7.500000000000014211 ) ) ;
#23977=CARTESIAN_POINT ( 'NONE',  ( 195.0811277904324754, 39.36132622696000283, 15.19607843137254477 ) ) ;
#23980=DIRECTION ( 'NONE',  ( 0.000000000000000000, 0.000000000000000000, 1.000000000000000000 ) ) ;
#23981=CIRCLE ( 'NONE', #70846, 2.500000000000009326 ) ;
#23991=SPHERICAL_SURFACE ( 'NONE', #48710, 2.000000000000000000 ) ;
#24016=ORIENTED_EDGE ( 'NONE', *, *, #45671, .F. ) ;
#24017=DIRECTION ( 'NONE',  ( -0.000000000000000000, -1.000000000000000000, -0.000000000000000000 ) ) ;
#24027=CARTESIAN_POINT ( 'NONE',  ( 153.6987871352711181, 19.48326534539917887, -11.45812909362560639 ) ) ;
#24031=ORIENTED_EDGE ( 'NONE', *, *, #13958, .T. ) ;
#24040=VERTEX_POINT ( 'NONE', #6879 ) ;
#24050=VECTOR ( 'NONE', #12462, 1000.000000000000000 ) ;
#24059=CARTESIAN_POINT ( 'NONE',  ( 150.6539576904058606, 293.9636489450775230, 0.000000000000000000 ) ) ;
#24065=CARTESIAN_POINT ( 'NONE',  ( 197.0984808611934795, 19.93437704977705494, -12.12215979493057638 ) ) ;
#24079=EDGE_CURVE ( 'NONE', #68325, #35152, #12497, .T. ) ;
#24080=DIRECTION ( 'NONE',  ( 0.000000000000000000, 0.000000000000000000, -1.000000000000000000 ) ) ;
#24091=CARTESIAN_POINT ( 'NONE',  ( 179.1465552314772083, 8.542400036368780647, -9.000000000000001776 ) ) ;
#24103=DIRECTION ( 'NONE',  ( -0.000000000000000000, -1.000000000000000000, -0.000000000000000000 ) ) ;
#24114=ORIENTED_EDGE ( 'NONE', *, *, #33104, .F. ) ;
#24115=DIRECTION ( 'NONE',  ( -0.000000000000000000, -1.000000000000000000, -0.000000000000000000 ) ) ;
#24119=TOROIDAL_SURFACE ( 'NONE', #80094, 24.00000000000002132, 2.046895004029262388 ) ;
#24127=ORIENTED_EDGE ( 'NONE', *, *, #6444, .F. ) ;
#24132=DIRECTION ( 'NONE',  ( -1.000000000000000000, -0.000000000000000000, -0.000000000000000000 ) ) ;
#24135=LINE ( 'NONE', #8072, #15278 ) ;
#24158=CARTESIAN_POINT ( 'NONE',  ( 152.5990036449066736, 20.65770287760360446, -10.64853154254647549 ) ) ;
#24170=CARTESIAN_POINT ( 'NONE',  ( 207.2825244649536955, 35.50712927932389107, 14.50000000000000178 ) ) ;
#24183=TOROIDAL_SURFACE ( 'NONE', #55965, 24.16304133878946558, 4.003189038634632269 ) ;
#24191=EDGE_CURVE ( 'NONE', #63777, #72522, #17016, .T. ) ;
#24204=CARTESIAN_POINT ( 'NONE',  ( 189.4188515237862589, 293.9636489450775798, -9.103929867429222611 ) ) ;
#24207=DIRECTION ( 'NONE',  ( 0.000000000000000000, 0.000000000000000000, 1.000000000000000000 ) ) ;
#24208=ADVANCED_FACE ( 'NONE', ( #56126 ), #84979, .T. ) ;
#24222=DIRECTION ( 'NONE',  ( 0.6023974895724104606, -0.000000000000000000, 0.7981962569173435273 ) ) ;
#24234=CARTESIAN_POINT ( 'NONE',  ( 196.0143093133015384, 20.19615242270663913, 11.99999999999998757 ) ) ;
#24238=CARTESIAN_POINT ( 'NONE',  ( 219.8344101925596021, 35.72494958537217968, -7.000000000000000000 ) ) ;
#24239=B_SPLINE_CURVE_WITH_KNOTS ( 'NONE', 3,
 ( #19103, #4416, #33770, #18626, #47958, #5381, #76862, #69755 ),
 .UNSPECIFIED., .F., .F.,
 ( 4, 2, 2, 4 ),
 ( 0.000000000000000000, 0.0009268394340039029598, 0.001390259151005891845, 0.001853678868007880729 ),
 .UNSPECIFIED. ) ;
#24254=ORIENTED_EDGE ( 'NONE', *, *, #62073, .F. ) ;
#24267=VERTEX_POINT ( 'NONE', #28189 ) ;
#24278=ORIENTED_EDGE ( 'NONE', *, *, #50050, .F. ) ;
#24286=CARTESIAN_POINT ( 'NONE',  ( 157.1249521815137484, 17.17215575532202010, 9.360165637272318762 ) ) ;
#24291=ADVANCED_FACE ( 'NONE', ( #42836 ), #86380, .T. ) ;
#24302=CARTESIAN_POINT ( 'NONE',  ( 193.9153122143737562, 214.9910457053126720, 17.21343741151142481 ) ) ;
#24307=DIRECTION ( 'NONE',  ( -0.000000000000000000, -1.000000000000000000, -0.000000000000000000 ) ) ;
#24310=EDGE_CURVE ( 'NONE', #19733, #1988, #54851, .T. ) ;
#24314=DIRECTION ( 'NONE',  ( 0.7957555401921962979, 0.6056179655966504871, 0.000000000000000000 ) ) ;
#24316=AXIS2_PLACEMENT_3D ( 'NONE', #87698, #87243, #43246 ) ;
#24318=DIRECTION ( 'NONE',  ( 1.000000000000000000, 0.000000000000000000, 0.000000000000000000 ) ) ;
#24320=CARTESIAN_POINT ( 'NONE',  ( 157.2348298300751708, 18.48484813927241177, -11.40642999294778015 ) ) ;
#24322=CARTESIAN_POINT ( 'NONE',  ( 140.6539576904058606, 275.0000000000000568, 11.50000000000000000 ) ) ;
#24335=EDGE_LOOP ( 'NONE', ( #24254, #54781, #49576, #39692 ) ) ;
#24336=ORIENTED_EDGE ( 'NONE', *, *, #35942, .T. ) ;
#24361=DIRECTION ( 'NONE',  ( 0.000000000000000000, 1.000000000000000000, 0.000000000000000000 ) ) ;
#24373=EDGE_LOOP ( 'NONE', ( #60077, #42239, #11123, #14160 ) ) ;
#24375=VERTEX_POINT ( 'NONE', #77913 ) ;
#24386=AXIS2_PLACEMENT_3D ( 'NONE', #46251, #31601, #82247 ) ;
#24392=VERTEX_POINT ( 'NONE', #49015 ) ;
#24398=ORIENTED_EDGE ( 'NONE', *, *, #74108, .F. ) ;
#24404=DIRECTION ( 'NONE',  ( -1.000000000000000000, 0.000000000000000000, 0.000000000000000000 ) ) ;
#24409=LINE ( 'NONE', #35266, #21616 ) ;
#24425=EDGE_CURVE ( 'NONE', #31737, #14834, #89578, .T. ) ;
#24433=DIRECTION ( 'NONE',  ( 0.9167375550253600291, 0.000000000000000000, -0.3994899938748465162 ) ) ;
#24438=EDGE_CURVE ( 'NONE', #60939, #44442, #48773, .T. ) ;
#24439=FACE_OUTER_BOUND ( 'NONE', #33451, .T. ) ;
#24442=CARTESIAN_POINT ( 'NONE',  ( 189.4188515237862589, 293.9636489450775798, -40.00000000000000711 ) ) ;
#24447=AXIS2_PLACEMENT_3D ( 'NONE', #56017, #34244, #6773 ) ;
#24454=DIRECTION ( 'NONE',  ( 0.000000000000000000, 1.000000000000000000, 0.000000000000000000 ) ) ;
#24456=CIRCLE ( 'NONE', #48721, 7.999911143031724237 ) ;
#24468=ORIENTED_EDGE ( 'NONE', *, *, #44600, .F. ) ;
#24473=B_SPLINE_CURVE_WITH_KNOTS ( 'NONE', 3,
 ( #53908, #16991, #80927, #73826, #45856, #38287 ),
 .UNSPECIFIED., .F., .F.,
 ( 4, 2, 4 ),
 ( 0.000000000000000000, 0.0009305040472776272007, 0.001861008094555254401 ),
 .UNSPECIFIED. ) ;
#24497=EDGE_CURVE ( 'NONE', #70758, #65093, #7955, .T. ) ;
#24511=PLANE ( 'NONE',  #12882 ) ;
#24514=DIRECTION ( 'NONE',  ( -0.000000000000000000, -0.000000000000000000, 1.000000000000000000 ) ) ;
#24515=CIRCLE ( 'NONE', #15462, 0.4999999999999998335 ) ;
#24516=CARTESIAN_POINT ( 'NONE',  ( 196.5385635022496444, 69.63708600450605957, 11.34458575897557964 ) ) ;
#24525=CARTESIAN_POINT ( 'NONE',  ( 207.3218713672209219, 35.53307536961114721, 15.03205023726508038 ) ) ;
#24526=VECTOR ( 'NONE', #90224, 1000.000000000000000 ) ;
#24529=ORIENTED_EDGE ( 'NONE', *, *, #91068, .T. ) ;
#24530=CARTESIAN_POINT ( 'NONE',  ( 195.2847367049472780, 40.73792109368745429, 14.92657523498152550 ) ) ;
#24543=CARTESIAN_POINT ( 'NONE',  ( 196.1963538710216994, 282.2246705312485915, 13.99999999999999112 ) ) ;
#24544=DIRECTION ( 'NONE',  ( 0.9531768234071952284, -0.3024135303179549261, 4.196830803964638850E-15 ) ) ;
#24553=CARTESIAN_POINT ( 'NONE',  ( 207.5150553188103970, 0.03396820302666808677, 7.457905934263069803 ) ) ;
#24559=CARTESIAN_POINT ( 'NONE',  ( 194.3594942055387094, 21.00000000000000000, 14.50689422379897842 ) ) ;
#24580=ORIENTED_EDGE ( 'NONE', *, *, #82014, .T. ) ;
#24581=DIRECTION ( 'NONE',  ( 0.000000000000000000, 1.000000000000000000, 0.000000000000000000 ) ) ;
#24582=AXIS2_PLACEMENT_3D ( 'NONE', #31867, #38947, #45575 ) ;
#24585=CARTESIAN_POINT ( 'NONE',  ( 152.4536156746142410, 275.5000000000000568, -12.49999999999999289 ) ) ;
#24595=ORIENTED_EDGE ( 'NONE', *, *, #42879, .F. ) ;
#24600=ADVANCED_FACE ( 'NONE', ( #21068 ), #64665, .F. ) ;
#24602=PLANE ( 'NONE',  #7363 ) ;
#24603=ORIENTED_EDGE ( 'NONE', *, *, #31259, .T. ) ;
#24606=PLANE ( 'NONE',  #21584 ) ;
#24618=ORIENTED_EDGE ( 'NONE', *, *, #57248, .F. ) ;
#24627=ORIENTED_EDGE ( 'NONE', *, *, #90853, .T. ) ;
#24633=CARTESIAN_POINT ( 'NONE',  ( 197.9931848604286699, 24.71549707027390141, 9.866139269184797556 ) ) ;
#24644=ORIENTED_EDGE ( 'NONE', *, *, #1109, .F. ) ;
#24645=CARTESIAN_POINT ( 'NONE',  ( 195.4781563537916895, 27.48493576247233605, 14.00000000000009059 ) ) ;
#24647=CIRCLE ( 'NONE', #15597, 25.00000000000000000 ) ;
#24653=AXIS2_PLACEMENT_3D ( 'NONE', #59391, #80223, #15837 ) ;
#24657=AXIS2_PLACEMENT_3D ( 'NONE', #56943, #57854, #86240 ) ;
#24662=CIRCLE ( 'NONE', #77595, 0.5000000000000004441 ) ;
#24672=DIRECTION ( 'NONE',  ( 0.4878460013594530520, 0.3579938043661777813, 0.7961449082880726058 ) ) ;
#24675=TOROIDAL_SURFACE ( 'NONE', #26167, 4.500000000000002665, 0.5000000000000000000 ) ;
#24680=CARTESIAN_POINT ( 'NONE',  ( 199.7657144415678658, 41.62711076580291092, 9.999999999999998224 ) ) ;
#24683=CARTESIAN_POINT ( 'NONE',  ( 195.2403266774578583, 20.74618149458048677, -13.25394924001932395 ) ) ;
#24686=CYLINDRICAL_SURFACE ( 'NONE', #13950, 0.5000000000000004441 ) ;
#24687=LINE ( 'NONE', #68244, #4996 ) ;
#24690=ADVANCED_FACE ( 'NONE', ( #72209 ), #16745, .T. ) ;
#24696=ORIENTED_EDGE ( 'NONE', *, *, #40031, .T. ) ;
#24700=DIRECTION ( 'NONE',  ( 0.000000000000000000, 0.000000000000000000, -1.000000000000000000 ) ) ;
#24710=AXIS2_PLACEMENT_3D ( 'NONE', #38633, #67536, #46195 ) ;
#24712=CARTESIAN_POINT ( 'NONE',  ( 152.4536156746142410, 249.5000000000000568, -14.50000000000000000 ) ) ;
#24713=EDGE_CURVE ( 'NONE', #50286, #21852, #45606, .T. ) ;
#24716=DIRECTION ( 'NONE',  ( 1.000000000000000000, -2.081668171172166620E-14, 0.000000000000000000 ) ) ;
#24728=CIRCLE ( 'NONE', #39831, 7.999911143031724237 ) ;
#24735=VERTEX_POINT ( 'NONE', #22921 ) ;
#24739=AXIS2_PLACEMENT_3D ( 'NONE', #89046, #1966, #23276 ) ;
#24741=EDGE_CURVE ( 'NONE', #41734, #17649, #85076, .T. ) ;
#24751=AXIS2_PLACEMENT_3D ( 'NONE', #54960, #46899, #83836 ) ;
#24767=ORIENTED_EDGE ( 'NONE', *, *, #77420, .T. ) ;
#24792=CARTESIAN_POINT ( 'NONE',  ( 165.2494399300530290, 8.542400036368780647, 9.000000000000001776 ) ) ;
#24793=DIRECTION ( 'NONE',  ( 0.000000000000000000, 1.000000000000000000, 0.000000000000000000 ) ) ;
#24797=CARTESIAN_POINT ( 'NONE',  ( 209.8744251295252354, 28.03846817292548366, 12.09245862095555601 ) ) ;
#24800=CARTESIAN_POINT ( 'NONE',  ( 203.5977283565847529, 62.01285785379746329, 9.999999999999994671 ) ) ;
#24802=CYLINDRICAL_SURFACE ( 'NONE', #39170, 3.000000000000004885 ) ;
#24811=AXIS2_PLACEMENT_3D ( 'NONE', #54371, #33068, #26440 ) ;
#24812=CIRCLE ( 'NONE', #91292, 24.00000000000000355 ) ;
#24817=CIRCLE ( 'NONE', #33877, 1.000000000000000888 ) ;
#24823=DIRECTION ( 'NONE',  ( -0.01818181818182024526, 0.000000000000000000, -0.9998346970812742596 ) ) ;
#24839=EDGE_CURVE ( 'NONE', #34882, #75628, #85143, .T. ) ;
#24842=DIRECTION ( 'NONE',  ( 0.3529856947623295493, 0.9356287187197470656, 0.000000000000000000 ) ) ;
#24854=VERTEX_POINT ( 'NONE', #52268 ) ;
#24856=ORIENTED_EDGE ( 'NONE', *, *, #38856, .F. ) ;
#24859=ADVANCED_FACE ( 'NONE', ( #58921 ), #87310, .F. ) ;
#24873=ORIENTED_EDGE ( 'NONE', *, *, #42570, .F. ) ;
#24878=ORIENTED_EDGE ( 'NONE', *, *, #23136, .F. ) ;
#24879=AXIS2_PLACEMENT_3D ( 'NONE', #20461, #14303, #41254 ) ;
#24885=CARTESIAN_POINT ( 'NONE',  ( 150.4957602436334696, 20.00000000000000355, -3.637614988394445081 ) ) ;
#24892=CARTESIAN_POINT ( 'NONE',  ( 197.3195042448029710, 214.9800000937857476, -12.43273589989834704 ) ) ;
#24906=CARTESIAN_POINT ( 'NONE',  ( 196.2275076780419170, 72.70431358716514580, 11.63072960017908564 ) ) ;
#24914=CARTESIAN_POINT ( 'NONE',  ( 221.0059830678134460, 1.828427124746190957, 9.000000000000000000 ) ) ;
#24919=EDGE_CURVE ( 'NONE', #7041, #75392, #39763, .T. ) ;
#24924=LINE ( 'NONE', #46670, #73087 ) ;
#24933=DIRECTION ( 'NONE',  ( 0.5877852522924681411, 0.000000000000000000, -0.8090169943749512260 ) ) ;
#24948=EDGE_CURVE ( 'NONE', #93704, #63051, #51879, .T. ) ;
#24951=VERTEX_POINT ( 'NONE', #88707 ) ;
#24952=DIRECTION ( 'NONE',  ( 0.000000000000000000, 0.000000000000000000, 1.000000000000000000 ) ) ;
#24954=CARTESIAN_POINT ( 'NONE',  ( 209.5646630284975629, 29.26077267968336315, 13.08022668053246740 ) ) ;
#24956=CIRCLE ( 'NONE', #20432, 0.9999999999999986677 ) ;
#24964=AXIS2_PLACEMENT_3D ( 'NONE', #31720, #53495, #17521 ) ;
#24971=EDGE_CURVE ( 'NONE', #42443, #62086, #88164, .T. ) ;
#24978=CARTESIAN_POINT ( 'NONE',  ( 204.7786681169002350, 32.98517505407394168, 9.000000000000001776 ) ) ;
#24991=EDGE_CURVE ( 'NONE', #31159, #88967, #47336, .T. ) ;
#24992=VERTEX_POINT ( 'NONE', #37584 ) ;
#24997=CARTESIAN_POINT ( 'NONE',  ( 175.2296996224750103, 20.00000000000000000, 0.000000000000000000 ) ) ;
#25001=CARTESIAN_POINT ( 'NONE',  ( 153.2628468892384603, 20.37991841447901820, 11.93555113919330424 ) ) ;
#25010=CARTESIAN_POINT ( 'NONE',  ( 195.2034772323600009, 41.96650104946161974, 13.30704316118699992 ) ) ;
#25012=ORIENTED_EDGE ( 'NONE', *, *, #57248, .T. ) ;
#25013=CARTESIAN_POINT ( 'NONE',  ( 201.2104617360081704, 15.00000000000000711, 10.00000000000000178 ) ) ;
#25027=DIRECTION ( 'NONE',  ( 0.000000000000000000, -1.000000000000000000, 0.000000000000000000 ) ) ;
#25028=CARTESIAN_POINT ( 'NONE',  ( 154.1772290835151011, 20.65814982784352694, -13.49254024715964029 ) ) ;
#25030=AXIS2_PLACEMENT_3D ( 'NONE', #55838, #85176, #28364 ) ;
#25040=DIRECTION ( 'NONE',  ( -0.000000000000000000, 1.000000000000000000, -0.000000000000000000 ) ) ;
#25051=CARTESIAN_POINT ( 'NONE',  ( 140.6539576904058606, 275.0000000000000568, 10.50000000000000000 ) ) ;
#25061=EDGE_LOOP ( 'NONE', ( #86444, #33035, #6562, #31270 ) ) ;
#25062=CARTESIAN_POINT ( 'NONE',  ( 160.5350683151633291, 276.0000000000000568, 20.22542485937379908 ) ) ;
#25072=EDGE_LOOP ( 'NONE', ( #91105, #61658, #37081, #80168 ) ) ;
#25078=CARTESIAN_POINT ( 'NONE',  ( 196.2769060748385641, 71.88909962519697672, 11.58303352224541172 ) ) ;
#25082=DIRECTION ( 'NONE',  ( -0.000000000000000000, -0.000000000000000000, -1.000000000000000000 ) ) ;
#25091=EDGE_LOOP ( 'NONE', ( #60646, #28800, #78064, #79289, #4691, #20100 ) ) ;
#25119=DIRECTION ( 'NONE',  ( 1.000000000000000000, 0.000000000000000000, -0.000000000000000000 ) ) ;
#25145=EDGE_CURVE ( 'NONE', #25416, #50728, #44221, .T. ) ;
#25150=PLANE ( 'NONE',  #24751 ) ;
#25152=CARTESIAN_POINT ( 'NONE',  ( 199.6898571221144039, 41.17245366902173487, 10.18361224148079280 ) ) ;
#25153=CARTESIAN_POINT ( 'NONE',  ( 175.2296996224750103, 140.2072866198470251, 0.000000000000000000 ) ) ;
#25162=EDGE_LOOP ( 'NONE', ( #6103, #7029, #91039, #43148, #55361, #29948 ) ) ;
#25163=CARTESIAN_POINT ( 'NONE',  ( 189.9243309297870610, 250.0000000000000568, 20.22542485937349355 ) ) ;
#25177=CARTESIAN_POINT ( 'NONE',  ( 155.9223079842149104, 17.31716537717099058, 7.900495735314976287 ) ) ;
#25180=CYLINDRICAL_SURFACE ( 'NONE', #18305, 0.5000000000000004441 ) ;
#25196=ORIENTED_EDGE ( 'NONE', *, *, #20342, .F. ) ;
#25202=CARTESIAN_POINT ( 'NONE',  ( 194.7336594103350080, 19.94899969135506979, -14.16570715603806008 ) ) ;
#25207=ORIENTED_EDGE ( 'NONE', *, *, #48163, .F. ) ;
#25214=CARTESIAN_POINT ( 'NONE',  ( 150.6539576904058606, 293.9636489450775230, 9.103929867429224387 ) ) ;
#25226=ORIENTED_EDGE ( 'NONE', *, *, #73250, .F. ) ;
#25227=CARTESIAN_POINT ( 'NONE',  ( 175.2296996224750103, 250.5000000000000568, 0.000000000000000000 ) ) ;
#25231=VERTEX_POINT ( 'NONE', #74044 ) ;
#25238=CARTESIAN_POINT ( 'NONE',  ( 175.2296996224750103, 160.0000000000000568, -24.00000000000001066 ) ) ;
#25243=CARTESIAN_POINT ( 'NONE',  ( 208.1751813995450107, 30.16346637533325747, 14.32775664334902821 ) ) ;
#25248=CARTESIAN_POINT ( 'NONE',  ( 189.9243309297870610, 215.0000000000000568, 20.22542485937349355 ) ) ;
#25253=CARTESIAN_POINT ( 'NONE',  ( 208.6610832702913285, 1.063508326896295486, 7.500000000000013323 ) ) ;
#25254=CARTESIAN_POINT ( 'NONE',  ( 195.1565306243040823, 21.00000000082943430, 15.11139605583089462 ) ) ;
#25257=ADVANCED_FACE ( 'NONE', ( #89163 ), #1612, .F. ) ;
#25258=CARTESIAN_POINT ( 'NONE',  ( 184.5358909326088792, 2.965303559109565779, 10.00000000000000000 ) ) ;
#25260=ORIENTED_EDGE ( 'NONE', *, *, #80129, .T. ) ;
#25261=CARTESIAN_POINT ( 'NONE',  ( 208.7913547201125084, 38.28482993310899474, 14.12814564770278025 ) ) ;
#25266=CARTESIAN_POINT ( 'NONE',  ( 156.0793278192224420, 19.94580804510003347, -11.55434249967656690 ) ) ;
#25279=CARTESIAN_POINT ( 'NONE',  ( 153.6539576904058038, 131.0000000000000568, 12.50000000000000000 ) ) ;
#25298=DIRECTION ( 'NONE',  ( 0.000000000000000000, 0.000000000000000000, 1.000000000000000000 ) ) ;
#25314=EDGE_LOOP ( 'NONE', ( #30460, #62937, #15656, #22615 ) ) ;
#25330=VERTEX_POINT ( 'NONE', #32366 ) ;
#25335=ORIENTED_EDGE ( 'NONE', *, *, #13517, .F. ) ;
#25341=CARTESIAN_POINT ( 'NONE',  ( 175.2296996224750103, 20.99999999999998934, 0.000000000000000000 ) ) ;
#25355=DIRECTION ( 'NONE',  ( -0.000000000000000000, -1.000000000000000000, -0.000000000000000000 ) ) ;
#25361=DIRECTION ( 'NONE',  ( 0.000000000000000000, 0.000000000000000000, 1.000000000000000000 ) ) ;
#25372=EDGE_CURVE ( 'NONE', #67402, #9610, #84399, .T. ) ;
#25387=DIRECTION ( 'NONE',  ( 1.000000000000000000, -0.000000000000000000, 0.000000000000000000 ) ) ;
#25399=AXIS2_PLACEMENT_3D ( 'NONE', #56152, #70375, #83600 ) ;
#25401=ORIENTED_EDGE ( 'NONE', *, *, #93547, .T. ) ;
#25404=CARTESIAN_POINT ( 'NONE',  ( 165.2424497756046549, 249.5000000000000568, 22.91843887563435800 ) ) ;
#25416=VERTEX_POINT ( 'NONE', #55550 ) ;
#25417=DIRECTION ( 'NONE',  ( 1.000000000000000000, 0.000000000000000000, 0.000000000000000000 ) ) ;
#25426=DIRECTION ( 'NONE',  ( 0.000000000000000000, 0.000000000000000000, 1.000000000000000000 ) ) ;
#25431=ORIENTED_EDGE ( 'NONE', *, *, #12195, .F. ) ;
#25449=CARTESIAN_POINT ( 'NONE',  ( 154.1407330040854333, 128.0000000000000568, 13.42592592592592737 ) ) ;
#25450=CARTESIAN_POINT ( 'NONE',  ( 199.2296996224019381, 66.10105075032892330, 2.340466192621719177 ) ) ;
#25458=DIRECTION ( 'NONE',  ( 2.940294503956655304E-16, -0.000000000000000000, 1.000000000000000000 ) ) ;
#25460=VERTEX_POINT ( 'NONE', #68823 ) ;
#25461=CARTESIAN_POINT ( 'NONE',  ( 202.9738562182569694, 293.9636489450776367, -40.00000000000000711 ) ) ;
#25469=VECTOR ( 'NONE', #43320, 1000.000000000000000 ) ;
#25478=FACE_OUTER_BOUND ( 'NONE', #17602, .T. ) ;
#25489=ADVANCED_FACE ( 'NONE', ( #83461 ), #4876, .T. ) ;
#25502=DIRECTION ( 'NONE',  ( 0.000000000000000000, 0.000000000000000000, 1.000000000000000000 ) ) ;
#25508=EDGE_CURVE ( 'NONE', #42443, #2063, #3475, .T. ) ;
#25512=VERTEX_POINT ( 'NONE', #32826 ) ;
#25513=DIRECTION ( 'NONE',  ( 0.000000000000000000, 0.000000000000000000, 1.000000000000000000 ) ) ;
#25515=CARTESIAN_POINT ( 'NONE',  ( 199.4819116658660221, 63.22432295887224285, 9.188210044104504703 ) ) ;
#25524=ORIENTED_EDGE ( 'NONE', *, *, #80334, .T. ) ;
#25528=CARTESIAN_POINT ( 'NONE',  ( 199.2296996224750103, 68.12454877784578855, -2.107038703920835587 ) ) ;
#25553=ORIENTED_EDGE ( 'NONE', *, *, #74314, .F. ) ;
#25559=DIRECTION ( 'NONE',  ( 0.000000000000000000, 0.000000000000000000, -1.000000000000000000 ) ) ;
#25570=FACE_OUTER_BOUND ( 'NONE', #68906, .T. ) ;
#25589=DIRECTION ( 'NONE',  ( -0.000000000000000000, -1.000000000000000000, -0.000000000000000000 ) ) ;
#25602=DIRECTION ( 'NONE',  ( 0.000000000000000000, -1.000000000000000000, 9.656854691831248164E-17 ) ) ;
#25605=CARTESIAN_POINT ( 'NONE',  ( 156.2461366866179731, 19.34073763602960128, 8.651974842892217410 ) ) ;
#25613=EDGE_CURVE ( 'NONE', #3069, #78294, #30747, .T. ) ;
#25616=ORIENTED_EDGE ( 'NONE', *, *, #20540, .F. ) ;
#25620=CARTESIAN_POINT ( 'NONE',  ( 207.7755975652984830, 28.53818587417392294, 12.00000000000000000 ) ) ;
#25631=DIRECTION ( 'NONE',  ( 0.000000000000000000, 1.000000000000000000, 0.000000000000000000 ) ) ;
#25637=EDGE_CURVE ( 'NONE', #35960, #43712, #41246, .T. ) ;
#25649=ORIENTED_EDGE ( 'NONE', *, *, #73796, .F. ) ;
#25654=CARTESIAN_POINT ( 'NONE',  ( 196.0143093133015384, 19.33012701892219098, -12.49999999999999289 ) ) ;
#25657=VECTOR ( 'NONE', #14719, 1000.000000000000000 ) ;
#25660=ORIENTED_EDGE ( 'NONE', *, *, #8160, .F. ) ;
#25668=DIRECTION ( 'NONE',  ( 0.000000000000000000, 1.000000000000000000, 0.000000000000000000 ) ) ;
#25669=EDGE_CURVE ( 'NONE', #25873, #23364, #79148, .T. ) ;
#25673=ADVANCED_FACE ( 'NONE', ( #62181 ), #68348, .T. ) ;
#25675=ORIENTED_EDGE ( 'NONE', *, *, #59092, .T. ) ;
#25682=EDGE_LOOP ( 'NONE', ( #91921, #73430, #37427, #70140 ) ) ;
#25696=CARTESIAN_POINT ( 'NONE',  ( 209.0573810755008992, 30.16382728711827710, 15.12480380411953718 ) ) ;
#25702=DIRECTION ( 'NONE',  ( 0.09665007798479530177, -0.000000000000000000, 0.9953184226294281567 ) ) ;
#25707=DIRECTION ( 'NONE',  ( 0.000000000000000000, 0.000000000000000000, -1.000000000000000000 ) ) ;
#25708=CARTESIAN_POINT ( 'NONE',  ( 153.8631963276546628, 19.40208621445597004, 11.71714748521188731 ) ) ;
#25711=CARTESIAN_POINT ( 'NONE',  ( 156.4870464395701219, 215.0000000000000568, 17.29054515234685141 ) ) ;
#25713=CARTESIAN_POINT ( 'NONE',  ( 156.4677141125679611, 15.48129629386866313, -7.027845929950994552 ) ) ;
#25715=CARTESIAN_POINT ( 'NONE',  ( 206.6195589736935005, 30.30844190587212594, 14.49999999999999822 ) ) ;
#25727=ADVANCED_FACE ( 'NONE', ( #55073 ), #75448, .T. ) ;
#25728=VERTEX_POINT ( 'NONE', #91505 ) ;
#25734=ORIENTED_EDGE ( 'NONE', *, *, #54408, .F. ) ;
#25736=CARTESIAN_POINT ( 'NONE',  ( 140.6539576904058606, 250.0000000000000568, -12.00000000000000000 ) ) ;
#25741=EDGE_CURVE ( 'NONE', #50317, #26361, #45929, .T. ) ;
#25761=EDGE_CURVE ( 'NONE', #47569, #23012, #62528, .T. ) ;
#25766=ORIENTED_EDGE ( 'NONE', *, *, #92370, .T. ) ;
#25777=B_SPLINE_CURVE_WITH_KNOTS ( 'NONE', 3,
 ( #79657, #8139, #65470, #29470, #37022, #29926, #73481, #9045, #31320, #30858, #17580, #67766, #1496, #73929, #88119, #38860 ),
 .UNSPECIFIED., .F., .F.,
 ( 4, 2, 2, 2, 2, 2, 2, 4 ),
 ( 0.000000000000000000, 0.001195571706423382121, 0.001793357559635075458, 0.002391143412846768578, 0.002988929266058461699, 0.003586715119270155253, 0.004184500972481848373, 0.004782286825693541493 ),
 .UNSPECIFIED. ) ;
#25803=CARTESIAN_POINT ( 'NONE',  ( 222.0386546523673985, 36.13108063356137478, 10.00000000000000000 ) ) ;
#25807=CARTESIAN_POINT ( 'NONE',  ( 196.2586151081795833, 20.67842735233990581, -13.53470692911517581 ) ) ;
#25820=CARTESIAN_POINT ( 'NONE',  ( 197.4477343783226786, 67.35408903922716206, 10.31406111472453091 ) ) ;
#25828=CARTESIAN_POINT ( 'NONE',  ( 195.8229337057643988, 41.01736685183180953, 14.50757396441050773 ) ) ;
#25829=CARTESIAN_POINT ( 'NONE',  ( 197.3200855685783495, 41.90484851767786978, 12.40975777105213851 ) ) ;
#25834=DIRECTION ( 'NONE',  ( 0.000000000000000000, 0.000000000000000000, 1.000000000000000000 ) ) ;
#25859=ORIENTED_EDGE ( 'NONE', *, *, #43329, .T. ) ;
#25862=FACE_OUTER_BOUND ( 'NONE', #55297, .T. ) ;
#25863=CIRCLE ( 'NONE', #78817, 1.499999999999999556 ) ;
#25873=VERTEX_POINT ( 'NONE', #49372 ) ;
#25879=EDGE_CURVE ( 'NONE', #22798, #90266, #58001, .T. ) ;
#25885=DIRECTION ( 'NONE',  ( 5.551115123125777653E-14, 0.000000000000000000, 1.000000000000000000 ) ) ;
#25890=ORIENTED_EDGE ( 'NONE', *, *, #33498, .F. ) ;
#25907=DIRECTION ( 'NONE',  ( -0.6249999999999139577, -7.583341244675574300E-14, 0.7806247497998688445 ) ) ;
#25917=DIRECTION ( 'NONE',  ( 0.000000000000000000, 0.000000000000000000, 1.000000000000000000 ) ) ;
#25919=ORIENTED_EDGE ( 'NONE', *, *, #31277, .T. ) ;
#25921=EDGE_CURVE ( 'NONE', #27188, #46489, #5064, .T. ) ;
#25937=CARTESIAN_POINT ( 'NONE',  ( 196.1963538710215857, 305.7026273589066250, -40.00000000000000711 ) ) ;
#25938=CARTESIAN_POINT ( 'NONE',  ( 156.4851178187871312, 15.00000000000000000, -7.000000000000000888 ) ) ;
#25951=CARTESIAN_POINT ( 'NONE',  ( 170.2305261370685798, 249.5000000000000568, -24.90909090909089940 ) ) ;
#25959=FACE_OUTER_BOUND ( 'NONE', #30312, .T. ) ;
#25962=DIRECTION ( 'NONE',  ( -0.000000000000000000, -1.000000000000000000, -0.000000000000000000 ) ) ;
#25971=CARTESIAN_POINT ( 'NONE',  ( 156.4217629211117355, 119.0463968525363327, 7.000000000000000000 ) ) ;
#25973=CARTESIAN_POINT ( 'NONE',  ( 206.1704063851378805, -4.856322230924656715E-17, -7.166288341785295835 ) ) ;
#25979=B_SPLINE_CURVE_WITH_KNOTS ( 'NONE', 3,
 ( #10879, #53038, #40675, #89952 ),
 .UNSPECIFIED., .F., .F.,
 ( 4, 4 ),
 ( 0.000000000000000000, 9.632970524408665937E-05 ),
 .UNSPECIFIED. ) ;
#25984=VERTEX_POINT ( 'NONE', #78265 ) ;
#25995=CARTESIAN_POINT ( 'NONE',  ( 175.2296996224750103, 250.0000000000000568, 25.00000000000000355 ) ) ;
#25997=CARTESIAN_POINT ( 'NONE',  ( 195.1350936496258441, 26.65530528383335707, 15.12636463707340617 ) ) ;
#26004=CONICAL_SURFACE ( 'NONE', #10922, 4.025000000000000355, 0.7853981633973095011 ) ;
#26014=EDGE_CURVE ( 'NONE', #92711, #27803, #85355, .T. ) ;
#26016=ADVANCED_FACE ( 'NONE', ( #71160 ), #30268, .F. ) ;
#26020=CARTESIAN_POINT ( 'NONE',  ( 199.0872936271226195, 69.92583464099143953, 8.677435037599675383 ) ) ;
#26035=VERTEX_POINT ( 'NONE', #6288 ) ;
#26057=CARTESIAN_POINT ( 'NONE',  ( 200.9021118021030361, 65.55478020306156850, 5.267193185414368095 ) ) ;
#26062=CIRCLE ( 'NONE', #403, 2.999999999999998224 ) ;
#26067=TOROIDAL_SURFACE ( 'NONE', #68399, 24.50000000000000355, 0.5000000000000000000 ) ;
#26069=DIRECTION ( 'NONE',  ( -0.000000000000000000, -1.000000000000000000, -0.000000000000000000 ) ) ;
#26072=CARTESIAN_POINT ( 'NONE',  ( 175.2296996224750103, 250.5000000000000568, 25.00000000000000355 ) ) ;
#26082=EDGE_CURVE ( 'NONE', #11326, #41151, #65513, .T. ) ;
#26089=DIRECTION ( 'NONE',  ( -0.000000000000000000, -1.000000000000000000, -0.000000000000000000 ) ) ;
#26101=CARTESIAN_POINT ( 'NONE',  ( 139.6539576904058606, 275.0000000000000568, 10.50000000000000000 ) ) ;
#26102=CARTESIAN_POINT ( 'NONE',  ( 193.9153122143737562, 249.5000000000000568, 17.21343741151142481 ) ) ;
#26116=ORIENTED_EDGE ( 'NONE', *, *, #15864, .T. ) ;
#26118=ORIENTED_EDGE ( 'NONE', *, *, #86488, .T. ) ;
#26120=VECTOR ( 'NONE', #89158, 1000.000000000000000 ) ;
#26129=AXIS2_PLACEMENT_3D ( 'NONE', #226, #56614, #57078 ) ;
#26132=AXIS2_PLACEMENT_3D ( 'NONE', #25227, #47452, #68793 ) ;
#26137=AXIS2_PLACEMENT_3D ( 'NONE', #125, #71175, #27613 ) ;
#26142=ORIENTED_EDGE ( 'NONE', *, *, #50050, .T. ) ;
#26144=CIRCLE ( 'NONE', #53385, 4.999999999999976907 ) ;
#26148=EDGE_CURVE ( 'NONE', #83549, #84679, #60962, .T. ) ;
#26152=CARTESIAN_POINT ( 'NONE',  ( 208.6208076322478746, 32.98517505407394168, 12.09245862095555601 ) ) ;
#26158=ORIENTED_EDGE ( 'NONE', *, *, #19092, .F. ) ;
#26167=AXIS2_PLACEMENT_3D ( 'NONE', #35522, #56364, #29346 ) ;
#26171=CARTESIAN_POINT ( 'NONE',  ( 175.2296996224750103, 138.1603916158177583, 24.00000000000001421 ) ) ;
#26176=CIRCLE ( 'NONE', #80651, 24.00000000000000355 ) ;
#26182=CARTESIAN_POINT ( 'NONE',  ( 209.9972545312790544, 27.55378999303206200, 10.50000000000000000 ) ) ;
#26183=FACE_OUTER_BOUND ( 'NONE', #20210, .T. ) ;
#26186=DIRECTION ( 'NONE',  ( 0.9693563597868444237, 0.2456588035076248677, -0.000000000000000000 ) ) ;
#26188=VERTEX_POINT ( 'NONE', #36913 ) ;
#26189=FACE_OUTER_BOUND ( 'NONE', #67270, .T. ) ;
#26191=CARTESIAN_POINT ( 'NONE',  ( 175.2296996224750103, 20.99999999999998934, 0.000000000000000000 ) ) ;
#26200=TOROIDAL_SURFACE ( 'NONE', #70010, 4.499999999999990230, 0.5000000000000000000 ) ;
#26211=ORIENTED_EDGE ( 'NONE', *, *, #35647, .F. ) ;
#26213=DIRECTION ( 'NONE',  ( -0.000000000000000000, -1.000000000000000000, -0.000000000000000000 ) ) ;
#26230=CARTESIAN_POINT ( 'NONE',  ( 154.3435542972835322, 20.31589174421842614, -11.82430550600266628 ) ) ;
#26232=CIRCLE ( 'NONE', #79182, 1.000000000000000888 ) ;
#26249=VERTEX_POINT ( 'NONE', #70694 ) ;
#26271=ORIENTED_EDGE ( 'NONE', *, *, #78636, .F. ) ;
#26273=ORIENTED_EDGE ( 'NONE', *, *, #19380, .T. ) ;
#26281=CARTESIAN_POINT ( 'NONE',  ( 153.2628468892384888, 20.37991841447901109, -11.93555113919333266 ) ) ;
#26297=CARTESIAN_POINT ( 'NONE',  ( 175.2296996224750103, 275.5000000000000568, 25.00000000000000355 ) ) ;
#26303=CARTESIAN_POINT ( 'NONE',  ( 198.0025355114448757, 65.94618789579841689, 9.918135210125075929 ) ) ;
#26306=CIRCLE ( 'NONE', #74632, 25.00000000000000355 ) ;
#26307=DIRECTION ( 'NONE',  ( 0.000000000000000000, 0.000000000000000000, 1.000000000000000000 ) ) ;
#26310=DIRECTION ( 'NONE',  ( -0.000000000000000000, -1.000000000000000000, -0.000000000000000000 ) ) ;
#26311=DIRECTION ( 'NONE',  ( 0.000000000000000000, 0.000000000000000000, 1.000000000000000000 ) ) ;
#26324=FACE_OUTER_BOUND ( 'NONE', #52478, .T. ) ;
#26328=EDGE_CURVE ( 'NONE', #70640, #82273, #34698, .T. ) ;
#26331=LINE ( 'NONE', #19686, #1410 ) ;
#26346=VERTEX_POINT ( 'NONE', #5824 ) ;
#26348=VECTOR ( 'NONE', #42354, 1000.000000000000000 ) ;
#26358=CIRCLE ( 'NONE', #5221, 21.95310499597075804 ) ;
#26361=VERTEX_POINT ( 'NONE', #12451 ) ;
#26364=AXIS2_PLACEMENT_3D ( 'NONE', #72331, #65247, #34940 ) ;
#26373=FACE_OUTER_BOUND ( 'NONE', #87456, .T. ) ;
#26375=DIRECTION ( 'NONE',  ( 0.4878460013594548283, 0.3579938043661797242, -0.7961449082880704964 ) ) ;
#26387=CONICAL_SURFACE ( 'NONE', #73233, 9.550761578869391144, 0.7853981633974327359 ) ;
#26389=ORIENTED_EDGE ( 'NONE', *, *, #30098, .F. ) ;
#26394=DIRECTION ( 'NONE',  ( 0.000000000000000000, 0.000000000000000000, 1.000000000000000000 ) ) ;
#26396=DIRECTION ( 'NONE',  ( -0.000000000000000000, -0.000000000000000000, -1.000000000000000000 ) ) ;
#26404=CARTESIAN_POINT ( 'NONE',  ( 154.6618539303304658, 20.39582633401224498, 12.36945559417337215 ) ) ;
#26423=DIRECTION ( 'NONE',  ( -0.000000000000000000, 1.000000000000000000, -0.000000000000000000 ) ) ;
#26434=( BOUNDED_SURFACE ( )  B_SPLINE_SURFACE ( 3, 2, ( 
 ( #67300, #45957, #46876 ),
 ( #2428, #32228, #81935 ),
 ( #54001, #2880, #45015 ),
 ( #31765, #17089, #82870 ),
 ( #46417, #16163, #89494 ),
 ( #81019, #31308, #18023 ) ),
 .UNSPECIFIED., .F., .F., .F. ) 
 B_SPLINE_SURFACE_WITH_KNOTS ( ( 4, 2, 4 ),
 ( 3, 3 ),
 ( -2.088173384207081540E-16, 0.001011815784625562549, 0.002023631569251334132 ),
 ( 0.000000000000000000, 1.000000000000000000 ),
 .UNSPECIFIED. ) 
 GEOMETRIC_REPRESENTATION_ITEM ( )  RATIONAL_B_SPLINE_SURFACE ( (
 ( 1.000000000000000000, 0.6287211027133666752, 1.000000000000000000),
 ( 1.000000000000000000, 0.5832186976974050863, 1.000000000000000000),
 ( 1.000000000000000000, 0.5529292259169074075, 1.000000000000000000),
 ( 1.000000000000000000, 0.5121682666463089895, 1.000000000000000000),
 ( 1.000000000000000000, 0.5021481801630829356, 1.000000000000000000),
 ( 1.000000000000000000, 0.5021841165015863417, 1.000000000000000000) ) ) 
 REPRESENTATION_ITEM ( '' )  SURFACE ( )  );
#26437=ADVANCED_FACE ( 'NONE', ( #58698 ), #77317, .F. ) ;
#26440=DIRECTION ( 'NONE',  ( 0.000000000000000000, 0.000000000000000000, -1.000000000000000000 ) ) ;
#26451=CARTESIAN_POINT ( 'NONE',  ( 195.2805408448962510, 40.11065606325327337, 14.93368823901625930 ) ) ;
#26459=VERTEX_POINT ( 'NONE', #89399 ) ;
#26460=CARTESIAN_POINT ( 'NONE',  ( 197.5319251031163219, 24.91057433061638093, 12.19320131867666746 ) ) ;
#26472=ORIENTED_EDGE ( 'NONE', *, *, #48886, .T. ) ;
#26482=CARTESIAN_POINT ( 'NONE',  ( 184.7149167944524493, 8.542400036368780647, -9.000000000000001776 ) ) ;
#26483=B_SPLINE_CURVE_WITH_KNOTS ( 'NONE', 3,
 ( #47844, #76283, #5266, #11409 ),
 .UNSPECIFIED., .F., .F.,
 ( 4, 4 ),
 ( 0.000000000000000000, 0.001237645497661998958 ),
 .UNSPECIFIED. ) ;
#26484=FACE_OUTER_BOUND ( 'NONE', #90988, .T. ) ;
#26503=VERTEX_POINT ( 'NONE', #44924 ) ;
#26504=CARTESIAN_POINT ( 'NONE',  ( 200.2296996224750103, 68.12454877777268791, 4.413917820073312015 ) ) ;
#26522=LINE ( 'NONE', #61581, #58003 ) ;
#26530=CARTESIAN_POINT ( 'NONE',  ( 200.4972393895363041, 64.43555889006553627, -7.250946725472672050 ) ) ;
#26554=CARTESIAN_POINT ( 'NONE',  ( 198.4468466364687060, 42.00370313906616104, 10.58981561310753250 ) ) ;
#26558=CARTESIAN_POINT ( 'NONE',  ( 140.6539576904058606, 249.5000000000000568, -12.00000000000000000 ) ) ;
#26565=ADVANCED_FACE ( 'NONE', ( #74762 ), #46779, .F. ) ;
#26568=ORIENTED_EDGE ( 'NONE', *, *, #21510, .F. ) ;
#26569=DIRECTION ( 'NONE',  ( -0.000000000000000000, -1.000000000000000000, -0.000000000000000000 ) ) ;
#26585=CARTESIAN_POINT ( 'NONE',  ( 156.4870464395701219, 215.0000000000000568, 17.29054515234685141 ) ) ;
#26599=EDGE_LOOP ( 'NONE', ( #34419, #83919, #42062, #40906, #93406, #9727 ) ) ;
#26601=ORIENTED_EDGE ( 'NONE', *, *, #40288, .F. ) ;
#26606=CARTESIAN_POINT ( 'NONE',  ( 194.3571872280090815, 19.99999999999999645, -14.59147969791757582 ) ) ;
#26626=MANIFOLD_SOLID_BREP ( 'Chamfer1', #44620 ) ;
#26631=ORIENTED_EDGE ( 'NONE', *, *, #35543, .F. ) ;
#26635=EDGE_CURVE ( 'NONE', #2170, #52231, #15667, .T. ) ;
#26637=ORIENTED_EDGE ( 'NONE', *, *, #38745, .T. ) ;
#26644=DIRECTION ( 'NONE',  ( -0.8195702660916290849, 0.000000000000000000, -0.5729786897769377774 ) ) ;
#26653=AXIS2_PLACEMENT_3D ( 'NONE', #92153, #41003, #62364 ) ;
#26658=EDGE_CURVE ( 'NONE', #51979, #40097, #12640, .T. ) ;
#26670=CARTESIAN_POINT ( 'NONE',  ( 156.3365481965735455, 16.61859728808169834, -10.14856962220658154 ) ) ;
#26672=CARTESIAN_POINT ( 'NONE',  ( 206.9189553108847406, 30.70889394204682432, 14.49999999999999822 ) ) ;
#26684=EDGE_CURVE ( 'NONE', #76858, #4814, #24473, .T. ) ;
#26686=EDGE_LOOP ( 'NONE', ( #72283, #80038, #84095, #47063, #92348, #73770, #32301 ) ) ;
#26689=CARTESIAN_POINT ( 'NONE',  ( 208.6208076322478746, 32.98517505407394168, 12.09245862095555601 ) ) ;
#26691=VERTEX_POINT ( 'NONE', #8939 ) ;
#26705=EDGE_CURVE ( 'NONE', #73161, #45887, #71982, .T. ) ;
#26737=VECTOR ( 'NONE', #1790, 1000.000000000000000 ) ;
#26744=EDGE_LOOP ( 'NONE', ( #32317, #87743, #85385, #58832 ) ) ;
#26750=VERTEX_POINT ( 'NONE', #88939 ) ;
#26760=CARTESIAN_POINT ( 'NONE',  ( 152.6996702291409633, 19.85642976176117358, -8.932053473878653449 ) ) ;
#26777=CARTESIAN_POINT ( 'NONE',  ( 196.4521542616569434, 72.01334855021748638, 11.25845938509887034 ) ) ;
#26781=CARTESIAN_POINT ( 'NONE',  ( 209.3190042249899250, 30.23012903947020646, 14.26380412667039010 ) ) ;
#26802=LINE ( 'NONE', #55688, #40710 ) ;
#26820=CARTESIAN_POINT ( 'NONE',  ( 198.9670582353434156, 298.8125465311976541, -6.365364976313826695 ) ) ;
#26829=ORIENTED_EDGE ( 'NONE', *, *, #56718, .T. ) ;
#26839=DIRECTION ( 'NONE',  ( 0.000000000000000000, 1.000000000000000000, 0.000000000000000000 ) ) ;
#26843=ORIENTED_EDGE ( 'NONE', *, *, #62073, .T. ) ;
#26856=ORIENTED_EDGE ( 'NONE', *, *, #57902, .T. ) ;
#26859=CARTESIAN_POINT ( 'NONE',  ( 175.2296996224749250, 275.0000000000000568, -24.99999999999999289 ) ) ;
#26860=DIRECTION ( 'NONE',  ( 5.551115123125777653E-14, 0.000000000000000000, 1.000000000000000000 ) ) ;
#26868=CARTESIAN_POINT ( 'NONE',  ( 179.7289557593406357, 250.0000000000000568, -24.91818181818184641 ) ) ;
#26870=EDGE_CURVE ( 'NONE', #12173, #25231, #27589, .T. ) ;
#26873=ORIENTED_EDGE ( 'NONE', *, *, #82203, .T. ) ;
#26879=EDGE_CURVE ( 'NONE', #17769, #45666, #47215, .T. ) ;
#26889=DIRECTION ( 'NONE',  ( 0.000000000000000000, 0.000000000000000000, 1.000000000000000000 ) ) ;
#26890=CARTESIAN_POINT ( 'NONE',  ( 208.6208076322478746, 32.98517505407394168, 15.00000000000000000 ) ) ;
#26904=AXIS2_PLACEMENT_3D ( 'NONE', #64489, #14734, #72039 ) ;
#26912=CARTESIAN_POINT ( 'NONE',  ( 207.6175730408114930, 30.32598770090644180, 14.41714557868295898 ) ) ;
#26915=CARTESIAN_POINT ( 'NONE',  ( 195.6860740630249893, 40.71007109152891701, 14.68571759922588704 ) ) ;
#26923=ORIENTED_EDGE ( 'NONE', *, *, #32342, .T. ) ;
#26924=CARTESIAN_POINT ( 'NONE',  ( 152.8567950062511329, 19.85971597382930298, 11.17893457256845657 ) ) ;
#26935=VERTEX_POINT ( 'NONE', #8371 ) ;
#26942=ORIENTED_EDGE ( 'NONE', *, *, #52600, .F. ) ;
#26948=DIRECTION ( 'NONE',  ( 0.000000000000000000, 1.000000000000000000, 0.000000000000000000 ) ) ;
#26953=ORIENTED_EDGE ( 'NONE', *, *, #34457, .F. ) ;
#26970=AXIS2_PLACEMENT_3D ( 'NONE', #43768, #71281, #13521 ) ;
#26971=DIRECTION ( 'NONE',  ( -0.000000000000000000, 1.000000000000000000, -0.000000000000000000 ) ) ;
#26983=( BOUNDED_SURFACE ( )  B_SPLINE_SURFACE ( 3, 2, ( 
 ( #64818, #57686, #16442 ),
 ( #15508, #38199, #22157 ),
 ( #73743, #854, #8403 ),
 ( #37281, #15988, #2247 ),
 ( #51479, #88402, #37733 ),
 ( #73291, #81296, #8855 ),
 ( #65745, #15050, #45294 ),
 ( #36825, #72357, #44840 ),
 ( #79468, #66187, #23552 ),
 ( #60017, #21695, #22604 ) ),
 .UNSPECIFIED., .F., .F., .F. ) 
 B_SPLINE_SURFACE_WITH_KNOTS ( ( 4, 2, 2, 2, 4 ),
 ( 3, 3 ),
 ( -2.168404344971008868E-19, 0.002513556688247616140, 0.005027113376495232280, 0.007540670064742848420, 0.01005422675299046456 ),
 ( 0.000000000000000000, 1.000000000000000000 ),
 .UNSPECIFIED. ) 
 GEOMETRIC_REPRESENTATION_ITEM ( )  RATIONAL_B_SPLINE_SURFACE ( (
 ( 1.000000000000000000, 0.8168508380123947754, 1.000000000000000000),
 ( 1.000000000000000000, 0.8469576315470376260, 1.000000000000000000),
 ( 1.000000000000000000, 0.8738409315859991811, 1.000000000000000000),
 ( 1.000000000000000000, 0.9200669567821229133, 1.000000000000000000),
 ( 1.000000000000000000, 0.9394145480628903755, 1.000000000000000000),
 ( 1.000000000000000000, 0.9701920524520508682, 1.000000000000000000),
 ( 1.000000000000000000, 0.9815163856013096044, 1.000000000000000000),
 ( 1.000000000000000000, 0.9964122006646789487, 1.000000000000000000),
 ( 1.000000000000000000, 1.000002041055608526, 1.000000000000000000),
 ( 1.000000000000000000, 1.000000000000000000, 1.000000000000000000) ) ) 
 REPRESENTATION_ITEM ( '' )  SURFACE ( )  );
#26989=( BOUNDED_SURFACE ( )  B_SPLINE_SURFACE ( 3, 2, ( 
 ( #28438, #21806, #43105 ),
 ( #6670, #27982, #58266 ),
 ( #63979, #80015, #72012 ),
 ( #15156, #14247, #36000 ),
 ( #13769, #28900, #93287 ),
 ( #50679, #56873, #42142 ),
 ( #35547, #64918, #71537 ),
 ( #64460, #79565, #7576 ),
 ( #57788, #57331, #92819 ),
 ( #86638, #42618, #87109 ) ),
 .UNSPECIFIED., .F., .F., .F. ) 
 B_SPLINE_SURFACE_WITH_KNOTS ( ( 4, 2, 2, 2, 4 ),
 ( 3, 3 ),
 ( 0.000000000000000000, 0.002512116609398717254, 0.005024233218797434508, 0.007536349828196151762, 0.01004846643759486902 ),
 ( 0.000000000000000000, 1.000000000000000000 ),
 .UNSPECIFIED. ) 
 GEOMETRIC_REPRESENTATION_ITEM ( )  RATIONAL_B_SPLINE_SURFACE ( (
 ( 1.000000000000000000, 0.8168508380123951085, 1.000000000000000000),
 ( 1.000000000000000000, 0.8469983227716978424, 1.000000000000000000),
 ( 1.000000000000000000, 0.8738795229725317970, 1.000000000000000000),
 ( 1.000000000000000000, 0.9200744724125300422, 1.000000000000000000),
 ( 1.000000000000000000, 0.9393932456999677383, 1.000000000000000000),
 ( 1.000000000000000000, 0.9701270577441517551, 1.000000000000000000),
 ( 1.000000000000000000, 0.9814990972768018462, 1.000000000000000000),
 ( 1.000000000000000000, 0.9964108658801225094, 1.000000000000000000),
 ( 1.000000000000000000, 1.000001410412673541, 1.000000000000000000),
 ( 1.000000000000000000, 1.000000000000000000, 1.000000000000000000) ) ) 
 REPRESENTATION_ITEM ( '' )  SURFACE ( )  );
#27010=CARTESIAN_POINT ( 'NONE',  ( 200.2296996224750103, 66.43830042146294090, 0.000000000000000000 ) ) ;
#27012=CARTESIAN_POINT ( 'NONE',  ( 184.7149167944524493, 8.542400036368780647, 9.000000000000001776 ) ) ;
#27034=ORIENTED_EDGE ( 'NONE', *, *, #44915, .F. ) ;
#27037=DIRECTION ( 'NONE',  ( -0.9693563597868447568, -0.2456588035076236187, 0.000000000000000000 ) ) ;
#27047=EDGE_CURVE ( 'NONE', #6353, #40624, #6428, .T. ) ;
#27064=ORIENTED_EDGE ( 'NONE', *, *, #84782, .T. ) ;
#27066=ORIENTED_EDGE ( 'NONE', *, *, #84321, .F. ) ;
#27071=EDGE_CURVE ( 'NONE', #19834, #62353, #38152, .T. ) ;
#27076=ORIENTED_EDGE ( 'NONE', *, *, #29049, .F. ) ;
#27095=ORIENTED_EDGE ( 'NONE', *, *, #59092, .F. ) ;
#27099=EDGE_CURVE ( 'NONE', #55010, #4883, #3359, .T. ) ;
#27101=VERTEX_POINT ( 'NONE', #74164 ) ;
#27115=CARTESIAN_POINT ( 'NONE',  ( 207.6175730408114646, 30.32598770090645246, 14.41714557868296076 ) ) ;
#27126=DIRECTION ( 'NONE',  ( 1.000000000000000000, -0.000000000000000000, 0.000000000000000000 ) ) ;
#27136=CARTESIAN_POINT ( 'NONE',  ( 175.2296996224750103, 275.5000000000000568, 0.000000000000000000 ) ) ;
#27139=CARTESIAN_POINT ( 'NONE',  ( 160.5350683151633291, 275.0000000000000568, -7.500000000000000000 ) ) ;
#27149=ORIENTED_EDGE ( 'NONE', *, *, #69768, .F. ) ;
#27154=EDGE_LOOP ( 'NONE', ( #26142, #22089, #83780, #648 ) ) ;
#27169=VECTOR ( 'NONE', #33906, 1000.000000000000000 ) ;
#27171=CYLINDRICAL_SURFACE ( 'NONE', #71185, 5.000000000000004441 ) ;
#27174=CIRCLE ( 'NONE', #18107, 0.5000000000000004441 ) ;
#27180=CARTESIAN_POINT ( 'NONE',  ( 157.4851178187871596, 1.000000000000000444, 8.171572875253808377 ) ) ;
#27188=VERTEX_POINT ( 'NONE', #17353 ) ;
#27191=ORIENTED_EDGE ( 'NONE', *, *, #85924, .F. ) ;
#27215=ORIENTED_EDGE ( 'NONE', *, *, #89850, .F. ) ;
#27218=EDGE_LOOP ( 'NONE', ( #12040, #18317, #12682, #17845 ) ) ;
#27225=CARTESIAN_POINT ( 'NONE',  ( 152.5497490326757202, 19.93678331745850585, -10.54177645505017935 ) ) ;
#27235=VECTOR ( 'NONE', #29383, 1000.000000000000000 ) ;
#27244=CARTESIAN_POINT ( 'NONE',  ( 156.4851178187871312, 69.18068689461284748, 10.00000000000000000 ) ) ;
#27251=CARTESIAN_POINT ( 'NONE',  ( 195.4737936193521648, 39.72103918308751247, 14.98565046456482008 ) ) ;
#27252=DIRECTION ( 'NONE',  ( -1.000000000000000000, -0.000000000000000000, -0.000000000000000000 ) ) ;
#27265=CARTESIAN_POINT ( 'NONE',  ( 175.2296996224750103, 250.0000000000000568, 0.000000000000000000 ) ) ;
#27268=CARTESIAN_POINT ( 'NONE',  ( 195.7212220663432163, 20.45996914382524423, -12.49744573203606279 ) ) ;
#27286=CARTESIAN_POINT ( 'NONE',  ( 156.0603832538696452, 17.29324094227561304, 10.42473456490728267 ) ) ;
#27297=ORIENTED_EDGE ( 'NONE', *, *, #73162, .F. ) ;
#27305=AXIS2_PLACEMENT_3D ( 'NONE', #75038, #46592, #24842 ) ;
#27309=CARTESIAN_POINT ( 'NONE',  ( 183.0442525570908288, 300.2961574867697436, -4.888549259831427740 ) ) ;
#27311=VECTOR ( 'NONE', #37606, 1000.000000000000000 ) ;
#27314=VERTEX_POINT ( 'NONE', #16871 ) ;
#27323=EDGE_LOOP ( 'NONE', ( #46817, #53388, #8560, #65884 ) ) ;
#27330=CARTESIAN_POINT ( 'NONE',  ( 197.4836817735085219, 42.27872732282707346, 11.66666666666666785 ) ) ;
#27331=CARTESIAN_POINT ( 'NONE',  ( 199.0143093133015100, 17.19615242270663202, 9.000000000000001776 ) ) ;
#27337=CARTESIAN_POINT ( 'NONE',  ( 208.0212563688061209, 27.56882951438707607, 14.33494424848942295 ) ) ;
#27338=DIRECTION ( 'NONE',  ( 0.000000000000000000, 0.000000000000000000, 1.000000000000000000 ) ) ;
#27357=CARTESIAN_POINT ( 'NONE',  ( 193.5407199155270064, 275.7877658745666167, 16.89624193776961647 ) ) ;
#27358=CARTESIAN_POINT ( 'NONE',  ( 206.7809450508160865, 35.77530089738193908, 15.00000000000000000 ) ) ;
#27385=CARTESIAN_POINT ( 'NONE',  ( 165.2494399300530290, 8.542400036368780647, -9.000000000000001776 ) ) ;
#27394=FACE_OUTER_BOUND ( 'NONE', #14380, .T. ) ;
#27396=CARTESIAN_POINT ( 'NONE',  ( 207.7755975652984830, 28.53818587417392294, 11.99999999999999822 ) ) ;
#27400=EDGE_CURVE ( 'NONE', #21372, #60748, #75370, .T. ) ;
#27409=CARTESIAN_POINT ( 'NONE',  ( 204.6539576904058606, 296.7472757692770529, 7.500000000000000000 ) ) ;
#27412=CARTESIAN_POINT ( 'NONE',  ( 198.8852758280200419, 66.55360856414498016, -4.692040283682947788 ) ) ;
#27414=VERTEX_POINT ( 'NONE', #1272 ) ;
#27420=FACE_OUTER_BOUND ( 'NONE', #6484, .T. ) ;
#27425=ORIENTED_EDGE ( 'NONE', *, *, #46545, .T. ) ;
#27431=EDGE_LOOP ( 'NONE', ( #62243, #68209, #41368, #61536, #67965, #48827, #55810, #22779, #11314, #41330, #42104, #91102, #5549, #4851, #7613 ) ) ;
#27441=AXIS2_PLACEMENT_3D ( 'NONE', #44395, #2262, #44852 ) ;
#27455=ORIENTED_EDGE ( 'NONE', *, *, #54344, .T. ) ;
#27471=CARTESIAN_POINT ( 'NONE',  ( 199.9390245229519110, 68.58287003106127599, -4.389327654518210942 ) ) ;
#27472=DIRECTION ( 'NONE',  ( 0.000000000000000000, 0.000000000000000000, 1.000000000000000000 ) ) ;
#27481=DIRECTION ( 'NONE',  ( -0.9510565162951498674, 0.000000000000000000, 0.3090169943749591086 ) ) ;
#27483=CARTESIAN_POINT ( 'NONE',  ( 159.4851178187871312, 0.000000000000000000, 10.00000000000000000 ) ) ;
#27493=CARTESIAN_POINT ( 'NONE',  ( 157.4851178187871312, 15.00000000000000000, 7.000000000000000888 ) ) ;
#27504=CIRCLE ( 'NONE', #71382, 2.000000000000000000 ) ;
#27507=AXIS2_PLACEMENT_3D ( 'NONE', #45493, #51226, #38410 ) ;
#27515=CIRCLE ( 'NONE', #45597, 0.4999999999999991673 ) ;
#27519=B_SPLINE_CURVE_WITH_KNOTS ( 'NONE', 3,
 ( #40982, #33924, #62832, #75145, #10257, #32048, #60942, #36134, #1084, #70395, #15289, #65509, #66417, #79696, #43691, #26820, #87694, #55706, #56173, #51713, #80149, #8631, #22846, #57922, #13100, #36594, #629, #21939 ),
 .UNSPECIFIED., .F., .F.,
 ( 4, 2, 2, 2, 2, 2, 2, 2, 2, 2, 2, 2, 2, 4 ),
 ( 0.000000000000000000, 0.0007588366528438087811, 0.001517673305687617562, 0.002276509958531426452, 0.003035346611375235124, 0.004553019917062885863, 0.005311856569906778236, 0.006070693222750670609, 0.006829529875594562982, 0.007588366528438454488, 0.009106039834126240101, 0.01062371313981402485, 0.01138254979265798661, 0.01214138644550194837 ),
 .UNSPECIFIED. ) ;
#27525=CARTESIAN_POINT ( 'NONE',  ( 196.1963538710215857, 305.7026273589066250, -40.00000000000000711 ) ) ;
#27526=CARTESIAN_POINT ( 'NONE',  ( 152.4773011712318578, 19.90414083357004671, -8.234854308319460969 ) ) ;
#27540=VERTEX_POINT ( 'NONE', #84990 ) ;
#27543=EDGE_CURVE ( 'NONE', #26691, #49791, #33888, .T. ) ;
#27549=VERTEX_POINT ( 'NONE', #18269 ) ;
#27556=DIRECTION ( 'NONE',  ( 0.000000000000000000, 0.000000000000000000, 1.000000000000000000 ) ) ;
#27561=ORIENTED_EDGE ( 'NONE', *, *, #81578, .T. ) ;
#27568=VERTEX_POINT ( 'NONE', #34359 ) ;
#27569=CARTESIAN_POINT ( 'NONE',  ( 205.2786681169002350, 32.98517505407394168, 15.00000000000000000 ) ) ;
#27577=VECTOR ( 'NONE', #7314, 1000.000000000000000 ) ;
#27580=CARTESIAN_POINT ( 'NONE',  ( 156.4851178187871312, 0.000000000000000000, -7.000000000000000888 ) ) ;
#27589=CIRCLE ( 'NONE', #7891, 24.00000000000000355 ) ;
#27591=CIRCLE ( 'NONE', #71392, 0.5000000000000128786 ) ;
#27599=DIRECTION ( 'NONE',  ( -0.000000000000000000, 1.000000000000000000, -0.000000000000000000 ) ) ;
#27600=CARTESIAN_POINT ( 'NONE',  ( 153.3249703231417982, 19.65100358619422849, 12.05267380659650556 ) ) ;
#27606=PLANE ( 'NONE',  #49939 ) ;
#27608=CARTESIAN_POINT ( 'NONE',  ( 209.2522817606372882, 36.37164913089609541, 14.78224109794540198 ) ) ;
#27610=DIRECTION ( 'NONE',  ( -0.000000000000000000, -1.000000000000000000, -0.000000000000000000 ) ) ;
#27613=DIRECTION ( 'NONE',  ( 0.000000000000000000, 0.000000000000000000, -1.000000000000000000 ) ) ;
#27622=EDGE_CURVE ( 'NONE', #200, #89141, #76036, .T. ) ;
#27624=ORIENTED_EDGE ( 'NONE', *, *, #91412, .T. ) ;
#27631=EDGE_CURVE ( 'NONE', #59332, #86133, #61718, .T. ) ;
#27645=FACE_OUTER_BOUND ( 'NONE', #58084, .T. ) ;
#27648=CIRCLE ( 'NONE', #14065, 0.5000000000000004441 ) ;
#27654=CIRCLE ( 'NONE', #74538, 1.000000000000008882 ) ;
#27660=AXIS2_PLACEMENT_3D ( 'NONE', #36461, #78627, #86173 ) ;
#27665=ORIENTED_EDGE ( 'NONE', *, *, #11779, .F. ) ;
#27668=ORIENTED_EDGE ( 'NONE', *, *, #50647, .T. ) ;
#27688=VECTOR ( 'NONE', #1072, 1000.000000000000000 ) ;
#27694=ORIENTED_EDGE ( 'NONE', *, *, #92268, .F. ) ;
#27701=DIRECTION ( 'NONE',  ( 0.000000000000000000, 1.000000000000000000, 0.000000000000000000 ) ) ;
#27704=EDGE_CURVE ( 'NONE', #46837, #63636, #77924, .T. ) ;
#27707=FACE_OUTER_BOUND ( 'NONE', #88, .T. ) ;
#27708=AXIS2_PLACEMENT_3D ( 'NONE', #30260, #67653, #24080 ) ;
#27716=VECTOR ( 'NONE', #8706, 1000.000000000000000 ) ;
#27721=CARTESIAN_POINT ( 'NONE',  ( 175.2296996224750103, 275.0000000000000568, 0.000000000000000000 ) ) ;
#27723=AXIS2_PLACEMENT_3D ( 'NONE', #83974, #40389, #47977 ) ;
#27724=MANIFOLD_SOLID_BREP ( 'Boss-Extrude27', #58252 ) ;
#27730=DIRECTION ( 'NONE',  ( -0.2456588035076310295, 0.9693563597868428694, 0.000000000000000000 ) ) ;
#27733=AXIS2_PLACEMENT_3D ( 'NONE', #33287, #40826, #83943 ) ;
#27743=FACE_OUTER_BOUND ( 'NONE', #77258, .T. ) ;
#27747=DIRECTION ( 'NONE',  ( -1.000000000000000000, 0.000000000000000000, 0.000000000000000000 ) ) ;
#27767=ADVANCED_FACE ( 'NONE', ( #32379 ), #49394, .F. ) ;
#27788=CARTESIAN_POINT ( 'NONE',  ( 164.2231345125756263, 300.2961574867697436, -7.500000000000000000 ) ) ;
#27789=AXIS2_PLACEMENT_3D ( 'NONE', #1707, #44788, #81699 ) ;
#27790=FACE_OUTER_BOUND ( 'NONE', #88683, .T. ) ;
#27793=EDGE_LOOP ( 'NONE', ( #35681, #16712 ) ) ;
#27800=CIRCLE ( 'NONE', #5079, 9.550761578869391144 ) ;
#27803=VERTEX_POINT ( 'NONE', #50307 ) ;
#27808=LINE ( 'NONE', #19748, #80984 ) ;
#27809=CARTESIAN_POINT ( 'NONE',  ( 153.9133111279456045, 20.47222690886501795, -13.06183683676589524 ) ) ;
#27810=AXIS2_PLACEMENT_3D ( 'NONE', #63497, #69165, #69630 ) ;
#27812=DIRECTION ( 'NONE',  ( 0.000000000000000000, 0.000000000000000000, -1.000000000000000000 ) ) ;
#27813=TOROIDAL_SURFACE ( 'NONE', #89741, 1.500000000000000888, 0.5000000000000000000 ) ;
#27819=DIRECTION ( 'NONE',  ( 0.000000000000000000, 0.000000000000000000, 1.000000000000000000 ) ) ;
#27820=DIRECTION ( 'NONE',  ( 1.000000000000000000, -0.000000000000000000, -0.000000000000000000 ) ) ;
#27822=AXIS2_PLACEMENT_3D ( 'NONE', #5043, #54283, #83622 ) ;
#27823=ORIENTED_EDGE ( 'NONE', *, *, #26635, .F. ) ;
#27824=ORIENTED_EDGE ( 'NONE', *, *, #60993, .T. ) ;
#27827=EDGE_CURVE ( 'NONE', #29052, #11817, #72930, .T. ) ;
#27841=DIRECTION ( 'NONE',  ( -1.000000000000000000, 0.000000000000000000, 0.000000000000000000 ) ) ;
#27856=ADVANCED_FACE ( 'NONE', ( #65025 ), #20971, .T. ) ;
#27867=AXIS2_PLACEMENT_3D ( 'NONE', #59647, #31673, #81381 ) ;
#27870=CARTESIAN_POINT ( 'NONE',  ( 195.1853111624926385, 40.37665348939848542, 15.05924827439051406 ) ) ;
#27876=VECTOR ( 'NONE', #77752, 1000.000000000000114 ) ;
#27882=CARTESIAN_POINT ( 'NONE',  ( 197.2116943569230045, 215.0000000000000568, -12.42446933126075592 ) ) ;
#27885=CARTESIAN_POINT ( 'NONE',  ( 138.6539576904058606, 250.0000000000000568, 10.50000000000000000 ) ) ;
#27893=AXIS2_PLACEMENT_3D ( 'NONE', #49296, #25631, #13329 ) ;
#27895=ORIENTED_EDGE ( 'NONE', *, *, #1952, .F. ) ;
#27896=CARTESIAN_POINT ( 'NONE',  ( 195.4781563537916043, 39.36132622696000283, 14.00000000000000000 ) ) ;
#27900=ADVANCED_FACE ( 'NONE', ( #13878 ), #26067, .T. ) ;
#27902=EDGE_LOOP ( 'NONE', ( #63936, #20529, #68374, #62739, #28716 ) ) ;
#27908=CARTESIAN_POINT ( 'NONE',  ( 199.2174190867142727, 65.99980561011084035, -9.232127820537071372 ) ) ;
#27909=CYLINDRICAL_SURFACE ( 'NONE', #5450, 4.999999999999986677 ) ;
#27913=VERTEX_POINT ( 'NONE', #70708 ) ;
#27927=DIRECTION ( 'NONE',  ( 0.000000000000000000, 0.000000000000000000, 1.000000000000000000 ) ) ;
#27936=B_SPLINE_CURVE_WITH_KNOTS ( 'NONE', 3,
 ( #33875, #91617, #55657, #40012, #84510, #4060 ),
 .UNSPECIFIED., .F., .F.,
 ( 4, 2, 4 ),
 ( 1.115630864829514821E-16, 0.0006602105328823850783, 0.001320421065764658484 ),
 .UNSPECIFIED. ) ;
#27943=ORIENTED_EDGE ( 'NONE', *, *, #46281, .T. ) ;
#27944=CARTESIAN_POINT ( 'NONE',  ( 156.5191989162425727, 214.5000000000000568, 16.58062614384861178 ) ) ;
#27947=AXIS2_PLACEMENT_3D ( 'NONE', #43106, #87561, #87110 ) ;
#27959=DIRECTION ( 'NONE',  ( 0.000000000000000000, 0.000000000000000000, 1.000000000000000000 ) ) ;
#27962=VECTOR ( 'NONE', #78002, 1000.000000000000000 ) ;
#27969=DIRECTION ( 'NONE',  ( -0.000000000000000000, 1.000000000000000000, -0.000000000000000000 ) ) ;
#27971=CARTESIAN_POINT ( 'NONE',  ( 201.2104617360081704, 15.00000000000000000, -10.00000000000000000 ) ) ;
#27982=CARTESIAN_POINT ( 'NONE',  ( 200.1411370654279551, 66.37844756382011724, -9.866896536115095984 ) ) ;
#27993=DIRECTION ( 'NONE',  ( 0.000000000000000000, 0.000000000000000000, 1.000000000000000000 ) ) ;
#28007=TOROIDAL_SURFACE ( 'NONE', #11350, 1.000000000000000000, 0.5000000000000000000 ) ;
#28008=DIRECTION ( 'NONE',  ( 0.000000000000000000, 0.000000000000000000, 1.000000000000000000 ) ) ;
#28020=CIRCLE ( 'NONE', #64349, 0.5000000000000001110 ) ;
#28025=ORIENTED_EDGE ( 'NONE', *, *, #6914, .T. ) ;
#28035=CARTESIAN_POINT ( 'NONE',  ( 175.2296996224750103, 160.0000000000000568, 24.00000000000001066 ) ) ;
#28045=ORIENTED_EDGE ( 'NONE', *, *, #84612, .F. ) ;
#28052=EDGE_LOOP ( 'NONE', ( #5054, #55514, #80394, #81443 ) ) ;
#28053=CARTESIAN_POINT ( 'NONE',  ( 194.8650209881936064, 26.44696541833617687, 13.81479162729918997 ) ) ;
#28063=DIRECTION ( 'NONE',  ( -0.000000000000000000, -1.000000000000000000, -0.000000000000000000 ) ) ;
#28070=EDGE_CURVE ( 'NONE', #44324, #46709, #51752, .T. ) ;
#28072=EDGE_CURVE ( 'NONE', #75355, #76874, #63907, .T. ) ;
#28088=FACE_OUTER_BOUND ( 'NONE', #56696, .T. ) ;
#28092=CARTESIAN_POINT ( 'NONE',  ( 197.4027394742815602, 40.84896208771628068, 12.00000000000000000 ) ) ;
#28095=CARTESIAN_POINT ( 'NONE',  ( 157.4787282879766508, 15.38390992556615622, -9.006389530800271714 ) ) ;
#28105=ORIENTED_EDGE ( 'NONE', *, *, #30387, .T. ) ;
#28108=CARTESIAN_POINT ( 'NONE',  ( 197.5379522065468052, 276.0000000000000568, -11.97918851819043873 ) ) ;
#28133=DIRECTION ( 'NONE',  ( -0.000000000000000000, -1.000000000000000000, -0.000000000000000000 ) ) ;
#28140=ORIENTED_EDGE ( 'NONE', *, *, #41040, .F. ) ;
#28143=EDGE_LOOP ( 'NONE', ( #74531, #83062, #34521, #32904 ) ) ;
#28161=EDGE_LOOP ( 'NONE', ( #63326, #82721, #89690, #20690, #59841, #66887 ) ) ;
#28168=ORIENTED_EDGE ( 'NONE', *, *, #33819, .T. ) ;
#28170=ORIENTED_EDGE ( 'NONE', *, *, #17248, .F. ) ;
#28179=EDGE_CURVE ( 'NONE', #12173, #69141, #78735, .T. ) ;
#28183=DIRECTION ( 'NONE',  ( 0.000000000000000000, 0.000000000000000000, 1.000000000000000000 ) ) ;
#28189=CARTESIAN_POINT ( 'NONE',  ( 196.1963538710215857, 305.7026273589066250, 13.99999999999999112 ) ) ;
#28193=LINE ( 'NONE', #35279, #47398 ) ;
#28195=B_SPLINE_CURVE_WITH_KNOTS ( 'NONE', 3,
 ( #22932, #80235, #52732, #81615, #43772, #79774 ),
 .UNSPECIFIED., .F., .F.,
 ( 4, 2, 4 ),
 ( 0.000000000000000000, 0.0009572278725339521555, 0.001914455745067904311 ),
 .UNSPECIFIED. ) ;
#28197=CARTESIAN_POINT ( 'NONE',  ( 175.2296996224750103, 214.5000000000000568, 0.000000000000000000 ) ) ;
#28201=CARTESIAN_POINT ( 'NONE',  ( 199.7700033442230279, 63.22432295887224285, -10.15684170342041703 ) ) ;
#28213=CARTESIAN_POINT ( 'NONE',  ( 170.2331121529641678, 214.9642003054772488, -24.76688354601320441 ) ) ;
#28217=CARTESIAN_POINT ( 'NONE',  ( 186.6539576904058890, 293.9636489450775230, 11.60392986742922439 ) ) ;
#28254=CARTESIAN_POINT ( 'NONE',  ( 175.2296996224750103, 20.99999999999998934, -24.00000000000000355 ) ) ;
#28255=CARTESIAN_POINT ( 'NONE',  ( 153.5370352062773520, 129.8649369643340492, -11.69957875851211249 ) ) ;
#28271=ORIENTED_EDGE ( 'NONE', *, *, #26870, .T. ) ;
#28274=CARTESIAN_POINT ( 'NONE',  ( 154.2759627658477939, 20.32662787347680222, 12.20915505293938530 ) ) ;
#28282=DIRECTION ( 'NONE',  ( -0.000000000000000000, -1.000000000000000000, -0.000000000000000000 ) ) ;
#28283=ORIENTED_EDGE ( 'NONE', *, *, #20809, .F. ) ;
#28284=CARTESIAN_POINT ( 'NONE',  ( 208.0212563688061209, 27.56882951438707607, 12.00000000000000000 ) ) ;
#28287=EDGE_CURVE ( 'NONE', #40097, #42461, #29008, .T. ) ;
#28299=CARTESIAN_POINT ( 'NONE',  ( 196.2373416849518151, 25.97420206995995073, 13.14673451885373368 ) ) ;
#28300=CARTESIAN_POINT ( 'NONE',  ( 199.4392256788250677, 65.82574266882504332, 7.741079165001067963 ) ) ;
#28307=EDGE_CURVE ( 'NONE', #15166, #10282, #43215, .T. ) ;
#28316=DIRECTION ( 'NONE',  ( -1.000000000000000000, 0.000000000000000000, 0.000000000000000000 ) ) ;
#28323=CARTESIAN_POINT ( 'NONE',  ( 202.6689663790774887, 287.6799160531548409, -4.951217617476999955 ) ) ;
#28326=DIRECTION ( 'NONE',  ( 0.000000000000000000, 0.000000000000000000, -1.000000000000000000 ) ) ;
#28330=LINE ( 'NONE', #52297, #484 ) ;
#28340=CARTESIAN_POINT ( 'NONE',  ( 152.6996702291354211, 19.85642976176308139, 8.932053473883454942 ) ) ;
#28342=DIRECTION ( 'NONE',  ( -0.000000000000000000, -1.000000000000000000, -0.000000000000000000 ) ) ;
#28352=CARTESIAN_POINT ( 'NONE',  ( 194.2870706637141325, 39.36132622696000283, 14.58823529411764675 ) ) ;
#28363=CARTESIAN_POINT ( 'NONE',  ( 197.1861737955271963, 69.99861189218830759, -10.13991136371132207 ) ) ;
#28364=DIRECTION ( 'NONE',  ( 0.000000000000000000, 0.000000000000000000, -1.000000000000000000 ) ) ;
#28371=B_SPLINE_CURVE_WITH_KNOTS ( 'NONE', 3,
 ( #9671, #17258, #86518, #28788, #9191, #44722 ),
 .UNSPECIFIED., .F., .F.,
 ( 4, 2, 4 ),
 ( 0.0009696774721519553974, 0.002350549526938858821, 0.003731421581725762136 ),
 .UNSPECIFIED. ) ;
#28374=ORIENTED_EDGE ( 'NONE', *, *, #51069, .F. ) ;
#28382=EDGE_CURVE ( 'NONE', #4576, #6353, #79670, .T. ) ;
#28384=VERTEX_POINT ( 'NONE', #49387 ) ;
#28399=EDGE_LOOP ( 'NONE', ( #66064, #54902, #53377, #41976 ) ) ;
#28400=ORIENTED_EDGE ( 'NONE', *, *, #64378, .T. ) ;
#28401=CARTESIAN_POINT ( 'NONE',  ( 156.5854952678944301, 214.6009552038394759, 16.65543863426000470 ) ) ;
#28405=EDGE_CURVE ( 'NONE', #66586, #13010, #78279, .T. ) ;
#28416=DIRECTION ( 'NONE',  ( 0.000000000000000000, -1.000000000000000000, 0.000000000000000000 ) ) ;
#28417=DIRECTION ( 'NONE',  ( 0.000000000000000000, 0.000000000000000000, 1.000000000000000000 ) ) ;
#28436=CARTESIAN_POINT ( 'NONE',  ( 153.8801639287781313, 129.5385997557426947, 11.85807839311486411 ) ) ;
#28438=CARTESIAN_POINT ( 'NONE',  ( 199.1087447750284980, 64.61450673763175701, -10.46317447812566215 ) ) ;
#28449=ORIENTED_EDGE ( 'NONE', *, *, #9944, .T. ) ;
#28452=CARTESIAN_POINT ( 'NONE',  ( 151.4851178187871312, 21.00000000000000000, 3.492110388858666870 ) ) ;
#28466=DIRECTION ( 'NONE',  ( 0.000000000000000000, 0.000000000000000000, 1.000000000000000000 ) ) ;
#28468=TOROIDAL_SURFACE ( 'NONE', #26904, 25.50000000000000355, 0.5000000000000000000 ) ;
#28486=EDGE_LOOP ( 'NONE', ( #2363, #28727, #22403, #71357 ) ) ;
#28487=ORIENTED_EDGE ( 'NONE', *, *, #9225, .T. ) ;
#28493=DIRECTION ( 'NONE',  ( 0.000000000000000000, 0.000000000000000000, 1.000000000000000000 ) ) ;
#28505=EDGE_LOOP ( 'NONE', ( #70059, #71493, #11478, #3377 ) ) ;
#28506=CYLINDRICAL_SURFACE ( 'NONE', #24657, 4.999999999999990230 ) ;
#28527=ADVANCED_FACE ( 'NONE', ( #52163, #87210 ), #45985, .F. ) ;
#28532=EDGE_CURVE ( 'NONE', #52326, #15079, #9531, .T. ) ;
#28535=VECTOR ( 'NONE', #38336, 1000.000000000000000 ) ;
#28548=DIRECTION ( 'NONE',  ( -0.8195702660916324156, 0.000000000000000000, -0.5729786897769331144 ) ) ;
#28558=ORIENTED_EDGE ( 'NONE', *, *, #79777, .F. ) ;
#28561=LINE ( 'NONE', #86762, #27688 ) ;
#28579=LINE ( 'NONE', #86312, #68192 ) ;
#28586=ADVANCED_FACE ( 'NONE', ( #67325 ), #22358, .T. ) ;
#28604=AXIS2_PLACEMENT_3D ( 'NONE', #45152, #37590, #9170 ) ;
#28625=ORIENTED_EDGE ( 'NONE', *, *, #5917, .F. ) ;
#28640=CARTESIAN_POINT ( 'NONE',  ( 221.8344101925596306, 0.000000000000000000, -7.000000000000000888 ) ) ;
#28646=DIRECTION ( 'NONE',  ( -1.000000000000000000, 0.000000000000000000, 0.000000000000000000 ) ) ;
#28650=LINE ( 'NONE', #6405, #88236 ) ;
#28654=DIRECTION ( 'NONE',  ( -1.000000000000000000, 0.000000000000000000, 0.000000000000000000 ) ) ;
#28658=DIRECTION ( 'NONE',  ( 0.9693563597868429804, 0.2456588035076310572, 7.238107246010827522E-15 ) ) ;
#28669=CIRCLE ( 'NONE', #22631, 6.286090667950827715 ) ;
#28671=CARTESIAN_POINT ( 'NONE',  ( 175.2296996224750103, 250.0000000000000568, 0.000000000000000000 ) ) ;
#28711=CARTESIAN_POINT ( 'NONE',  ( 160.5350683151633291, 249.5000000000000568, 20.22542485937379908 ) ) ;
#28716=ORIENTED_EDGE ( 'NONE', *, *, #21995, .F. ) ;
#28727=ORIENTED_EDGE ( 'NONE', *, *, #43406, .T. ) ;
#28729=DIRECTION ( 'NONE',  ( 0.000000000000000000, 0.000000000000000000, 1.000000000000000000 ) ) ;
#28732=CARTESIAN_POINT ( 'NONE',  ( 156.1965750133393271, 18.75975317436940415, 8.718057073926352984 ) ) ;
#28735=AXIS2_PLACEMENT_3D ( 'NONE', #63922, #427, #50139 ) ;
#28740=CARTESIAN_POINT ( 'NONE',  ( 175.2296996224750103, 15.00000000000000000, -15.00000000000000000 ) ) ;
#28742=CARTESIAN_POINT ( 'NONE',  ( 164.7144138485119242, 214.9642006536927568, 22.97375162482067168 ) ) ;
#28744=ORIENTED_EDGE ( 'NONE', *, *, #29988, .T. ) ;
#28759=DIRECTION ( 'NONE',  ( 0.000000000000000000, 0.000000000000000000, 1.000000000000000000 ) ) ;
#28760=DIRECTION ( 'NONE',  ( -0.000000000000000000, -1.000000000000000000, -0.000000000000000000 ) ) ;
#28773=CARTESIAN_POINT ( 'NONE',  ( 154.7659666677360235, 19.56018909072649237, -12.94946946942526189 ) ) ;
#28782=CARTESIAN_POINT ( 'NONE',  ( 196.7383257810085695, 42.27872732282707346, 11.00000000000001243 ) ) ;
#28785=FACE_OUTER_BOUND ( 'NONE', #89706, .T. ) ;
#28788=CARTESIAN_POINT ( 'NONE',  ( 155.8725544043047080, 19.96731923950699894, -14.33077026901615803 ) ) ;
#28796=EDGE_CURVE ( 'NONE', #45831, #69300, #62102, .T. ) ;
#28797=VECTOR ( 'NONE', #80839, 1000.000000000000000 ) ;
#28800=ORIENTED_EDGE ( 'NONE', *, *, #44642, .T. ) ;
#28801=DIRECTION ( 'NONE',  ( 0.000000000000000000, 0.000000000000000000, 1.000000000000000000 ) ) ;
#28813=VERTEX_POINT ( 'NONE', #80120 ) ;
#28814=CARTESIAN_POINT ( 'NONE',  ( 194.9397804919432247, 41.66501297569659101, 13.69433569849578802 ) ) ;
#28819=EDGE_CURVE ( 'NONE', #60748, #45831, #1508, .T. ) ;
#28821=ORIENTED_EDGE ( 'NONE', *, *, #17291, .T. ) ;
#28828=FACE_OUTER_BOUND ( 'NONE', #23228, .T. ) ;
#28829=CARTESIAN_POINT ( 'NONE',  ( 138.6539576904058606, 130.8284271247462414, -11.67157287525380838 ) ) ;
#28838=ORIENTED_EDGE ( 'NONE', *, *, #82958, .F. ) ;
#28847=CARTESIAN_POINT ( 'NONE',  ( 222.0386546523673985, 36.13108063356137478, 7.000000000000000000 ) ) ;
#28861=VERTEX_POINT ( 'NONE', #23290 ) ;
#28876=CARTESIAN_POINT ( 'NONE',  ( 200.2296996224750103, 68.12454877777268791, -4.440892098500626793E-14 ) ) ;
#28877=CARTESIAN_POINT ( 'NONE',  ( 164.6148405695019505, 214.9970011440366875, 23.11617803653516035 ) ) ;
#28886=CARTESIAN_POINT ( 'NONE',  ( 151.4851178187871312, 20.00000000000000000, -3.492110388858666870 ) ) ;
#28897=CARTESIAN_POINT ( 'NONE',  ( 153.5370352062774089, 129.8649369643341061, 11.69957875851211959 ) ) ;
#28900=CARTESIAN_POINT ( 'NONE',  ( 198.5955908591174648, 68.60853014440941422, -10.61435496113653443 ) ) ;
#28901=CARTESIAN_POINT ( 'NONE',  ( 207.7039919494849016, 30.29338434242851363, 15.02863188060213773 ) ) ;
#28912=CARTESIAN_POINT ( 'NONE',  ( 201.2104617360081704, 69.18068689461284748, -10.00000000000000000 ) ) ;
#28927=ADVANCED_FACE ( 'NONE', ( #37935 ), #37034, .T. ) ;
#28928=DIRECTION ( 'NONE',  ( 0.000000000000000000, 0.000000000000000000, -1.000000000000000000 ) ) ;
#28941=ORIENTED_EDGE ( 'NONE', *, *, #61608, .F. ) ;
#28948=VERTEX_POINT ( 'NONE', #1059 ) ;
#28949=ORIENTED_EDGE ( 'NONE', *, *, #48544, .T. ) ;
#28955=CARTESIAN_POINT ( 'NONE',  ( 200.3186454232214828, 250.0000000000000568, -3.421094783296261710 ) ) ;
#28995=CIRCLE ( 'NONE', #12354, 0.4999999999999996114 ) ;
#29001=CARTESIAN_POINT ( 'NONE',  ( 209.4593673012390127, 36.32691179220002198, 14.77866956795211273 ) ) ;
#29002=AXIS2_PLACEMENT_3D ( 'NONE', #43885, #66163, #45736 ) ;
#29007=CARTESIAN_POINT ( 'NONE',  ( 164.7123623445222904, 3.000000000000000000, 10.00000000000000178 ) ) ;
#29008=LINE ( 'NONE', #72561, #21627 ) ;
#29020=CARTESIAN_POINT ( 'NONE',  ( 197.2369698562987992, 24.81718856582945776, 11.94944555321362500 ) ) ;
#29022=EDGE_LOOP ( 'NONE', ( #10470, #67848, #1361, #77970, #29205 ) ) ;
#29030=VERTEX_POINT ( 'NONE', #89523 ) ;
#29049=EDGE_CURVE ( 'NONE', #66900, #60939, #24687, .T. ) ;
#29052=VERTEX_POINT ( 'NONE', #69643 ) ;
#29055=ORIENTED_EDGE ( 'NONE', *, *, #33498, .T. ) ;
#29058=EDGE_CURVE ( 'NONE', #48695, #78455, #27654, .T. ) ;
#29065=CIRCLE ( 'NONE', #330, 0.4999999999999922839 ) ;
#29076=VECTOR ( 'NONE', #20970, 1000.000000000000000 ) ;
#29083=ORIENTED_EDGE ( 'NONE', *, *, #70067, .F. ) ;
#29095=FACE_OUTER_BOUND ( 'NONE', #56992, .T. ) ;
#29106=CARTESIAN_POINT ( 'NONE',  ( 155.7140808774799723, 20.00000000000000355, 15.62500000000000000 ) ) ;
#29110=CARTESIAN_POINT ( 'NONE',  ( 214.2238915819278589, 32.98517505407394168, 10.50000000000000000 ) ) ;
#29113=DIRECTION ( 'NONE',  ( 0.000000000000000000, 1.000000000000000000, 0.000000000000000000 ) ) ;
#29117=CARTESIAN_POINT ( 'NONE',  ( 198.7793562774353404, 65.30699008317354526, -10.61576606199975714 ) ) ;
#29167=EDGE_CURVE ( 'NONE', #74948, #9812, #7963, .T. ) ;
#29173=DIRECTION ( 'NONE',  ( 0.7957555401921969640, 0.6056179655966498210, 0.000000000000000000 ) ) ;
#29189=CARTESIAN_POINT ( 'NONE',  ( 196.4697998462662270, 24.53660424933035600, 13.19104620540694306 ) ) ;
#29190=TOROIDAL_SURFACE ( 'NONE', #62522, 1.000000000000000000, 0.5000000000000000000 ) ;
#29193=AXIS2_PLACEMENT_3D ( 'NONE', #82520, #10539, #3444 ) ;
#29199=CARTESIAN_POINT ( 'NONE',  ( 209.8744251295252070, 28.03846817292547655, 13.95110425196124737 ) ) ;
#29202=LINE ( 'NONE', #6504, #11176 ) ;
#29205=ORIENTED_EDGE ( 'NONE', *, *, #34990, .T. ) ;
#29206=CARTESIAN_POINT ( 'NONE',  ( 208.6392664839860061, 27.72544851617926298, 12.02381566707519944 ) ) ;
#29208=CIRCLE ( 'NONE', #77605, 0.5000000000000003331 ) ;
#29218=CIRCLE ( 'NONE', #82122, 24.99999999999999645 ) ;
#29221=CARTESIAN_POINT ( 'NONE',  ( 197.0002228694559960, 291.9912828655285466, -7.756604549753964406 ) ) ;
#29223=EDGE_CURVE ( 'NONE', #72640, #66586, #83839, .T. ) ;
#29238=CARTESIAN_POINT ( 'NONE',  ( 197.8477145984406889, 64.61450673763175701, 7.741079165001056417 ) ) ;
#29240=CARTESIAN_POINT ( 'NONE',  ( 208.6208076322478746, 32.98517505407394168, 14.69807322781335657 ) ) ;
#29246=CARTESIAN_POINT ( 'NONE',  ( 196.1970748449012376, 41.31174257127814542, 11.68933045232663659 ) ) ;
#29258=AXIS2_PLACEMENT_3D ( 'NONE', #38153, #23508, #66147 ) ;
#29265=DIRECTION ( 'NONE',  ( 1.000000000000000000, -0.000000000000000000, 0.000000000000000000 ) ) ;
#29266=AXIS2_PLACEMENT_3D ( 'NONE', #37447, #51649, #37902 ) ;
#29278=EDGE_LOOP ( 'NONE', ( #72356, #12541, #22828 ) ) ;
#29279=CARTESIAN_POINT ( 'NONE',  ( 195.8903875302077893, 41.38157328953137437, 12.21596753353894549 ) ) ;
#29291=CARTESIAN_POINT ( 'NONE',  ( 196.7846939763287821, 69.56630120087481828, -10.93783953956503652 ) ) ;
#29292=DIRECTION ( 'NONE',  ( 0.000000000000000000, 0.000000000000000000, 1.000000000000000000 ) ) ;
#29296=ORIENTED_EDGE ( 'NONE', *, *, #43478, .F. ) ;
#29304=ORIENTED_EDGE ( 'NONE', *, *, #3303, .F. ) ;
#29316=AXIS2_PLACEMENT_3D ( 'NONE', #20071, #71216, #48469 ) ;
#29329=VERTEX_POINT ( 'NONE', #76747 ) ;
#29330=CARTESIAN_POINT ( 'NONE',  ( 175.2296996224750103, 249.5000000000000568, 0.000000000000000000 ) ) ;
#29336=EDGE_CURVE ( 'NONE', #13609, #11375, #54861, .T. ) ;
#29340=VECTOR ( 'NONE', #69848, 1000.000000000000114 ) ;
#29346=DIRECTION ( 'NONE',  ( 0.000000000000000000, 0.000000000000000000, 1.000000000000000000 ) ) ;
#29347=ADVANCED_FACE ( 'NONE', ( #32256 ), #82894, .T. ) ;
#29357=AXIS2_PLACEMENT_3D ( 'NONE', #50185, #79082, #21793 ) ;
#29358=CIRCLE ( 'NONE', #83732, 0.4999999999999989453 ) ;
#29362=DIRECTION ( 'NONE',  ( -0.000000000000000000, -1.000000000000000000, -0.000000000000000000 ) ) ;
#29365=VECTOR ( 'NONE', #85336, 1000.000000000000000 ) ;
#29371=DIRECTION ( 'NONE',  ( -0.000000000000000000, -0.000000000000000000, -1.000000000000000000 ) ) ;
#29383=DIRECTION ( 'NONE',  ( 0.000000000000000000, -1.000000000000000000, 0.000000000000000000 ) ) ;
#29398=CYLINDRICAL_SURFACE ( 'NONE', #82335, 4.999999999999990230 ) ;
#29399=DIRECTION ( 'NONE',  ( 0.000000000000000000, 0.000000000000000000, 1.000000000000000000 ) ) ;
#29402=AXIS2_PLACEMENT_3D ( 'NONE', #83456, #68342, #60779 ) ;
#29412=ORIENTED_EDGE ( 'NONE', *, *, #11598, .F. ) ;
#29421=ORIENTED_EDGE ( 'NONE', *, *, #70753, .T. ) ;
#29427=DIRECTION ( 'NONE',  ( 0.3262578496237564796, 0.000000000000000000, 0.9452808130703185263 ) ) ;
#29440=EDGE_LOOP ( 'NONE', ( #63428, #20319, #43522, #20586 ) ) ;
#29441=EDGE_CURVE ( 'NONE', #16112, #86133, #17094, .T. ) ;
#29442=CARTESIAN_POINT ( 'NONE',  ( 196.1797262162750712, 26.01001517850438560, 13.20229404944032048 ) ) ;
#29444=AXIS2_PLACEMENT_3D ( 'NONE', #7055, #12763, #86554 ) ;
#29447=EDGE_CURVE ( 'NONE', #83522, #20445, #3847, .T. ) ;
#29457=DIRECTION ( 'NONE',  ( 0.000000000000000000, 0.000000000000000000, 1.000000000000000000 ) ) ;
#29470=CARTESIAN_POINT ( 'NONE',  ( 195.3067512911517554, 24.77037501708018041, 13.15092252244243731 ) ) ;
#29476=CARTESIAN_POINT ( 'NONE',  ( 197.2116943569230330, 275.5000000000000568, -11.92446933126074882 ) ) ;
#29478=( BOUNDED_SURFACE ( )  B_SPLINE_SURFACE ( 3, 2, ( 
 ( #79844, #14984, #86939 ),
 ( #36286, #309, #22091 ),
 ( #29189, #50961, #43840 ),
 ( #7405, #55374, #10855 ),
 ( #46371, #83761, #40189 ),
 ( #54416, #18433, #2838 ),
 ( #62001, #83287, #75731 ),
 ( #77141, #62482, #32659 ),
 ( #11337, #69108, #90380 ),
 ( #54882, #82371, #89449 ),
 ( #47290, #10390, #39255 ),
 ( #25997, #90836, #60611 ),
 ( #69568, #61547, #41115 ),
 ( #3774, #61086, #33573 ) ),
 .UNSPECIFIED., .F., .F., .F. ) 
 B_SPLINE_SURFACE_WITH_KNOTS ( ( 4, 2, 2, 2, 2, 2, 4 ),
 ( 3, 3 ),
 ( -2.168404344971008868E-19, 0.001236320232021350871, 0.001854480348032026523, 0.002472640464042702175, 0.003090800580053378044, 0.003708960696064053479, 0.004945280928085404350 ),
 ( 0.000000000000000000, 1.000000000000000000 ),
 .UNSPECIFIED. ) 
 GEOMETRIC_REPRESENTATION_ITEM ( )  RATIONAL_B_SPLINE_SURFACE ( (
 ( 1.000000000000000000, 0.8108476219622878789, 1.000000000000000000),
 ( 1.000000000000000000, 0.8255659973181316280, 1.000000000000000000),
 ( 1.000000000000000000, 0.8395011523844640999, 1.000000000000000000),
 ( 1.000000000000000000, 0.8588211550359595714, 1.000000000000000000),
 ( 1.000000000000000000, 0.8649348442247276614, 1.000000000000000000),
 ( 1.000000000000000000, 0.8760455507363352767, 1.000000000000000000),
 ( 1.000000000000000000, 0.8810998449843068236, 1.000000000000000000),
 ( 1.000000000000000000, 0.8900036393297112713, 1.000000000000000000),
 ( 1.000000000000000000, 0.8938622710284911399, 1.000000000000000000),
 ( 1.000000000000000000, 0.8997338558210890014, 1.000000000000000000),
 ( 1.000000000000000000, 0.9018082123496811153, 1.000000000000000000),
 ( 1.000000000000000000, 0.9050182246966690380, 1.000000000000000000),
 ( 1.000000000000000000, 0.9029724514273207436, 1.000000000000000000),
 ( 1.000000000000000000, 0.8966167345234181685, 1.000000000000000000) ) ) 
 REPRESENTATION_ITEM ( '' )  SURFACE ( )  );
#29479=CARTESIAN_POINT ( 'NONE',  ( 209.4803090767392462, 35.69423656899339647, 14.26380412667038833 ) ) ;
#29482=CARTESIAN_POINT ( 'NONE',  ( 204.6539576904058606, 300.0210572133868823, 3.999999999999991562 ) ) ;
#29489=( BOUNDED_CURVE ( )  B_SPLINE_CURVE ( 3, ( #69392, #19666, #48064, #76506 ),
 .UNSPECIFIED., .F., .F. ) 
 B_SPLINE_CURVE_WITH_KNOTS ( ( 4, 4 ),
 ( 5.759586531581287971, 6.283185307179586232 ),
 .UNSPECIFIED. ) 
 CURVE ( )  GEOMETRIC_REPRESENTATION_ITEM ( )  RATIONAL_B_SPLINE_CURVE ( ( 1.000000000000000000, 0.9772838841927120601, 0.9772838841927120601, 1.000000000000000000 ) ) 
 REPRESENTATION_ITEM ( '' )  );
#29494=ORIENTED_EDGE ( 'NONE', *, *, #43350, .T. ) ;
#29497=CARTESIAN_POINT ( 'NONE',  ( 196.8928068234201021, 24.78327594025822478, 12.47839767815188772 ) ) ;
#29499=AXIS2_PLACEMENT_3D ( 'NONE', #35349, #41959, #85055 ) ;
#29508=ORIENTED_EDGE ( 'NONE', *, *, #61091, .F. ) ;
#29513=DIRECTION ( 'NONE',  ( -1.000000000000000000, 0.000000000000000000, 0.000000000000000000 ) ) ;
#29517=FACE_OUTER_BOUND ( 'NONE', #81114, .T. ) ;
#29560=ORIENTED_EDGE ( 'NONE', *, *, #75324, .T. ) ;
#29574=LINE ( 'NONE', #64653, #60830 ) ;
#29580=DIRECTION ( 'NONE',  ( -0.000000000000000000, -0.000000000000000000, 1.000000000000000000 ) ) ;
#29582=EDGE_CURVE ( 'NONE', #57029, #85724, #15923, .T. ) ;
#29587=DIRECTION ( 'NONE',  ( 0.000000000000000000, 0.000000000000000000, 1.000000000000000000 ) ) ;
#29590=CARTESIAN_POINT ( 'NONE',  ( 151.4990408432631739, 130.0000000000000568, 12.49999999999999289 ) ) ;
#29592=CARTESIAN_POINT ( 'NONE',  ( 154.7156223832750186, 19.57420759269872690, -12.98093464719507395 ) ) ;
#29603=EDGE_CURVE ( 'NONE', #64179, #84307, #51819, .T. ) ;
#29646=ADVANCED_FACE ( 'NONE', ( #9373 ), #73797, .T. ) ;
#29667=DIRECTION ( 'NONE',  ( -0.000000000000000000, 1.000000000000000000, -0.000000000000000000 ) ) ;
#29673=CARTESIAN_POINT ( 'NONE',  ( 207.9416365392708883, 29.59756043702767769, 14.84194439653736630 ) ) ;
#29674=CARTESIAN_POINT ( 'NONE',  ( 154.4601611254704494, 20.78894139178057543, 13.92477262272432625 ) ) ;
#29676=EDGE_LOOP ( 'NONE', ( #16566, #92275, #43042, #40209 ) ) ;
#29680=CARTESIAN_POINT ( 'NONE',  ( 199.1510190623362462, 40.29428703769173126, 9.290748352207996774 ) ) ;
#29694=CARTESIAN_POINT ( 'NONE',  ( 208.8914842347286367, 1.063508326896293932, -7.500000000000007105 ) ) ;
#29697=EDGE_CURVE ( 'NONE', #51603, #63777, #91133, .T. ) ;
#29704=CARTESIAN_POINT ( 'NONE',  ( 0.000000000000000000, 0.000000000000000000, 7.500000000000000000 ) ) ;
#29709=EDGE_CURVE ( 'NONE', #90266, #82861, #59065, .T. ) ;
#29710=DIRECTION ( 'NONE',  ( 0.000000000000000000, 1.000000000000000000, 0.000000000000000000 ) ) ;
#29718=CARTESIAN_POINT ( 'NONE',  ( 208.8121973762197854, 29.40831337191700712, 14.72017627883221813 ) ) ;
#29721=CARTESIAN_POINT ( 'NONE',  ( 188.2019740231993410, 44.81720372851549428, 15.00000000000000000 ) ) ;
#29735=CARTESIAN_POINT ( 'NONE',  ( 222.8344101925596306, 0.000000000000000000, -7.000000000000000888 ) ) ;
#29737=CARTESIAN_POINT ( 'NONE',  ( 175.2296996224750103, 247.0000000000001137, 0.000000000000000000 ) ) ;
#29746=ORIENTED_EDGE ( 'NONE', *, *, #22620, .T. ) ;
#29757=DIRECTION ( 'NONE',  ( 0.000000000000000000, 1.000000000000000000, 0.000000000000000000 ) ) ;
#29767=EDGE_CURVE ( 'NONE', #40624, #8082, #23605, .T. ) ;
#29781=DIRECTION ( 'NONE',  ( 0.000000000000000000, 1.000000000000000000, 0.000000000000000000 ) ) ;
#29795=CARTESIAN_POINT ( 'NONE',  ( 196.0143093133015952, 19.33012701892214480, -12.49999999999990941 ) ) ;
#29801=ADVANCED_FACE ( 'NONE', ( #67632 ), #88066, .T. ) ;
#29820=DIRECTION ( 'NONE',  ( -0.2456588035076310295, 0.9693563597868428694, 0.000000000000000000 ) ) ;
#29843=ORIENTED_EDGE ( 'NONE', *, *, #93160, .T. ) ;
#29847=DIRECTION ( 'NONE',  ( 0.000000000000000000, 0.000000000000000000, 1.000000000000000000 ) ) ;
#29850=ADVANCED_FACE ( 'NONE', ( #46292 ), #75196, .T. ) ;
#29857=EDGE_LOOP ( 'NONE', ( #3411, #64395, #55491, #62493 ) ) ;
#29860=CARTESIAN_POINT ( 'NONE',  ( 200.4892204403987250, 64.44609543878978286, -7.254661561165810291 ) ) ;
#29861=FACE_OUTER_BOUND ( 'NONE', #46487, .T. ) ;
#29864=CARTESIAN_POINT ( 'NONE',  ( 208.6208076322478746, 32.98517505407394168, 9.000000000000001776 ) ) ;
#29868=EDGE_CURVE ( 'NONE', #39851, #4210, #12568, .T. ) ;
#29883=ORIENTED_EDGE ( 'NONE', *, *, #80555, .T. ) ;
#29889=FACE_OUTER_BOUND ( 'NONE', #48367, .T. ) ;
#29901=ORIENTED_EDGE ( 'NONE', *, *, #54992, .T. ) ;
#29902=CARTESIAN_POINT ( 'NONE',  ( 194.5542095385274592, 25.91226055734863465, 14.23298358910922445 ) ) ;
#29912=DIRECTION ( 'NONE',  ( 0.000000000000000000, -1.000000000000000000, 0.000000000000000000 ) ) ;
#29926=CARTESIAN_POINT ( 'NONE',  ( 195.0179948445400271, 25.07543301046760931, 13.58130950507239731 ) ) ;
#29932=CARTESIAN_POINT ( 'NONE',  ( 197.4836817735085219, 24.47698789593438917, 11.66666666666666785 ) ) ;
#29934=FACE_OUTER_BOUND ( 'NONE', #77397, .T. ) ;
#29937=DIRECTION ( 'NONE',  ( 0.1455045995357758803, 0.000000000000000000, -0.9893575751536618501 ) ) ;
#29938=CARTESIAN_POINT ( 'NONE',  ( 0.000000000000000000, 0.000000000000000000, 9.000000000000001776 ) ) ;
#29948=ORIENTED_EDGE ( 'NONE', *, *, #85740, .F. ) ;
#29949=DIRECTION ( 'NONE',  ( -1.000000000000000000, 0.000000000000000000, 0.000000000000000000 ) ) ;
#29952=LINE ( 'NONE', #13430, #47299 ) ;
#29964=CARTESIAN_POINT ( 'NONE',  ( 156.0793278192250284, 19.12150670425092258, 12.12861874973152609 ) ) ;
#29968=CYLINDRICAL_SURFACE ( 'NONE', #72727, 25.00000000000000355 ) ;
#29982=ORIENTED_EDGE ( 'NONE', *, *, #84181, .T. ) ;
#29985=ORIENTED_EDGE ( 'NONE', *, *, #47895, .T. ) ;
#29988=EDGE_CURVE ( 'NONE', #72022, #70265, #89445, .T. ) ;
#30005=EDGE_LOOP ( 'NONE', ( #20468, #40087 ) ) ;
#30011=EDGE_CURVE ( 'NONE', #44324, #69962, #2345, .T. ) ;
#30016=VERTEX_POINT ( 'NONE', #84149 ) ;
#30018=AXIS2_PLACEMENT_3D ( 'NONE', #70813, #18266, #69864 ) ;
#30033=LINE ( 'NONE', #220, #92848 ) ;
#30034=( BOUNDED_SURFACE ( )  B_SPLINE_SURFACE ( 3, 2, ( 
 ( #61704, #40351, #32814 ),
 ( #11967, #25696, #34225 ),
 ( #69268, #91960, #40815 ),
 ( #25243, #69732, #55062 ),
 ( #76840, #19537, #82990 ),
 ( #27115, #54117, #4397 ) ),
 .UNSPECIFIED., .F., .F., .F. ) 
 B_SPLINE_SURFACE_WITH_KNOTS ( ( 4, 2, 4 ),
 ( 3, 3 ),
 ( 2.168404344971008868E-19, 0.001011634320662447954, 0.002023268641324895908 ),
 ( 0.000000000000000000, 1.000000000000000000 ),
 .UNSPECIFIED. ) 
 GEOMETRIC_REPRESENTATION_ITEM ( )  RATIONAL_B_SPLINE_SURFACE ( (
 ( 1.000000000000000000, 0.5021841165015733521, 1.000000000000000000),
 ( 1.000000000000000000, 0.5023663462998690932, 1.000000000000000000),
 ( 1.000000000000000000, 0.5117996075019977109, 1.000000000000000000),
 ( 1.000000000000000000, 0.5521543867336666800, 1.000000000000000000),
 ( 1.000000000000000000, 0.5833157748965640543, 1.000000000000000000),
 ( 1.000000000000000000, 0.6287211027133851049, 1.000000000000000000) ) ) 
 REPRESENTATION_ITEM ( '' )  SURFACE ( )  );
#30040=DIRECTION ( 'NONE',  ( 1.000000000000000000, 0.000000000000000000, 0.000000000000000000 ) ) ;
#30043=CARTESIAN_POINT ( 'NONE',  ( 193.9646936176702070, 20.00000000000000000, 15.00000000000000000 ) ) ;
#30045=CARTESIAN_POINT ( 'NONE',  ( 155.7883889513935856, 17.75303870060648848, -10.69672886740455198 ) ) ;
#30078=EDGE_CURVE ( 'NONE', #52100, #15639, #19297, .T. ) ;
#30098=EDGE_CURVE ( 'NONE', #11198, #90976, #28995, .T. ) ;
#30099=ADVANCED_FACE ( 'NONE', ( #41032 ), #72854, .T. ) ;
#30105=CARTESIAN_POINT ( 'NONE',  ( 175.2296996224750103, 20.99999999999998934, 0.000000000000000000 ) ) ;
#30119=EDGE_LOOP ( 'NONE', ( #85209, #12735, #25616, #60863 ) ) ;
#30120=CYLINDRICAL_SURFACE ( 'NONE', #71966, 7.500000000000013323 ) ;
#30122=B_SPLINE_CURVE_WITH_KNOTS ( 'NONE', 3,
 ( #27358, #86965, #56246, #85575 ),
 .UNSPECIFIED., .F., .F.,
 ( 4, 4 ),
 ( 6.938893903907228378E-18, 0.001032852107770759233 ),
 .UNSPECIFIED. ) ;
#30126=CARTESIAN_POINT ( 'NONE',  ( 180.7287904564219332, 276.0000000000000568, -24.90000000000003411 ) ) ;
#30133=CARTESIAN_POINT ( 'NONE',  ( 210.7238915819278589, 32.98517505407394168, 12.09245862095555601 ) ) ;
#30146=CARTESIAN_POINT ( 'NONE',  ( 152.6876711748310242, 19.85946110189832581, 8.896468494892323164 ) ) ;
#30155=CARTESIAN_POINT ( 'NONE',  ( 196.0143093133015384, 19.33012701892218743, 12.49999999999999112 ) ) ;
#30159=ADVANCED_FACE ( 'NONE', ( #69959 ), #32104, .F. ) ;
#30161=DIRECTION ( 'NONE',  ( 0.000000000000000000, 0.000000000000000000, 1.000000000000000000 ) ) ;
#30186=CARTESIAN_POINT ( 'NONE',  ( 151.4851178187871312, 21.00000000000000000, 3.492110388858666870 ) ) ;
#30198=CARTESIAN_POINT ( 'NONE',  ( 207.5863589332323329, 29.28491128719180026, 13.57731244650625513 ) ) ;
#30208=DIRECTION ( 'NONE',  ( 0.000000000000000000, 1.000000000000000000, 0.000000000000000000 ) ) ;
#30210=AXIS2_PLACEMENT_3D ( 'NONE', #11982, #40365, #31898 ) ;
#30213=VERTEX_POINT ( 'NONE', #33980 ) ;
#30221=ADVANCED_FACE ( 'NONE', ( #62883 ), #65320, .T. ) ;
#30229=ADVANCED_FACE ( 'NONE', ( #12679 ), #10777, .T. ) ;
#30231=CARTESIAN_POINT ( 'NONE',  ( 156.9186804554042283, 250.2122328390418602, 16.89624193607524205 ) ) ;
#30232=DIRECTION ( 'NONE',  ( 0.3024135303179485423, 0.9531768234071972268, 0.000000000000000000 ) ) ;
#30240=DIRECTION ( 'NONE',  ( -1.000000000000000000, 0.000000000000000000, 0.000000000000000000 ) ) ;
#30244=VERTEX_POINT ( 'NONE', #83211 ) ;
#30246=CARTESIAN_POINT ( 'NONE',  ( 201.2104617360081704, 15.00000000000001243, -10.00000000000000178 ) ) ;
#30259=CARTESIAN_POINT ( 'NONE',  ( 196.8208173705680224, 214.5799893323897152, -12.60277379099805195 ) ) ;
#30260=CARTESIAN_POINT ( 'NONE',  ( 201.2104617360081704, 250.0000000000000568, 15.00000000000000000 ) ) ;
#30268=CYLINDRICAL_SURFACE ( 'NONE', #92709, 0.5000000000000004441 ) ;
#30272=FACE_OUTER_BOUND ( 'NONE', #74574, .T. ) ;
#30280=AXIS2_PLACEMENT_3D ( 'NONE', #48260, #40210, #84714 ) ;
#30283=ADVANCED_FACE ( 'NONE', ( #47217 ), #44106, .T. ) ;
#30290=DIRECTION ( 'NONE',  ( -1.000000000000000000, 0.000000000000000000, 0.000000000000000000 ) ) ;
#30301=CARTESIAN_POINT ( 'NONE',  ( 200.5815643859949944, 65.97596549932491428, -9.780880230328994784 ) ) ;
#30312=EDGE_LOOP ( 'NONE', ( #42417, #79238, #20796, #16453 ) ) ;
#30316=CARTESIAN_POINT ( 'NONE',  ( 196.8803347170859865, 250.0000000000000568, 12.49999999999999289 ) ) ;
#30319=CARTESIAN_POINT ( 'NONE',  ( 195.4781563537916043, 32.98517505407394168, 13.99999999999999822 ) ) ;
#30328=VERTEX_POINT ( 'NONE', #58098 ) ;
#30336=ORIENTED_EDGE ( 'NONE', *, *, #1737, .T. ) ;
#30338=AXIS2_PLACEMENT_3D ( 'NONE', #81171, #66519, #53703 ) ;
#30344=CARTESIAN_POINT ( 'NONE',  ( 175.2296996224750103, 249.5000000000000568, 0.000000000000000000 ) ) ;
#30356=ORIENTED_EDGE ( 'NONE', *, *, #22221, .F. ) ;
#30357=DIRECTION ( 'NONE',  ( 0.000000000000000000, 1.000000000000000000, 0.000000000000000000 ) ) ;
#30366=PLANE ( 'NONE',  #82258 ) ;
#30380=DIRECTION ( 'NONE',  ( 1.000000000000000000, 0.000000000000000000, 0.000000000000000000 ) ) ;
#30385=EDGE_CURVE ( 'NONE', #80198, #57275, #48641, .T. ) ;
#30387=EDGE_CURVE ( 'NONE', #1567, #84679, #60972, .T. ) ;
#30390=DIRECTION ( 'NONE',  ( -1.000000000000000000, -0.000000000000000000, 0.000000000000000000 ) ) ;
#30393=CARTESIAN_POINT ( 'NONE',  ( 160.5350683151633291, 250.0000000000000568, 15.22542485937381329 ) ) ;
#30394=DIRECTION ( 'NONE',  ( 0.000000000000000000, 0.000000000000000000, -1.000000000000000000 ) ) ;
#30403=ORIENTED_EDGE ( 'NONE', *, *, #48446, .F. ) ;
#30406=CIRCLE ( 'NONE', #54592, 6.286090667950827715 ) ;
#30420=CARTESIAN_POINT ( 'NONE',  ( 158.3977298502311157, 17.52828139914342032, 10.67961748034988823 ) ) ;
#30423=CARTESIAN_POINT ( 'NONE',  ( 160.5350683151633291, 275.5000000000000568, 12.00000000000000000 ) ) ;
#30437=ORIENTED_EDGE ( 'NONE', *, *, #73694, .F. ) ;
#30440=ORIENTED_EDGE ( 'NONE', *, *, #1762, .F. ) ;
#30450=ORIENTED_EDGE ( 'NONE', *, *, #56743, .T. ) ;
#30460=ORIENTED_EDGE ( 'NONE', *, *, #91412, .F. ) ;
#30468=CARTESIAN_POINT ( 'NONE',  ( 157.4642333713238429, 15.57755555264427372, 7.027845929950953696 ) ) ;
#30479=CIRCLE ( 'NONE', #39499, 25.00000000000000355 ) ;
#30483=DIRECTION ( 'NONE',  ( 0.000000000000000000, 0.000000000000000000, -1.000000000000000000 ) ) ;
#30486=AXIS2_PLACEMENT_3D ( 'NONE', #15960, #87891, #37257 ) ;
#30497=CARTESIAN_POINT ( 'NONE',  ( 154.3120505024572822, 19.86534941647866859, 13.70129228612852046 ) ) ;
#30500=EDGE_CURVE ( 'NONE', #90630, #60346, #84939, .T. ) ;
#30521=CARTESIAN_POINT ( 'NONE',  ( 209.2537080094121222, 37.08901624725314150, 12.07126757350762603 ) ) ;
#30538=DIRECTION ( 'NONE',  ( -0.000000000000000000, -1.000000000000000000, -0.000000000000000000 ) ) ;
#30539=AXIS2_PLACEMENT_3D ( 'NONE', #62399, #33492, #25917 ) ;
#30550=CIRCLE ( 'NONE', #42637, 4.999999999999986677 ) ;
#30570=ORIENTED_EDGE ( 'NONE', *, *, #17571, .T. ) ;
#30577=CARTESIAN_POINT ( 'NONE',  ( 197.5379522065467768, 249.5000000000000568, -11.97918851819042807 ) ) ;
#30578=( BOUNDED_CURVE ( )  B_SPLINE_CURVE ( 3, ( #65014, #36553, #14798, #87198 ),
 .UNSPECIFIED., .F., .F. ) 
 B_SPLINE_CURVE_WITH_KNOTS ( ( 4, 4 ),
 ( 1.570796326794895892, 2.617993877991479312 ),
 .UNSPECIFIED. ) 
 CURVE ( )  GEOMETRIC_REPRESENTATION_ITEM ( )  RATIONAL_B_SPLINE_CURVE ( ( 1.000000000000000000, 0.9106836025229615439, 0.9106836025229615439, 1.000000000000000000 ) ) 
 REPRESENTATION_ITEM ( '' )  );
#30584=CARTESIAN_POINT ( 'NONE',  ( 152.4536156746142410, 275.0000000000000568, -11.50000000000000355 ) ) ;
#30589=EDGE_LOOP ( 'NONE', ( #82390, #11465, #45235, #59837 ) ) ;
#30594=EDGE_CURVE ( 'NONE', #24375, #39851, #1533, .T. ) ;
#30608=CIRCLE ( 'NONE', #21561, 2.000000000000000888 ) ;
#30616=DIRECTION ( 'NONE',  ( -0.000000000000000000, 1.000000000000000000, -0.000000000000000000 ) ) ;
#30621=EDGE_CURVE ( 'NONE', #33982, #2466, #56225, .T. ) ;
#30626=DIRECTION ( 'NONE',  ( -0.9565177946839567014, 2.529868470129570114E-15, 0.2916739763039208899 ) ) ;
#30630=ADVANCED_FACE ( 'NONE', ( #35839, #36295 ), #86011, .F. ) ;
#30650=ORIENTED_EDGE ( 'NONE', *, *, #14576, .T. ) ;
#30651=LINE ( 'NONE', #72807, #57533 ) ;
#30674=DIRECTION ( 'NONE',  ( 0.000000000000000000, 0.000000000000000000, 1.000000000000000000 ) ) ;
#30675=AXIS2_PLACEMENT_3D ( 'NONE', #59838, #8679, #53650 ) ;
#30687=AXIS2_PLACEMENT_3D ( 'NONE', #8372, #36791, #823 ) ;
#30697=AXIS2_PLACEMENT_3D ( 'NONE', #60787, #53678, #50986 ) ;
#30698=ADVANCED_FACE ( 'NONE', ( #5573 ), #20236, .T. ) ;
#30700=FACE_OUTER_BOUND ( 'NONE', #71123, .T. ) ;
#30714=ORIENTED_EDGE ( 'NONE', *, *, #35942, .F. ) ;
#30715=VERTEX_POINT ( 'NONE', #34905 ) ;
#30716=CARTESIAN_POINT ( 'NONE',  ( 198.6639115758706282, 17.12212513345147258, -10.45170682515602323 ) ) ;
#30720=ADVANCED_FACE ( 'NONE', ( #65212 ), #49113, .F. ) ;
#30730=CARTESIAN_POINT ( 'NONE',  ( 196.8771864013320680, 214.6606447562234905, -12.54327527393323649 ) ) ;
#30742=EDGE_CURVE ( 'NONE', #63051, #14152, #50968, .T. ) ;
#30744=CARTESIAN_POINT ( 'NONE',  ( 183.0442525570908288, 300.2961574867697436, -7.500000000000000000 ) ) ;
#30746=CARTESIAN_POINT ( 'NONE',  ( 170.7304434856092143, 276.0000000000000568, -24.91818181818181088 ) ) ;
#30747=CIRCLE ( 'NONE', #48839, 2.000000000000001776 ) ;
#30750=CIRCLE ( 'NONE', #48842, 2.000000000000000000 ) ;
#30756=CIRCLE ( 'NONE', #70025, 4.999999999999976907 ) ;
#30759=CARTESIAN_POINT ( 'NONE',  ( 201.2104617360081704, 0.000000000000000000, 9.000000000000001776 ) ) ;
#30771=ORIENTED_EDGE ( 'NONE', *, *, #68018, .T. ) ;
#30772=CARTESIAN_POINT ( 'NONE',  ( 202.6531192844442728, 63.25403289341416269, -9.673168394505404777 ) ) ;
#30773=VECTOR ( 'NONE', #68109, 1000.000000000000000 ) ;
#30776=DIRECTION ( 'NONE',  ( 1.000000000000000000, -0.000000000000000000, 5.880589007913310608E-16 ) ) ;
#30786=ORIENTED_EDGE ( 'NONE', *, *, #59917, .F. ) ;
#30790=CARTESIAN_POINT ( 'NONE',  ( 198.3013281324776926, 65.29263651785086608, 9.735123833055002507 ) ) ;
#30793=DIRECTION ( 'NONE',  ( 0.000000000000000000, 0.000000000000000000, 1.000000000000000000 ) ) ;
#30810=EDGE_LOOP ( 'NONE', ( #87571, #9856, #38318, #70436 ) ) ;
#30811=ORIENTED_EDGE ( 'NONE', *, *, #35747, .T. ) ;
#30813=AXIS2_PLACEMENT_3D ( 'NONE', #49578, #85091, #42463 ) ;
#30819=CARTESIAN_POINT ( 'NONE',  ( 209.1374487190023501, 30.94653725228601715, 12.09245862095555601 ) ) ;
#30825=AXIS2_PLACEMENT_3D ( 'NONE', #37594, #8717, #59878 ) ;
#30832=CARTESIAN_POINT ( 'NONE',  ( 194.2870706607532441, 27.06158795357650604, 14.58823529798582896 ) ) ;
#30834=AXIS2_PLACEMENT_3D ( 'NONE', #75687, #10812, #92218 ) ;
#30851=AXIS2_PLACEMENT_3D ( 'NONE', #29737, #81298, #65747 ) ;
#30858=CARTESIAN_POINT ( 'NONE',  ( 194.5400481336216387, 25.95059276991969099, 14.25215709970754041 ) ) ;
#30864=DIRECTION ( 'NONE',  ( 1.000000000000000000, 0.000000000000000000, 0.000000000000000000 ) ) ;
#30866=FACE_OUTER_BOUND ( 'NONE', #29022, .T. ) ;
#30869=CARTESIAN_POINT ( 'NONE',  ( 198.5293976728803784, 41.98013133710430367, 10.72178272438543445 ) ) ;
#30878=EDGE_CURVE ( 'NONE', #46575, #25984, #92508, .T. ) ;
#30880=EDGE_LOOP ( 'NONE', ( #4119, #57344, #86774 ) ) ;
#30884=CARTESIAN_POINT ( 'NONE',  ( 195.4781563537916043, 27.48493576247232895, 15.00000000000000000 ) ) ;
#30896=AXIS2_PLACEMENT_3D ( 'NONE', #43436, #56263, #13186 ) ;
#30898=CIRCLE ( 'NONE', #83803, 0.5000000000000004441 ) ;
#30899=CARTESIAN_POINT ( 'NONE',  ( 156.4697130957886202, 16.02030068022430598, 10.01540472299883788 ) ) ;
#30902=CARTESIAN_POINT ( 'NONE',  ( 219.8344101925596021, 35.72494958537217968, 7.000000000000000000 ) ) ;
#30904=CIRCLE ( 'NONE', #83810, 0.5000000000000004441 ) ;
#30920=ORIENTED_EDGE ( 'NONE', *, *, #30385, .T. ) ;
#30936=EDGE_CURVE ( 'NONE', #69284, #47807, #1813, .T. ) ;
#30940=ADVANCED_FACE ( 'NONE', ( #81233, #23007 ), #51420, .T. ) ;
#30950=CARTESIAN_POINT ( 'NONE',  ( 159.4851178187817879, 15.28877977928774357, 9.000000000000001776 ) ) ;
#30953=ORIENTED_EDGE ( 'NONE', *, *, #16095, .T. ) ;
#30954=VERTEX_POINT ( 'NONE', #44318 ) ;
#30980=CIRCLE ( 'NONE', #19087, 25.00000000000000355 ) ;
#30982=DIRECTION ( 'NONE',  ( 1.000000000000000000, 0.000000000000000000, 0.000000000000000000 ) ) ;
#30986=CIRCLE ( 'NONE', #83880, 2.000000000000001776 ) ;
#31000=VERTEX_POINT ( 'NONE', #30584 ) ;
#31004=DIRECTION ( 'NONE',  ( 0.000000000000000000, 0.000000000000000000, 1.000000000000000000 ) ) ;
#31007=DIRECTION ( 'NONE',  ( 0.000000000000000000, 0.000000000000000000, 1.000000000000000000 ) ) ;
#31038=ORIENTED_EDGE ( 'NONE', *, *, #89992, .F. ) ;
#31045=CARTESIAN_POINT ( 'NONE',  ( 207.7761861081325776, 35.69891260691534285, 14.41714557868295010 ) ) ;
#31052=EDGE_CURVE ( 'NONE', #36421, #48026, #57731, .T. ) ;
#31054=CIRCLE ( 'NONE', #40070, 0.4999999999999983347 ) ;
#31059=VERTEX_POINT ( 'NONE', #8793 ) ;
#31060=CARTESIAN_POINT ( 'NONE',  ( 156.5440870305766055, 249.5000000000000568, 17.21343741151179429 ) ) ;
#31066=CARTESIAN_POINT ( 'NONE',  ( 197.4232166643840856, 67.42327970493053613, -10.33362320210538421 ) ) ;
#31067=DIRECTION ( 'NONE',  ( -1.000000000000000000, 0.000000000000000000, 0.000000000000000000 ) ) ;
#31072=ORIENTED_EDGE ( 'NONE', *, *, #42128, .T. ) ;
#31073=CARTESIAN_POINT ( 'NONE',  ( 196.7383257810085979, 24.47698789593438917, 11.00000000000000000 ) ) ;
#31092=DIRECTION ( 'NONE',  ( 0.000000000000000000, 0.000000000000000000, 1.000000000000000000 ) ) ;
#31097=DIRECTION ( 'NONE',  ( 0.000000000000000000, 0.8660254037842823882, 0.5000000000002706724 ) ) ;
#31102=CARTESIAN_POINT ( 'NONE',  ( 189.9243309297870610, 275.5000000000000568, 20.22542485937349355 ) ) ;
#31130=VERTEX_POINT ( 'NONE', #45230 ) ;
#31131=LINE ( 'NONE', #377, #15201 ) ;
#31148=EDGE_CURVE ( 'NONE', #26188, #50286, #72748, .T. ) ;
#31154=LINE ( 'NONE', #1326, #59420 ) ;
#31159=VERTEX_POINT ( 'NONE', #25238 ) ;
#31175=ADVANCED_FACE ( 'NONE', ( #74135 ), #6362, .T. ) ;
#31177=CARTESIAN_POINT ( 'NONE',  ( 152.6524812969444724, 129.6175404775655409, 12.50000000000000000 ) ) ;
#31178=DIRECTION ( 'NONE',  ( 0.9531768234071974488, -0.3024135303179478762, 6.994718006607575617E-16 ) ) ;
#31186=DIRECTION ( 'NONE',  ( 1.000000000000000000, -0.000000000000000000, -0.000000000000000000 ) ) ;
#31188=AXIS2_PLACEMENT_3D ( 'NONE', #53852, #60966, #4131 ) ;
#31191=ORIENTED_EDGE ( 'NONE', *, *, #18859, .T. ) ;
#31193=CARTESIAN_POINT ( 'NONE',  ( 197.3663942936547073, 19.61288093082362138, -11.77299963048799825 ) ) ;
#31231=DIRECTION ( 'NONE',  ( -0.000000000000000000, -1.000000000000000000, -0.000000000000000000 ) ) ;
#31241=ORIENTED_EDGE ( 'NONE', *, *, #89572, .T. ) ;
#31242=CARTESIAN_POINT ( 'NONE',  ( 186.6539576904058890, 293.9636489450775230, 0.000000000000000000 ) ) ;
#31245=PLANE ( 'NONE',  #14179 ) ;
#31259=EDGE_CURVE ( 'NONE', #40445, #42785, #14755, .T. ) ;
#31270=ORIENTED_EDGE ( 'NONE', *, *, #32042, .T. ) ;
#31275=EDGE_CURVE ( 'NONE', #3784, #73161, #87399, .T. ) ;
#31277=EDGE_CURVE ( 'NONE', #78077, #59807, #16883, .T. ) ;
#31280=ORIENTED_EDGE ( 'NONE', *, *, #10209, .T. ) ;
#31287=CARTESIAN_POINT ( 'NONE',  ( 200.8419735307467420, 26.78103457774644269, 8.999999999999998224 ) ) ;
#31298=ORIENTED_EDGE ( 'NONE', *, *, #61840, .T. ) ;
#31308=CARTESIAN_POINT ( 'NONE',  ( 209.4803090767392462, 35.69423656899339647, 15.12480380540109870 ) ) ;
#31320=CARTESIAN_POINT ( 'NONE',  ( 194.6773453981025455, 25.62504034132872377, 14.06423177434174399 ) ) ;
#31329=CARTESIAN_POINT ( 'NONE',  ( 193.9646936176702070, 21.00000000000000000, -15.00000000000000000 ) ) ;
#31332=FACE_OUTER_BOUND ( 'NONE', #55099, .T. ) ;
#31341=ADVANCED_FACE ( 'NONE', ( #44782 ), #15449, .F. ) ;
#31344=CYLINDRICAL_SURFACE ( 'NONE', #58876, 0.5000000000000004441 ) ;
#31347=CARTESIAN_POINT ( 'NONE',  ( 196.9925019505417083, 24.91416401846167261, 12.94510111180389167 ) ) ;
#31359=CARTESIAN_POINT ( 'NONE',  ( 159.4851178187871312, 14.99999999999999645, 10.00000000000000178 ) ) ;
#31389=ORIENTED_EDGE ( 'NONE', *, *, #63818, .T. ) ;
#31400=ORIENTED_EDGE ( 'NONE', *, *, #80190, .F. ) ;
#31409=CARTESIAN_POINT ( 'NONE',  ( 158.9078607026168868, 17.25638377771124965, 9.432942837125230184 ) ) ;
#31412=EDGE_CURVE ( 'NONE', #82273, #18551, #27504, .T. ) ;
#31414=EDGE_LOOP ( 'NONE', ( #28558, #36122, #87979, #22156 ) ) ;
#31415=ORIENTED_EDGE ( 'NONE', *, *, #79046, .T. ) ;
#31426=CARTESIAN_POINT ( 'NONE',  ( 193.8296338041434126, 214.9642006536927852, 17.09991073265190309 ) ) ;
#31431=CARTESIAN_POINT ( 'NONE',  ( 219.8344101925596021, 3.000000000000000000, -9.000000000000001776 ) ) ;
#31437=CARTESIAN_POINT ( 'NONE',  ( 175.2296996224750103, 133.0000000000000000, -24.00000000000001066 ) ) ;
#31440=CARTESIAN_POINT ( 'NONE',  ( 154.1415209985679269, 20.37991841447901820, -11.45812909362559040 ) ) ;
#31442=CARTESIAN_POINT ( 'NONE',  ( 157.7437329832428077, 18.12362412296337411, -11.08836552221236538 ) ) ;
#31444=DIRECTION ( 'NONE',  ( 0.000000000000000000, 0.000000000000000000, -1.000000000000000000 ) ) ;
#31457=EDGE_LOOP ( 'NONE', ( #8232, #83885, #22381, #81907, #70861 ) ) ;
#31461=DIRECTION ( 'NONE',  ( 0.000000000000000000, 0.000000000000000000, 1.000000000000000000 ) ) ;
#31465=DIRECTION ( 'NONE',  ( 0.000000000000000000, 1.000000000000000000, 0.000000000000000000 ) ) ;
#31497=ORIENTED_EDGE ( 'NONE', *, *, #17827, .T. ) ;
#31513=ORIENTED_EDGE ( 'NONE', *, *, #63164, .F. ) ;
#31519=ORIENTED_EDGE ( 'NONE', *, *, #11007, .F. ) ;
#31528=EDGE_CURVE ( 'NONE', #28948, #8050, #76835, .T. ) ;
#31539=CARTESIAN_POINT ( 'NONE',  ( 189.9243309297870610, 275.5000000000000568, 25.22542485937350065 ) ) ;
#31544=DIRECTION ( 'NONE',  ( -0.000000000000000000, -1.000000000000000000, -0.000000000000000000 ) ) ;
#31554=DIRECTION ( 'NONE',  ( 1.000000000000000000, 0.000000000000000000, 0.000000000000000000 ) ) ;
#31567=ORIENTED_EDGE ( 'NONE', *, *, #7026, .F. ) ;
#31573=EDGE_CURVE ( 'NONE', #45087, #29052, #90993, .T. ) ;
#31575=DIRECTION ( 'NONE',  ( -1.000000000000000000, 0.000000000000000000, 0.000000000000000000 ) ) ;
#31588=ORIENTED_EDGE ( 'NONE', *, *, #52296, .T. ) ;
#31591=CARTESIAN_POINT ( 'NONE',  ( 209.1283748988095113, 29.46063112669806472, 13.48243931971135012 ) ) ;
#31600=ORIENTED_EDGE ( 'NONE', *, *, #5711, .F. ) ;
#31601=DIRECTION ( 'NONE',  ( -0.000000000000000000, -0.000000000000000000, -1.000000000000000000 ) ) ;
#31632=CIRCLE ( 'NONE', #43719, 25.00000000000001066 ) ;
#31633=CARTESIAN_POINT ( 'NONE',  ( 208.8914279315829106, 0.04196010845019378793, -7.500000000000011546 ) ) ;
#31641=CARTESIAN_POINT ( 'NONE',  ( 207.0609454132517726, 35.99714003645362226, 15.00000000000000000 ) ) ;
#31644=ORIENTED_EDGE ( 'NONE', *, *, #3875, .F. ) ;
#31646=CARTESIAN_POINT ( 'NONE',  ( 199.4949018615358511, 17.05867184936722936, -10.28330198088168501 ) ) ;
#31660=CARTESIAN_POINT ( 'NONE',  ( 199.0143093133015100, 17.19615242270663202, -9.000000000000001776 ) ) ;
#31672=ADVANCED_FACE ( 'NONE', ( #55534 ), #84383, .F. ) ;
#31673=DIRECTION ( 'NONE',  ( 0.000000000000000000, 1.000000000000000000, 0.000000000000000000 ) ) ;
#31682=ADVANCED_FACE ( 'NONE', ( #62166 ), #19532, .F. ) ;
#31692=EDGE_CURVE ( 'NONE', #2170, #46575, #24817, .T. ) ;
#31697=ORIENTED_EDGE ( 'NONE', *, *, #68134, .F. ) ;
#31698=CARTESIAN_POINT ( 'NONE',  ( 139.6539576904058606, 132.0000000000000568, 10.50000000000000000 ) ) ;
#31701=VECTOR ( 'NONE', #15840, 1000.000000000000000 ) ;
#31706=B_SPLINE_CURVE_WITH_KNOTS ( 'NONE', 3,
 ( #18457, #45933, #90861, #17544 ),
 .UNSPECIFIED., .F., .F.,
 ( 4, 4 ),
 ( 0.000000000000000000, 0.001074155171061463854 ),
 .UNSPECIFIED. ) ;
#31710=VERTEX_POINT ( 'NONE', #33742 ) ;
#31713=CARTESIAN_POINT ( 'NONE',  ( 199.0061125298537377, 249.5000000000000568, -7.725424859374024678 ) ) ;
#31719=CYLINDRICAL_SURFACE ( 'NONE', #76808, 2.000000000000000000 ) ;
#31720=CARTESIAN_POINT ( 'NONE',  ( 175.2296996224750103, 250.5000000000000568, 0.000000000000000000 ) ) ;
#31737=VERTEX_POINT ( 'NONE', #49353 ) ;
#31754=EDGE_LOOP ( 'NONE', ( #88527, #67687, #90731, #60590 ) ) ;
#31765=CARTESIAN_POINT ( 'NONE',  ( 208.9100279911569658, 35.82717761498059872, 14.27724168160876950 ) ) ;
#31774=EDGE_CURVE ( 'NONE', #6020, #36590, #11962, .T. ) ;
#31783=DIRECTION ( 'NONE',  ( 0.000000000000000000, 0.000000000000000000, 1.000000000000000000 ) ) ;
#31785=LINE ( 'NONE', #9997, #61913 ) ;
#31788=CARTESIAN_POINT ( 'NONE',  ( 200.2324206114115555, 214.8829713991971744, -2.809954999877010806 ) ) ;
#31803=EDGE_CURVE ( 'NONE', #19733, #1988, #65674, .T. ) ;
#31815=CARTESIAN_POINT ( 'NONE',  ( 156.4851178187871312, 14.99999999999999467, 7.000000000000000888 ) ) ;
#31817=AXIS2_PLACEMENT_3D ( 'NONE', #57230, #70016, #34035 ) ;
#31835=EDGE_LOOP ( 'NONE', ( #65337, #16237, #35843, #37883 ) ) ;
#31838=ORIENTED_EDGE ( 'NONE', *, *, #11779, .T. ) ;
#31848=EDGE_LOOP ( 'NONE', ( #2915, #46604, #83770, #35704 ) ) ;
#31866=ORIENTED_EDGE ( 'NONE', *, *, #89197, .T. ) ;
#31867=CARTESIAN_POINT ( 'NONE',  ( 208.6208076322478746, 32.98517505407394168, 14.49999999999999822 ) ) ;
#31888=CARTESIAN_POINT ( 'NONE',  ( 214.2238915819278589, 32.98517505407394168, 10.00000000000000000 ) ) ;
#31896=CIRCLE ( 'NONE', #4718, 3.000000000000002665 ) ;
#31898=DIRECTION ( 'NONE',  ( -1.000000000000000000, 0.000000000000000000, -0.000000000000000000 ) ) ;
#31900=CARTESIAN_POINT ( 'NONE',  ( 199.1087447750284980, 64.61450673763175701, 10.46317447812566392 ) ) ;
#31902=DIRECTION ( 'NONE',  ( -0.2156506209390900430, 0.000000000000000000, 0.9764705882352960886 ) ) ;
#31927=EDGE_CURVE ( 'NONE', #17402, #90054, #33063, .T. ) ;
#31954=ORIENTED_EDGE ( 'NONE', *, *, #37042, .F. ) ;
#31964=AXIS2_PLACEMENT_3D ( 'NONE', #68516, #4120, #54295 ) ;
#31987=DIRECTION ( 'NONE',  ( 1.000000000000000000, 0.000000000000000000, 0.000000000000000000 ) ) ;
#32000=CARTESIAN_POINT ( 'NONE',  ( 197.6897354370363473, 68.42890619940936858, 10.08371065145146872 ) ) ;
#32009=CARTESIAN_POINT ( 'NONE',  ( 201.6359441630863500, 62.93935058108146308, 6.999999999999996447 ) ) ;
#32014=CARTESIAN_POINT ( 'NONE',  ( 199.9311642430739653, 275.7557892102190067, -9.103929867429339851 ) ) ;
#32022=AXIS2_PLACEMENT_3D ( 'NONE', #85814, #92929, #64565 ) ;
#32027=CARTESIAN_POINT ( 'NONE',  ( 202.8019728163925492, 61.40723988820079171, -7.000000000000000888 ) ) ;
#32032=AXIS2_PLACEMENT_3D ( 'NONE', #35874, #58133, #6065 ) ;
#32042=EDGE_CURVE ( 'NONE', #35022, #60748, #55993, .T. ) ;
#32048=CARTESIAN_POINT ( 'NONE',  ( 202.9228084772383340, 300.2547313093774619, -4.941765029749829452 ) ) ;
#32059=CARTESIAN_POINT ( 'NONE',  ( 186.2362647323748490, 249.5000000000000568, 22.80382896336987031 ) ) ;
#32068=DIRECTION ( 'NONE',  ( -0.2156506209390900430, 0.000000000000000000, -0.9764705882352960886 ) ) ;
#32069=DIRECTION ( 'NONE',  ( 2.220446049250312686E-15, 0.000000000000000000, 1.000000000000000000 ) ) ;
#32073=ORIENTED_EDGE ( 'NONE', *, *, #85946, .F. ) ;
#32082=ORIENTED_EDGE ( 'NONE', *, *, #19750, .T. ) ;
#32090=CARTESIAN_POINT ( 'NONE',  ( 153.7504314680575987, 128.6410103095127226, 12.94315874461255689 ) ) ;
#32092=CARTESIAN_POINT ( 'NONE',  ( 195.2616234104794728, 71.31492948064700954, 13.29451844366211866 ) ) ;
#32093=CIRCLE ( 'NONE', #88034, 26.99999999999999289 ) ;
#32101=( GEOMETRIC_REPRESENTATION_CONTEXT ( 3 ) GLOBAL_UNCERTAINTY_ASSIGNED_CONTEXT ( ( #36837 ) ) GLOBAL_UNIT_ASSIGNED_CONTEXT ( ( #76509, #40946, #40478 ) ) REPRESENTATION_CONTEXT ( 'NONE', 'WORKASPACE' ) );
#32104=CYLINDRICAL_SURFACE ( 'NONE', #13936, 24.00000000000000355 ) ;
#32105=AXIS2_PLACEMENT_3D ( 'NONE', #76977, #54713, #91636 ) ;
#32108=ORIENTED_EDGE ( 'NONE', *, *, #12755, .F. ) ;
#32109=ORIENTED_EDGE ( 'NONE', *, *, #48515, .F. ) ;
#32125=CARTESIAN_POINT ( 'NONE',  ( 208.6208076322478746, 32.98517505407394168, 13.08022668053247095 ) ) ;
#32126=CARTESIAN_POINT ( 'NONE',  ( 155.4162060973593213, 20.04122387618562939, -15.25295451850657358 ) ) ;
#32138=DIRECTION ( 'NONE',  ( 0.000000000000000000, 0.000000000000000000, 1.000000000000000000 ) ) ;
#32160=ORIENTED_EDGE ( 'NONE', *, *, #22050, .T. ) ;
#32161=CARTESIAN_POINT ( 'NONE',  ( 190.2832783574276903, 8.542400036368780647, 9.000000000000001776 ) ) ;
#32162=CIRCLE ( 'NONE', #92641, 0.4999999999999983347 ) ;
#32173=EDGE_LOOP ( 'NONE', ( #86260, #48009, #63311, #11264 ) ) ;
#32182=DIRECTION ( 'NONE',  ( 0.000000000000000000, 0.000000000000000000, 1.000000000000000000 ) ) ;
#32190=AXIS2_PLACEMENT_3D ( 'NONE', #3861, #76762, #18064 ) ;
#32199=EDGE_LOOP ( 'NONE', ( #46513, #64743, #59187, #43388 ) ) ;
#32200=ORIENTED_EDGE ( 'NONE', *, *, #55616, .T. ) ;
#32201=DIRECTION ( 'NONE',  ( 0.000000000000000000, 0.000000000000000000, 1.000000000000000000 ) ) ;
#32206=CARTESIAN_POINT ( 'NONE',  ( 150.4957602436334412, 21.00000000000000000, -3.637614988394445081 ) ) ;
#32210=EDGE_CURVE ( 'NONE', #45666, #67402, #3664, .T. ) ;
#32218=ORIENTED_EDGE ( 'NONE', *, *, #58549, .F. ) ;
#32226=VECTOR ( 'NONE', #87542, 1000.000000000000000 ) ;
#32228=CARTESIAN_POINT ( 'NONE',  ( 208.1597743490453638, 35.80769208713102358, 15.05537761763264371 ) ) ;
#32238=AXIS2_PLACEMENT_3D ( 'NONE', #52924, #75645, #38717 ) ;
#32242=CARTESIAN_POINT ( 'NONE',  ( 196.0517256323039135, 25.50333437355849142, 11.93519303445567736 ) ) ;
#32245=CIRCLE ( 'NONE', #15627, 0.5000000000000000000 ) ;
#32250=CARTESIAN_POINT ( 'NONE',  ( 155.2961426000043730, 19.82592759221628498, 13.64628225442075937 ) ) ;
#32252=VECTOR ( 'NONE', #73854, 1000.000000000000000 ) ;
#32253=DIRECTION ( 'NONE',  ( -0.9531768234071978929, 0.3024135303179465439, 0.000000000000000000 ) ) ;
#32255=FACE_OUTER_BOUND ( 'NONE', #54741, .T. ) ;
#32256=FACE_OUTER_BOUND ( 'NONE', #46606, .T. ) ;
#32265=ORIENTED_EDGE ( 'NONE', *, *, #26684, .T. ) ;
#32266=CARTESIAN_POINT ( 'NONE',  ( 189.9243309297870610, 215.0000000000000568, 20.22542485937349355 ) ) ;
#32269=DIRECTION ( 'NONE',  ( 1.000000000000000000, 0.000000000000000000, 0.000000000000000000 ) ) ;
#32279=AXIS2_PLACEMENT_3D ( 'NONE', #74155, #31544, #58578 ) ;
#32281=CARTESIAN_POINT ( 'NONE',  ( 156.4869342561325993, 15.84738232520213863, 9.998183562658692125 ) ) ;
#32284=DIRECTION ( 'NONE',  ( 0.000000000000000000, 0.000000000000000000, -1.000000000000000000 ) ) ;
#32285=AXIS2_PLACEMENT_3D ( 'NONE', #22689, #51562, #80450 ) ;
#32295=VECTOR ( 'NONE', #13067, 1000.000000000000000 ) ;
#32301=ORIENTED_EDGE ( 'NONE', *, *, #46824, .F. ) ;
#32302=EDGE_CURVE ( 'NONE', #27101, #10184, #12926, .T. ) ;
#32304=ORIENTED_EDGE ( 'NONE', *, *, #8766, .T. ) ;
#32306=CIRCLE ( 'NONE', #85236, 0.9999999999999977796 ) ;
#32311=ADVANCED_FACE ( 'NONE', ( #20487 ), #30366, .F. ) ;
#32312=CARTESIAN_POINT ( 'NONE',  ( 200.2296996224750103, 68.12454877777268791, 0.000000000000000000 ) ) ;
#32317=ORIENTED_EDGE ( 'NONE', *, *, #86489, .F. ) ;
#32320=TOROIDAL_SURFACE ( 'NONE', #20229, 24.00000000000002132, 2.046895004029262388 ) ;
#32330=ORIENTED_EDGE ( 'NONE', *, *, #49257, .F. ) ;
#32338=EDGE_LOOP ( 'NONE', ( #86764, #16134, #22665, #92379 ) ) ;
#32342=EDGE_CURVE ( 'NONE', #66900, #61882, #20903, .T. ) ;
#32345=ORIENTED_EDGE ( 'NONE', *, *, #26014, .T. ) ;
#32356=CARTESIAN_POINT ( 'NONE',  ( 196.0143093133015384, 19.33012701892218743, 12.49999999999999112 ) ) ;
#32361=DIRECTION ( 'NONE',  ( -0.000000000000000000, 1.000000000000000000, -0.000000000000000000 ) ) ;
#32366=CARTESIAN_POINT ( 'NONE',  ( 154.9842916688209868, 275.0000000000000568, -12.88888888888890705 ) ) ;
#32367=DIRECTION ( 'NONE',  ( 0.000000000000000000, 1.000000000000000000, 0.000000000000000000 ) ) ;
#32369=AXIS2_PLACEMENT_3D ( 'NONE', #61812, #11611, #75086 ) ;
#32373=AXIS2_PLACEMENT_3D ( 'NONE', #65834, #22692, #58702 ) ;
#32374=CARTESIAN_POINT ( 'NONE',  ( 208.5338978937603258, 38.36651302259750196, 14.22786471510243089 ) ) ;
#32379=FACE_OUTER_BOUND ( 'NONE', #13467, .T. ) ;
#32390=ORIENTED_EDGE ( 'NONE', *, *, #91063, .F. ) ;
#32394=DIRECTION ( 'NONE',  ( 0.000000000000000000, -1.000000000000000000, 0.000000000000000000 ) ) ;
#32396=ORIENTED_EDGE ( 'NONE', *, *, #16325, .T. ) ;
#32398=CARTESIAN_POINT ( 'NONE',  ( 189.9243309297870610, 276.0000000000000568, 20.22542485937349355 ) ) ;
#32402=AXIS2_PLACEMENT_3D ( 'NONE', #68978, #32980, #90702 ) ;
#32429=ORIENTED_EDGE ( 'NONE', *, *, #6382, .T. ) ;
#32450=EDGE_LOOP ( 'NONE', ( #76571, #82977 ) ) ;
#32451=TOROIDAL_SURFACE ( 'NONE', #43000, 1.000000000000000000, 0.5000000000000000000 ) ;
#32453=EDGE_CURVE ( 'NONE', #82273, #30954, #37456, .T. ) ;
#32454=ADVANCED_FACE ( 'NONE', ( #50757, #71618 ), #14326, .T. ) ;
#32459=CARTESIAN_POINT ( 'NONE',  ( 150.7067237504873845, 20.03350844490827853, -5.072059973232346586 ) ) ;
#32462=CIRCLE ( 'NONE', #64282, 4.999999999999990230 ) ;
#32466=FACE_OUTER_BOUND ( 'NONE', #69684, .T. ) ;
#32471=B_SPLINE_CURVE_WITH_KNOTS ( 'NONE', 3,
 ( #62777, #89728, #62282, #55183 ),
 .UNSPECIFIED., .F., .F.,
 ( 4, 4 ),
 ( 0.000000000000000000, 0.001030223387688887536 ),
 .UNSPECIFIED. ) ;
#32482=CARTESIAN_POINT ( 'NONE',  ( 193.9723528053802397, 215.0000000000000568, 17.29054515234648548 ) ) ;
#32489=CARTESIAN_POINT ( 'NONE',  ( 196.7625956450359297, 41.84090722167074006, 13.23774126259613659 ) ) ;
#32499=B_SPLINE_CURVE_WITH_KNOTS ( 'NONE', 3,
 ( #84166, #48176, #12208, #35859, #27357, #77548, #64776, #41539 ),
 .UNSPECIFIED., .F., .F.,
 ( 4, 2, 2, 4 ),
 ( -4.472612521061397354E-06, 0.0004667749420422217231, 0.0007023987193238632977, 0.0009380224966055048181 ),
 .UNSPECIFIED. ) ;
#32511=( BOUNDED_CURVE ( )  B_SPLINE_CURVE ( 3, ( #63904, #56312, #78554, #71456 ),
 .UNSPECIFIED., .F., .F. ) 
 B_SPLINE_CURVE_WITH_KNOTS ( ( 4, 4 ),
 ( 3.871320309816762339, 4.712388980384689674 ),
 .UNSPECIFIED. ) 
 CURVE ( )  GEOMETRIC_REPRESENTATION_ITEM ( )  RATIONAL_B_SPLINE_CURVE ( ( 1.000000000000000000, 0.9419139527835183046, 0.9419139527835183046, 1.000000000000000000 ) ) 
 REPRESENTATION_ITEM ( '' )  );
#32521=AXIS2_PLACEMENT_3D ( 'NONE', #52570, #22310, #44993 ) ;
#32523=EDGE_CURVE ( 'NONE', #48610, #85305, #50502, .T. ) ;
#32526=ORIENTED_EDGE ( 'NONE', *, *, #66323, .F. ) ;
#32529=DIRECTION ( 'NONE',  ( 1.000000000000000000, 0.000000000000000000, 0.000000000000000000 ) ) ;
#32542=VERTEX_POINT ( 'NONE', #36538 ) ;
#32543=LINE ( 'NONE', #60953, #83371 ) ;
#32553=CARTESIAN_POINT ( 'NONE',  ( 175.2296996224750103, 275.5000000000000568, 0.000000000000000000 ) ) ;
#32557=ORIENTED_EDGE ( 'NONE', *, *, #80129, .F. ) ;
#32566=ORIENTED_EDGE ( 'NONE', *, *, #41871, .F. ) ;
#32574=CARTESIAN_POINT ( 'NONE',  ( 151.0524635986548674, 20.99320456764978715, 6.527652849435607862 ) ) ;
#32583=DIRECTION ( 'NONE',  ( 0.000000000000000000, 0.000000000000000000, 1.000000000000000000 ) ) ;
#32586=ORIENTED_EDGE ( 'NONE', *, *, #11892, .T. ) ;
#32587=CARTESIAN_POINT ( 'NONE',  ( 198.0894686820290929, 18.12099305396683135, 11.05388702473232954 ) ) ;
#32604=VECTOR ( 'NONE', #93117, 1000.000000000000000 ) ;
#32614=FACE_OUTER_BOUND ( 'NONE', #31754, .T. ) ;
#32616=DIRECTION ( 'NONE',  ( 0.000000000000000000, 0.000000000000000000, 1.000000000000000000 ) ) ;
#32622=CARTESIAN_POINT ( 'NONE',  ( 195.4781563537916043, 250.0000000000000568, 15.50000000000000000 ) ) ;
#32634=EDGE_LOOP ( 'NONE', ( #39409, #27624, #92055, #56834 ) ) ;
#32635=DIRECTION ( 'NONE',  ( 1.000000000000000000, 0.000000000000000000, 0.000000000000000000 ) ) ;
#32641=EDGE_CURVE ( 'NONE', #52690, #82136, #68691, .T. ) ;
#32642=EDGE_CURVE ( 'NONE', #73985, #17168, #13729, .T. ) ;
#32658=DIRECTION ( 'NONE',  ( 0.000000000000000000, 1.000000000000000000, 0.000000000000000000 ) ) ;
#32659=CARTESIAN_POINT ( 'NONE',  ( 195.9246352305470680, 25.72798252258608898, 14.39643678788906378 ) ) ;
#32668=ORIENTED_EDGE ( 'NONE', *, *, #26328, .T. ) ;
#32694=ORIENTED_EDGE ( 'NONE', *, *, #75975, .F. ) ;
#32695=CARTESIAN_POINT ( 'NONE',  ( 207.4724402404594343, 29.73442829110639352, 14.90057469441957672 ) ) ;
#32703=CARTESIAN_POINT ( 'NONE',  ( 138.6539576904058606, 250.0000000000000568, 12.50000000000000000 ) ) ;
#32709=ADVANCED_FACE ( 'NONE', ( #60657 ), #26434, .T. ) ;
#32715=FACE_OUTER_BOUND ( 'NONE', #78909, .T. ) ;
#32717=DIRECTION ( 'NONE',  ( -0.000000000000000000, -0.000000000000000000, -1.000000000000000000 ) ) ;
#32724=DIRECTION ( 'NONE',  ( -1.000000000000000000, 0.000000000000000000, 0.000000000000000000 ) ) ;
#32741=DIRECTION ( 'NONE',  ( 0.000000000000000000, 0.000000000000000000, 1.000000000000000000 ) ) ;
#32754=DIRECTION ( 'NONE',  ( 1.000000000000000000, 0.000000000000000000, 0.000000000000000000 ) ) ;
#32775=CARTESIAN_POINT ( 'NONE',  ( 196.5860305738692944, 20.47868439449646161, -13.00974972892932691 ) ) ;
#32780=ORIENTED_EDGE ( 'NONE', *, *, #59618, .T. ) ;
#32787=CARTESIAN_POINT ( 'NONE',  ( 184.7149167944524493, 8.542400036368780647, -9.000000000000001776 ) ) ;
#32814=CARTESIAN_POINT ( 'NONE',  ( 209.5027106082920056, 29.50523358103493621, 14.69807322781335834 ) ) ;
#32820=DIRECTION ( 'NONE',  ( 0.000000000000000000, 0.000000000000000000, 1.000000000000000000 ) ) ;
#32825=B_SPLINE_CURVE_WITH_KNOTS ( 'NONE', 3,
 ( #77497, #12644, #77982, #21134, #41489, #28255, #70872, #42430, #48126, #78443 ),
 .UNSPECIFIED., .F., .F.,
 ( 4, 2, 2, 2, 4 ),
 ( -1.095445519328078919E-05, 0.001993413916517096894, 0.002494506009444676011, 0.002995598102372255128, 0.003997782288227412495 ),
 .UNSPECIFIED. ) ;
#32826=CARTESIAN_POINT ( 'NONE',  ( 196.0143093133015384, 73.40565171261609123, 11.99999999999998757 ) ) ;
#32830=LINE ( 'NONE', #90552, #13601 ) ;
#32832=ORIENTED_EDGE ( 'NONE', *, *, #27099, .F. ) ;
#32833=CARTESIAN_POINT ( 'NONE',  ( 156.4697130957825095, 16.02030068022343201, -10.01540472299836182 ) ) ;
#32835=CARTESIAN_POINT ( 'NONE',  ( 207.3685651567432728, 30.41993118425675036, 14.46441793359390005 ) ) ;
#32848=ORIENTED_EDGE ( 'NONE', *, *, #72944, .T. ) ;
#32855=CARTESIAN_POINT ( 'NONE',  ( 198.7796172868510496, 65.30644135522835825, 10.61564514751593791 ) ) ;
#32871=DIRECTION ( 'NONE',  ( 0.000000000000000000, 0.000000000000000000, 1.000000000000000000 ) ) ;
#32884=ORIENTED_EDGE ( 'NONE', *, *, #57901, .F. ) ;
#32904=ORIENTED_EDGE ( 'NONE', *, *, #49892, .T. ) ;
#32918=DIRECTION ( 'NONE',  ( 1.000000000000000000, 0.000000000000000000, 0.000000000000000000 ) ) ;
#32922=DIRECTION ( 'NONE',  ( 1.000000000000000000, 0.000000000000000000, 0.000000000000000000 ) ) ;
#32930=CARTESIAN_POINT ( 'NONE',  ( 187.8995604928813918, 43.86402690510830382, 10.50000000000000000 ) ) ;
#32940=CARTESIAN_POINT ( 'NONE',  ( 209.0350460744446934, 30.15816704241420609, 14.26380412667063524 ) ) ;
#32943=DIRECTION ( 'NONE',  ( -1.000000000000000000, -0.000000000000000000, -0.000000000000000000 ) ) ;
#32949=DIRECTION ( 'NONE',  ( 0.9441124463974853720, 0.2938448091926765815, -0.1493550021521704296 ) ) ;
#32951=ADVANCED_FACE ( 'NONE', ( #89973 ), #21796, .T. ) ;
#32973=ADVANCED_FACE ( 'NONE', ( #59738 ), #39765, .F. ) ;
#32975=VECTOR ( 'NONE', #34627, 1000.000000000000000 ) ;
#32980=DIRECTION ( 'NONE',  ( 0.000000000000000000, 1.000000000000000000, 0.000000000000000000 ) ) ;
#32991=ORIENTED_EDGE ( 'NONE', *, *, #9108, .T. ) ;
#33002=CARTESIAN_POINT ( 'NONE',  ( 153.8638694011456209, 19.41512922080416459, -11.71395201670714137 ) ) ;
#33022=DIRECTION ( 'NONE',  ( 0.000000000000000000, 0.000000000000000000, -1.000000000000000000 ) ) ;
#33023=CARTESIAN_POINT ( 'NONE',  ( 197.7129307445136135, 68.09401877029563366, 12.80442219776279522 ) ) ;
#33030=DIRECTION ( 'NONE',  ( -0.000000000000000000, -1.000000000000000000, -0.000000000000000000 ) ) ;
#33035=ORIENTED_EDGE ( 'NONE', *, *, #33481, .T. ) ;
#33036=CARTESIAN_POINT ( 'NONE',  ( 200.7304780712221088, 15.47998366481819232, 9.999999999999360512 ) ) ;
#33051=DIRECTION ( 'NONE',  ( 0.000000000000000000, 0.000000000000000000, 1.000000000000000000 ) ) ;
#33052=CARTESIAN_POINT ( 'NONE',  ( 175.2296996224750103, 250.0000000000000568, 0.000000000000000000 ) ) ;
#33054=( BOUNDED_SURFACE ( )  B_SPLINE_SURFACE ( 3, 2, ( 
 ( #31900, #54597, #47956 ),
 ( #90109, #75915, #91020 ),
 ( #17701, #46554, #83468 ),
 ( #55083, #24800, #69753 ) ),
 .UNSPECIFIED., .F., .F., .F. ) 
 B_SPLINE_SURFACE_WITH_KNOTS ( ( 4, 4 ),
 ( 3, 3 ),
 ( 4.278565243615663150, 4.712388980384689674 ),
 ( 0.000000000000000000, 1.000000000000000000 ),
 .UNSPECIFIED. ) 
 GEOMETRIC_REPRESENTATION_ITEM ( )  RATIONAL_B_SPLINE_SURFACE ( (
 ( 1.000000000000000000, 0.8168508380123946644, 1.000000000000000000),
 ( 1.000000000000000000, 0.7849082635113637796, 1.000000000000000000),
 ( 1.000000000000000000, 0.7478056585118687538, 1.000000000000000000),
 ( 1.000000000000000000, 0.7071067811865480168, 1.000000000000000000) ) ) 
 REPRESENTATION_ITEM ( '' )  SURFACE ( )  );
#33063=( BOUNDED_CURVE ( )  B_SPLINE_CURVE ( 3, ( #40346, #34219, #19078, #91954 ),
 .UNSPECIFIED., .F., .F. ) 
 B_SPLINE_CURVE_WITH_KNOTS ( ( 4, 4 ),
 ( 0.7297276562269670031, 1.570796326794896558 ),
 .UNSPECIFIED. ) 
 CURVE ( )  GEOMETRIC_REPRESENTATION_ITEM ( )  RATIONAL_B_SPLINE_CURVE ( ( 1.000000000000000000, 0.9419139527835179715, 0.9419139527835179715, 1.000000000000000000 ) ) 
 REPRESENTATION_ITEM ( '' )  );
#33068=DIRECTION ( 'NONE',  ( -1.000000000000000000, 0.000000000000000000, 0.000000000000000000 ) ) ;
#33077=CARTESIAN_POINT ( 'NONE',  ( 205.7381008070598227, 0.000000000000000000, -7.000000000000000888 ) ) ;
#33085=EDGE_LOOP ( 'NONE', ( #7167, #69563, #3504, #19299 ) ) ;
#33088=CARTESIAN_POINT ( 'NONE',  ( 207.2844387419798693, 0.02860196560701895249, -7.415405905516098350 ) ) ;
#33097=ADVANCED_FACE ( 'NONE', ( #45475 ), #33156, .T. ) ;
#33099=EDGE_LOOP ( 'NONE', ( #31072, #54676, #23762, #56402 ) ) ;
#33104=EDGE_CURVE ( 'NONE', #43740, #70513, #36113, .T. ) ;
#33110=AXIS2_PLACEMENT_3D ( 'NONE', #64091, #65479, #596 ) ;
#33112=CARTESIAN_POINT ( 'NONE',  ( 152.4536156746142410, 275.5000000000000568, -14.50000000000000000 ) ) ;
#33121=ORIENTED_EDGE ( 'NONE', *, *, #75497, .T. ) ;
#33132=CARTESIAN_POINT ( 'NONE',  ( 200.2349812190172713, 66.43136063442170780, 7.741079165001067963 ) ) ;
#33148=DIRECTION ( 'NONE',  ( 0.000000000000000000, 0.000000000000000000, -1.000000000000000000 ) ) ;
#33156=CYLINDRICAL_SURFACE ( 'NONE', #634, 1.499999999999999556 ) ;
#33170=AXIS2_PLACEMENT_3D ( 'NONE', #59760, #52159, #80572 ) ;
#33175=AXIS2_PLACEMENT_3D ( 'NONE', #82073, #89628, #90106 ) ;
#33182=CYLINDRICAL_SURFACE ( 'NONE', #65608, 5.000000000000000888 ) ;
#33184=DIRECTION ( 'NONE',  ( 1.000000000000000000, -0.000000000000000000, 0.000000000000000000 ) ) ;
#33185=DIRECTION ( 'NONE',  ( 0.000000000000000000, -1.000000000000000000, 0.000000000000000000 ) ) ;
#33195=VERTEX_POINT ( 'NONE', #12814 ) ;
#33199=CARTESIAN_POINT ( 'NONE',  ( 175.2296996224750103, 276.0000000000000568, 0.000000000000000000 ) ) ;
#33225=VERTEX_POINT ( 'NONE', #48757 ) ;
#33227=ORIENTED_EDGE ( 'NONE', *, *, #59326, .F. ) ;
#33234=CIRCLE ( 'NONE', #15141, 2.500000000000002220 ) ;
#33240=AXIS2_PLACEMENT_3D ( 'NONE', #84405, #64087, #34242 ) ;
#33257=ORIENTED_EDGE ( 'NONE', *, *, #58566, .F. ) ;
#33258=LINE ( 'NONE', #62155, #51812 ) ;
#33286=DIRECTION ( 'NONE',  ( 0.000000000000000000, 0.000000000000000000, 1.000000000000000000 ) ) ;
#33287=CARTESIAN_POINT ( 'NONE',  ( 209.6287663260175975, 29.00782453271232697, 15.00000000000000000 ) ) ;
#33290=FACE_OUTER_BOUND ( 'NONE', #13464, .T. ) ;
#33294=CARTESIAN_POINT ( 'NONE',  ( 152.4536156746142410, 250.5000000000000568, -11.99999999999999289 ) ) ;
#33297=CARTESIAN_POINT ( 'NONE',  ( 154.7156223832783724, 20.48904911123736028, -12.57712157663156560 ) ) ;
#33306=CIRCLE ( 'NONE', #36354, 1.000000000000000888 ) ;
#33309=AXIS2_PLACEMENT_3D ( 'NONE', #86635, #21802, #50676 ) ;
#33315=DIRECTION ( 'NONE',  ( 1.000000000000000000, 0.000000000000000000, 0.000000000000000000 ) ) ;
#33329=CARTESIAN_POINT ( 'NONE',  ( 151.4851178187871312, 15.00000000000000000, 0.000000000000000000 ) ) ;
#33343=ORIENTED_EDGE ( 'NONE', *, *, #50473, .F. ) ;
#33346=ORIENTED_EDGE ( 'NONE', *, *, #35766, .F. ) ;
#33369=EDGE_CURVE ( 'NONE', #63082, #78294, #35443, .T. ) ;
#33371=VECTOR ( 'NONE', #77841, 1000.000000000000000 ) ;
#33378=CARTESIAN_POINT ( 'NONE',  ( 153.1901962297480111, 19.73438857712018901, -11.80184082122067757 ) ) ;
#33391=CARTESIAN_POINT ( 'NONE',  ( 153.7618596668268367, 19.60625832729682827, -12.81530480009370443 ) ) ;
#33396=CARTESIAN_POINT ( 'NONE',  ( 196.1824782687554034, 72.66633770555792182, 11.70872282517771623 ) ) ;
#33401=CARTESIAN_POINT ( 'NONE',  ( 199.4819116658660221, 63.22432295887224285, -9.188210044104502927 ) ) ;
#33405=CARTESIAN_POINT ( 'NONE',  ( 175.2296996224750103, 246.0000000000001137, 0.000000000000000000 ) ) ;
#33418=DIRECTION ( 'NONE',  ( -0.000000000000000000, -0.000000000000000000, -1.000000000000000000 ) ) ;
#33436=ORIENTED_EDGE ( 'NONE', *, *, #72628, .F. ) ;
#33437=CARTESIAN_POINT ( 'NONE',  ( 199.4897031045222775, 67.51130003612513519, 8.507168327817714371 ) ) ;
#33439=CARTESIAN_POINT ( 'NONE',  ( 208.2200286604726500, 29.14932976030723211, 13.33523498126286455 ) ) ;
#33450=ORIENTED_EDGE ( 'NONE', *, *, #65327, .F. ) ;
#33451=EDGE_LOOP ( 'NONE', ( #31191, #25859, #3310, #74688 ) ) ;
#33460=CARTESIAN_POINT ( 'NONE',  ( 184.1778392089217107, 3.000000000000000888, 9.000000000000001776 ) ) ;
#33461=CARTESIAN_POINT ( 'NONE',  ( 153.2628468892384603, 20.37991841447901820, 11.93555113919330424 ) ) ;
#33465=VERTEX_POINT ( 'NONE', #84738 ) ;
#33474=VERTEX_POINT ( 'NONE', #5237 ) ;
#33479=DIRECTION ( 'NONE',  ( 0.9531768234071980039, -0.3024135303179465439, 1.282457197809570761E-15 ) ) ;
#33481=EDGE_CURVE ( 'NONE', #21372, #3443, #34109, .T. ) ;
#33482=CYLINDRICAL_SURFACE ( 'NONE', #5238, 5.103083949679981579 ) ;
#33490=CARTESIAN_POINT ( 'NONE',  ( 185.1905923765118587, 250.0000000000000568, 21.83530662808691147 ) ) ;
#33492=DIRECTION ( 'NONE',  ( 0.000000000000000000, 1.000000000000000000, 0.000000000000000000 ) ) ;
#33494=ORIENTED_EDGE ( 'NONE', *, *, #59139, .F. ) ;
#33495=DIRECTION ( 'NONE',  ( -2.265761274745217776E-15, 0.000000000000000000, 1.000000000000000000 ) ) ;
#33498=EDGE_CURVE ( 'NONE', #87978, #44024, #30904, .T. ) ;
#33505=VECTOR ( 'NONE', #76127, 1000.000000000000000 ) ;
#33511=CARTESIAN_POINT ( 'NONE',  ( 189.4188515237862589, 293.9636489450775798, 13.99999999999999112 ) ) ;
#33512=CARTESIAN_POINT ( 'NONE',  ( 195.4525831896995953, 39.48772993134988241, 14.00000000000000533 ) ) ;
#33525=LINE ( 'NONE', #62431, #41472 ) ;
#33527=CARTESIAN_POINT ( 'NONE',  ( 180.6209651459523968, 275.0000000000000568, -24.41176470588238701 ) ) ;
#33534=CARTESIAN_POINT ( 'NONE',  ( 159.4851178187871312, 3.000000000000000000, -10.00000000000000000 ) ) ;
#33537=CARTESIAN_POINT ( 'NONE',  ( 196.3508760566247418, 41.60265626164483876, 13.80739217974186595 ) ) ;
#33545=ORIENTED_EDGE ( 'NONE', *, *, #24191, .F. ) ;
#33546=DIRECTION ( 'NONE',  ( 0.000000000000000000, 0.000000000000000000, -1.000000000000000000 ) ) ;
#33558=ORIENTED_EDGE ( 'NONE', *, *, #28307, .F. ) ;
#33570=CIRCLE ( 'NONE', #16951, 1.000000000000006439 ) ;
#33572=AXIS2_PLACEMENT_3D ( 'NONE', #3361, #2900, #31783 ) ;
#33573=CARTESIAN_POINT ( 'NONE',  ( 195.4781563537916895, 27.48493576247232895, 15.00000000000008882 ) ) ;
#33581=AXIS2_PLACEMENT_3D ( 'NONE', #79211, #72115, #7231 ) ;
#33584=EDGE_LOOP ( 'NONE', ( #55456, #38731, #86592, #87155 ) ) ;
#33612=CARTESIAN_POINT ( 'NONE',  ( 169.2494399300530290, 8.542400036368780647, 9.974999999999996092 ) ) ;
#33617=EDGE_CURVE ( 'NONE', #1567, #35945, #38450, .T. ) ;
#33636=CARTESIAN_POINT ( 'NONE',  ( 201.2509219215139922, 65.09645894978945080, 0.000000000000000000 ) ) ;
#33638=DIRECTION ( 'NONE',  ( 4.095251346825558428E-15, -1.000000000000000000, 0.000000000000000000 ) ) ;
#33639=AXIS2_PLACEMENT_3D ( 'NONE', #75079, #88337, #53766 ) ;
#33648=DIRECTION ( 'NONE',  ( 0.000000000000000000, 0.000000000000000000, 1.000000000000000000 ) ) ;
#33649=AXIS2_PLACEMENT_3D ( 'NONE', #15448, #72747, #7868 ) ;
#33651=CARTESIAN_POINT ( 'NONE',  ( 197.4046495284674165, 214.9970011440366875, -12.46212327005319587 ) ) ;
#33653=CARTESIAN_POINT ( 'NONE',  ( 154.1415209985679269, 20.37991841447902175, 11.45812909362559040 ) ) ;
#33662=ORIENTED_EDGE ( 'NONE', *, *, #91947, .T. ) ;
#33666=CARTESIAN_POINT ( 'NONE',  ( 156.5191989162425727, 250.0000000000000568, 16.58062614384861178 ) ) ;
#33672=VECTOR ( 'NONE', #49851, 1000.000000000000000 ) ;
#33681=CARTESIAN_POINT ( 'NONE',  ( 185.4166944662902665, 214.7015631973135044, 22.87680765314684095 ) ) ;
#33695=VERTEX_POINT ( 'NONE', #72403 ) ;
#33697=ORIENTED_EDGE ( 'NONE', *, *, #34577, .F. ) ;
#33703=DIRECTION ( 'NONE',  ( 1.000000000000000000, 0.000000000000000000, 0.000000000000000000 ) ) ;
#33708=ORIENTED_EDGE ( 'NONE', *, *, #46281, .F. ) ;
#33722=ORIENTED_EDGE ( 'NONE', *, *, #79144, .F. ) ;
#33724=CIRCLE ( 'NONE', #54864, 4.500000000000003553 ) ;
#33730=ORIENTED_EDGE ( 'NONE', *, *, #23779, .F. ) ;
#33742=CARTESIAN_POINT ( 'NONE',  ( 199.0061125298537377, 275.5000000000000568, -12.72542485937401580 ) ) ;
#33744=AXIS2_PLACEMENT_3D ( 'NONE', #23625, #51553, #45368 ) ;
#33748=DIRECTION ( 'NONE',  ( -0.000000000000000000, 1.000000000000000000, -0.000000000000000000 ) ) ;
#33760=DIRECTION ( 'NONE',  ( -1.000000000000000000, 0.000000000000000000, 0.000000000000000000 ) ) ;
#33767=ORIENTED_EDGE ( 'NONE', *, *, #48884, .F. ) ;
#33768=CARTESIAN_POINT ( 'NONE',  ( 207.6573036349384438, 36.26995571305734956, 14.90818566952114921 ) ) ;
#33770=CARTESIAN_POINT ( 'NONE',  ( 207.0345761854011073, 29.47290414794718671, 13.79342392267523643 ) ) ;
#33780=CIRCLE ( 'NONE', #35267, 0.4999999999999977796 ) ;
#33789=ORIENTED_EDGE ( 'NONE', *, *, #53476, .T. ) ;
#33794=AXIS2_PLACEMENT_3D ( 'NONE', #70362, #21079, #36216 ) ;
#33804=CIRCLE ( 'NONE', #14157, 24.00000000000000355 ) ;
#33810=CIRCLE ( 'NONE', #45889, 4.999999999999985789 ) ;
#33815=EDGE_CURVE ( 'NONE', #33225, #89964, #62021, .T. ) ;
#33817=CARTESIAN_POINT ( 'NONE',  ( 158.3135449435333442, 1.828427124746190957, 9.000000000000000000 ) ) ;
#33819=EDGE_CURVE ( 'NONE', #19834, #64501, #51071, .T. ) ;
#33825=AXIS2_PLACEMENT_3D ( 'NONE', #85617, #87007, #43007 ) ;
#33827=VERTEX_POINT ( 'NONE', #79957 ) ;
#33830=ORIENTED_EDGE ( 'NONE', *, *, #68796, .F. ) ;
#33846=ORIENTED_EDGE ( 'NONE', *, *, #73031, .T. ) ;
#33856=ADVANCED_FACE ( 'NONE', ( #1812 ), #7521, .T. ) ;
#33875=CARTESIAN_POINT ( 'NONE',  ( 153.9133111279453203, 20.47222690886559704, 13.06183683676577267 ) ) ;
#33877=AXIS2_PLACEMENT_3D ( 'NONE', #69263, #4392, #85790 ) ;
#33883=AXIS2_PLACEMENT_3D ( 'NONE', #2482, #60247, #10027 ) ;
#33888=LINE ( 'NONE', #4073, #50281 ) ;
#33889=CARTESIAN_POINT ( 'NONE',  ( 202.9738562182569694, 293.9636489450776367, -54.00000000000000000 ) ) ;
#33894=LINE ( 'NONE', #18754, #24526 ) ;
#33903=CARTESIAN_POINT ( 'NONE',  ( 152.4536156746142410, 276.0000000000000568, 12.00000000000000000 ) ) ;
#33906=DIRECTION ( 'NONE',  ( -0.000000000000000000, -1.000000000000000000, -0.000000000000000000 ) ) ;
#33924=CARTESIAN_POINT ( 'NONE',  ( 204.4182217051425141, 300.0864416745848757, -5.149757974892338552 ) ) ;
#33936=ORIENTED_EDGE ( 'NONE', *, *, #8605, .T. ) ;
#33941=AXIS2_PLACEMENT_3D ( 'NONE', #41741, #34196, #70654 ) ;
#33948=CARTESIAN_POINT ( 'NONE',  ( 194.2870706637141325, 27.48493576247232184, 14.58823529411763431 ) ) ;
#33949=AXIS2_PLACEMENT_3D ( 'NONE', #15558, #59599, #88449 ) ;
#33950=DIRECTION ( 'NONE',  ( 2.312964634635742267E-15, 0.000000000000000000, 1.000000000000000000 ) ) ;
#33954=ORIENTED_EDGE ( 'NONE', *, *, #4023, .T. ) ;
#33963=ORIENTED_EDGE ( 'NONE', *, *, #8701, .F. ) ;
#33968=CARTESIAN_POINT ( 'NONE',  ( 198.8231951154315880, 63.33276796857077784, 10.00000000000000000 ) ) ;
#33978=EDGE_CURVE ( 'NONE', #44024, #61775, #87503, .T. ) ;
#33980=CARTESIAN_POINT ( 'NONE',  ( 205.7786681169002350, 32.98517505407394168, 14.49999999999999822 ) ) ;
#33982=VERTEX_POINT ( 'NONE', #8901 ) ;
#33983=CARTESIAN_POINT ( 'NONE',  ( 199.0883366025557848, 17.54655016013997582, 10.45170682515655436 ) ) ;
#33997=DIRECTION ( 'NONE',  ( 0.000000000000000000, 1.000000000000000000, 0.000000000000000000 ) ) ;
#33998=CARTESIAN_POINT ( 'NONE',  ( 195.4387718505159626, 39.61567108744358734, 13.99040197475940772 ) ) ;
#34009=ADVANCED_FACE ( 'NONE', ( #30700 ), #22651, .F. ) ;
#34010=AXIS2_PLACEMENT_3D ( 'NONE', #22766, #74354, #58773 ) ;
#34012=DIRECTION ( 'NONE',  ( -0.2456588035076310295, 0.9693563597868428694, 0.000000000000000000 ) ) ;
#34023=CIRCLE ( 'NONE', #76324, 24.00000000000000355 ) ;
#34025=CARTESIAN_POINT ( 'NONE',  ( 164.2231345125756263, 264.6571197653884155, -7.500000000000000000 ) ) ;
#34034=ORIENTED_EDGE ( 'NONE', *, *, #87889, .F. ) ;
#34035=DIRECTION ( 'NONE',  ( -5.551115123125781913E-15, 0.000000000000000000, 1.000000000000000000 ) ) ;
#34047=ORIENTED_EDGE ( 'NONE', *, *, #61560, .F. ) ;
#34052=EDGE_CURVE ( 'NONE', #78455, #93104, #45051, .T. ) ;
#34061=LINE ( 'NONE', #25995, #38838 ) ;
#34083=ORIENTED_EDGE ( 'NONE', *, *, #9771, .F. ) ;
#34084=CARTESIAN_POINT ( 'NONE',  ( 154.7659666677267865, 20.47222690886501439, -12.53936336329526391 ) ) ;
#34100=ORIENTED_EDGE ( 'NONE', *, *, #50606, .T. ) ;
#34101=CARTESIAN_POINT ( 'NONE',  ( 206.6195589736935005, 30.30844190587212594, 15.00000000000000000 ) ) ;
#34109=LINE ( 'NONE', #11844, #67212 ) ;
#34121=CARTESIAN_POINT ( 'NONE',  ( 156.4851178187871312, 6.488953147413177264E-16, 8.757359312880714342 ) ) ;
#34123=DIRECTION ( 'NONE',  ( 0.000000000000000000, -0.000000000000000000, -1.000000000000000000 ) ) ;
#34135=DIRECTION ( 'NONE',  ( -1.000000000000000000, -0.000000000000000000, 0.000000000000000000 ) ) ;
#34144=EDGE_CURVE ( 'NONE', #33982, #48324, #89669, .T. ) ;
#34146=ORIENTED_EDGE ( 'NONE', *, *, #16095, .F. ) ;
#34147=LINE ( 'NONE', #91881, #21152 ) ;
#34163=ADVANCED_FACE ( 'NONE', ( #69020 ), #83668, .T. ) ;
#34178=VERTEX_POINT ( 'NONE', #16950 ) ;
#34189=ORIENTED_EDGE ( 'NONE', *, *, #66440, .F. ) ;
#34196=DIRECTION ( 'NONE',  ( 0.000000000000000000, 1.000000000000000000, 0.000000000000000000 ) ) ;
#34201=VERTEX_POINT ( 'NONE', #75187 ) ;
#34209=CARTESIAN_POINT ( 'NONE',  ( 160.5350683151633291, 250.5000000000000568, 20.22542485937379908 ) ) ;
#34219=CARTESIAN_POINT ( 'NONE',  ( 198.3547199411611928, 26.15070318860490772, 11.03083405179678067 ) ) ;
#34225=CARTESIAN_POINT ( 'NONE',  ( 209.1556935201577119, 29.41729090122338164, 14.69807323163421664 ) ) ;
#34233=EDGE_CURVE ( 'NONE', #87290, #1585, #15739, .T. ) ;
#34236=DIRECTION ( 'NONE',  ( 0.000000000000000000, 0.000000000000000000, -1.000000000000000000 ) ) ;
#34237=CARTESIAN_POINT ( 'NONE',  ( 196.7071296363290855, 19.50333209967907422, 12.79999999999999716 ) ) ;
#34242=DIRECTION ( 'NONE',  ( -0.7957555401921969640, -0.6056179655966498210, 0.000000000000000000 ) ) ;
#34244=DIRECTION ( 'NONE',  ( 0.000000000000000000, 1.000000000000000000, 0.000000000000000000 ) ) ;
#34246=DIRECTION ( 'NONE',  ( -0.8009040723493942027, 0.5987926743825080500, 0.000000000000000000 ) ) ;
#34249=CARTESIAN_POINT ( 'NONE',  ( 158.3977298502259146, 18.03393767897227207, -9.815540976419979913 ) ) ;
#34259=ORIENTED_EDGE ( 'NONE', *, *, #59920, .T. ) ;
#34262=CARTESIAN_POINT ( 'NONE',  ( 206.3138962770341323, 36.06169532515022524, 14.00000000000000178 ) ) ;
#34264=VERTEX_POINT ( 'NONE', #46283 ) ;
#34266=PLANE ( 'NONE',  #83578 ) ;
#34294=EDGE_CURVE ( 'NONE', #50747, #34264, #59867, .T. ) ;
#34296=VERTEX_POINT ( 'NONE', #88900 ) ;
#34299=ORIENTED_EDGE ( 'NONE', *, *, #36505, .T. ) ;
#34302=EDGE_CURVE ( 'NONE', #12419, #11243, #68549, .T. ) ;
#34317=ORIENTED_EDGE ( 'NONE', *, *, #4507, .T. ) ;
#34323=ORIENTED_EDGE ( 'NONE', *, *, #14640, .F. ) ;
#34327=PRODUCT_DEFINITION_CONTEXT ( 'detailed design', #80138, 'design' ) ;
#34328=B_SPLINE_CURVE_WITH_KNOTS ( 'NONE', 3,
 ( #31329, #53081, #74886, #24683, #82441, #27268, #40498, #76990 ),
 .UNSPECIFIED., .F., .F.,
 ( 4, 2, 2, 4 ),
 ( 0.000000000000000000, 0.001862880473700167768, 0.002794320710550249158, 0.003725760947400331199 ),
 .UNSPECIFIED. ) ;
#34345=CARTESIAN_POINT ( 'NONE',  ( 153.9133111279456045, 20.47222690886501795, -13.06183683676589702 ) ) ;
#34356=CARTESIAN_POINT ( 'NONE',  ( 208.7492649171146013, 30.13137537953640077, 14.27679763129792789 ) ) ;
#34359=CARTESIAN_POINT ( 'NONE',  ( 169.2744399300530347, 8.542400036368780647, 9.000000000000001776 ) ) ;
#34360=DIRECTION ( 'NONE',  ( 0.000000000000000000, -1.000000000000000000, 0.000000000000000000 ) ) ;
#34373=LINE ( 'NONE', #92111, #75290 ) ;
#34376=DIRECTION ( 'NONE',  ( 0.5729786897769825194, 5.686911123206608097E-15, 0.8195702660915978877 ) ) ;
#34393=CARTESIAN_POINT ( 'NONE',  ( 157.2348298300756539, 18.48484813927058923, 11.40642999294609083 ) ) ;
#34403=ORIENTED_EDGE ( 'NONE', *, *, #8766, .F. ) ;
#34414=CARTESIAN_POINT ( 'NONE',  ( 157.4970531492008661, 276.0000000000000568, 16.90571646082702983 ) ) ;
#34415=DIRECTION ( 'NONE',  ( -0.8526555397811730330, 0.000000000000000000, -0.5224734734706408812 ) ) ;
#34419=ORIENTED_EDGE ( 'NONE', *, *, #43977, .F. ) ;
#34429=ORIENTED_EDGE ( 'NONE', *, *, #53698, .T. ) ;
#34435=CARTESIAN_POINT ( 'NONE',  ( 157.4851178187871312, 15.00000000000000000, 10.00000000000000000 ) ) ;
#34436=CYLINDRICAL_SURFACE ( 'NONE', #35525, 4.999999999999990230 ) ;
#34437=CARTESIAN_POINT ( 'NONE',  ( 196.0143093133015384, 20.19615242270663913, 11.99999999999998757 ) ) ;
#34443=DIRECTION ( 'NONE',  ( -0.000000000000000000, -0.000000000000000000, -1.000000000000000000 ) ) ;
#34444=CARTESIAN_POINT ( 'NONE',  ( 175.2296996224750103, 247.0000000000001137, 0.000000000000000000 ) ) ;
#34446=ORIENTED_EDGE ( 'NONE', *, *, #61091, .T. ) ;
#34447=VERTEX_POINT ( 'NONE', #46743 ) ;
#34448=LINE ( 'NONE', #49117, #20205 ) ;
#34457=EDGE_CURVE ( 'NONE', #90280, #76413, #91148, .T. ) ;
#34463=FACE_OUTER_BOUND ( 'NONE', #30119, .T. ) ;
#34464=EDGE_CURVE ( 'NONE', #40097, #557, #36767, .T. ) ;
#34465=EDGE_CURVE ( 'NONE', #1176, #44442, #60522, .T. ) ;
#34466=CARTESIAN_POINT ( 'NONE',  ( 160.5350683151633291, 215.0000000000000568, 25.22542485937379197 ) ) ;
#34479=CYLINDRICAL_SURFACE ( 'NONE', #16894, 4.000000000000003553 ) ;
#34481=B_SPLINE_CURVE_WITH_KNOTS ( 'NONE', 3,
 ( #64916, #79562, #71058, #28436, #35057, #28897, #14245, #5723, #63977, #34598 ),
 .UNSPECIFIED., .F., .F.,
 ( 4, 2, 2, 2, 4 ),
 ( -1.095445519331009314E-05, 0.001993413916517070006, 0.002494506009444649557, 0.002995598102372229541, 0.003997782288227388209 ),
 .UNSPECIFIED. ) ;
#34491=CARTESIAN_POINT ( 'NONE',  ( 156.4851178187871312, 0.000000000000000000, -7.000000000000000888 ) ) ;
#34494=CARTESIAN_POINT ( 'NONE',  ( 196.7540967208871052, 41.83829464925010910, 13.24991213668545775 ) ) ;
#34503=CARTESIAN_POINT ( 'NONE',  ( 175.2296996224750103, 275.5000000000000568, 0.000000000000000000 ) ) ;
#34505=CARTESIAN_POINT ( 'NONE',  ( 201.2104617360081704, 15.00000000000000000, 10.00000000000000000 ) ) ;
#34515=ORIENTED_EDGE ( 'NONE', *, *, #24438, .T. ) ;
#34516=CARTESIAN_POINT ( 'NONE',  ( 194.7373591563044215, 39.36132622696001704, 13.99999999999999822 ) ) ;
#34519=DIRECTION ( 'NONE',  ( -0.000000000000000000, -1.000000000000000000, -0.000000000000000000 ) ) ;
#34521=ORIENTED_EDGE ( 'NONE', *, *, #74260, .F. ) ;
#34527=CYLINDRICAL_SURFACE ( 'NONE', #74466, 5.568361562975243650 ) ;
#34545=AXIS2_PLACEMENT_3D ( 'NONE', #88363, #23513, #31092 ) ;
#34560=ORIENTED_EDGE ( 'NONE', *, *, #34465, .F. ) ;
#34562=CARTESIAN_POINT ( 'NONE',  ( 201.2509219215139922, 65.09645894978946501, 0.000000000000000000 ) ) ;
#34566=EDGE_CURVE ( 'NONE', #14772, #27101, #45760, .T. ) ;
#34571=CARTESIAN_POINT ( 'NONE',  ( 201.6359441630863500, 62.93935058108146308, -6.999999999999996447 ) ) ;
#34577=EDGE_CURVE ( 'NONE', #23459, #30328, #20149, .T. ) ;
#34578=DIRECTION ( 'NONE',  ( -0.9510565162951499785, 0.000000000000000000, 0.3090169943749582204 ) ) ;
#34585=EDGE_CURVE ( 'NONE', #83027, #65034, #9733, .T. ) ;
#34598=CARTESIAN_POINT ( 'NONE',  ( 152.4536156746142410, 130.6065089285656313, 11.50000000000000000 ) ) ;
#34609=AXIS2_PLACEMENT_3D ( 'NONE', #20967, #14351, #13414 ) ;
#34613=CARTESIAN_POINT ( 'NONE',  ( 209.9972545312790544, 27.55378999303205845, 10.50000000000000000 ) ) ;
#34616=ADVANCED_FACE ( 'NONE', ( #76587 ), #33482, .T. ) ;
#34626=LINE ( 'NONE', #27525, #8198 ) ;
#34627=DIRECTION ( 'NONE',  ( 0.000000000000000000, 0.000000000000000000, 1.000000000000000000 ) ) ;
#34635=EDGE_CURVE ( 'NONE', #1470, #32542, #83001, .T. ) ;
#34640=EDGE_LOOP ( 'NONE', ( #78207, #42943, #71372, #20870 ) ) ;
#34642=ORIENTED_EDGE ( 'NONE', *, *, #36169, .T. ) ;
#34656=DIRECTION ( 'NONE',  ( -1.000000000000000000, 0.000000000000000000, 0.000000000000000000 ) ) ;
#34669=ORIENTED_EDGE ( 'NONE', *, *, #1954, .F. ) ;
#34670=CARTESIAN_POINT ( 'NONE',  ( 201.2104617360081704, 0.000000000000000000, -9.000000000000001776 ) ) ;
#34675=AXIS2_PLACEMENT_3D ( 'NONE', #6430, #35305, #29949 ) ;
#34681=DIRECTION ( 'NONE',  ( 0.000000000000000000, 0.000000000000000000, 1.000000000000000000 ) ) ;
#34695=EDGE_CURVE ( 'NONE', #75996, #59807, #62473, .T. ) ;
#34698=LINE ( 'NONE', #938, #32226 ) ;
#34702=EDGE_CURVE ( 'NONE', #25984, #40097, #29208, .T. ) ;
#34705=CARTESIAN_POINT ( 'NONE',  ( 200.5559520117673458, 215.0000000000000568, -2.971689740512053035 ) ) ;
#34708=CARTESIAN_POINT ( 'NONE',  ( 159.4851178187871312, 15.00000000000000000, -9.000000000000001776 ) ) ;
#34711=CARTESIAN_POINT ( 'NONE',  ( 159.2635086430407796, 16.43186977800939275, -9.166206881811431728 ) ) ;
#34740=AXIS2_PLACEMENT_3D ( 'NONE', #18519, #26569, #19003 ) ;
#34741=CARTESIAN_POINT ( 'NONE',  ( 154.2407498497630058, 20.33092290645582523, -11.64075539514040081 ) ) ;
#34744=CIRCLE ( 'NONE', #61979, 5.568361562975243650 ) ;
#34750=CARTESIAN_POINT ( 'NONE',  ( 222.8344101925596306, 3.000000000000000000, 10.00000000000000000 ) ) ;
#34758=ORIENTED_EDGE ( 'NONE', *, *, #2889, .T. ) ;
#34761=ORIENTED_EDGE ( 'NONE', *, *, #70954, .T. ) ;
#34764=EDGE_CURVE ( 'NONE', #27188, #31159, #813, .T. ) ;
#34785=ORIENTED_EDGE ( 'NONE', *, *, #32641, .F. ) ;
#34787=ORIENTED_EDGE ( 'NONE', *, *, #30500, .F. ) ;
#34788=EDGE_CURVE ( 'NONE', #70318, #48610, #17320, .T. ) ;
#34795=CARTESIAN_POINT ( 'NONE',  ( 175.2296996224750103, 133.0000000000000000, 23.00000000000000711 ) ) ;
#34800=DIRECTION ( 'NONE',  ( -1.110223024625155531E-13, 0.000000000000000000, 1.000000000000000000 ) ) ;
#34806=AXIS2_PLACEMENT_3D ( 'NONE', #90356, #67688, #83265 ) ;
#34809=CARTESIAN_POINT ( 'NONE',  ( 219.8344101925596021, 35.72494958537217968, -7.000000000000000000 ) ) ;
#34814=DIRECTION ( 'NONE',  ( 0.000000000000000000, 1.000000000000000000, 0.000000000000000000 ) ) ;
#34825=EDGE_CURVE ( 'NONE', #68312, #12543, #61268, .T. ) ;
#34828=B_SPLINE_CURVE_WITH_KNOTS ( 'NONE', 3,
 ( #5577, #85560, #14548, #29206, #93129, #28284 ),
 .UNSPECIFIED., .F., .F.,
 ( 4, 2, 4 ),
 ( 0.000000000000000000, 0.0009570384287224865559, 0.001914076857444973112 ),
 .UNSPECIFIED. ) ;
#34835=CARTESIAN_POINT ( 'NONE',  ( 202.9738562182569694, 293.9636489450776367, -44.00000000000000000 ) ) ;
#34865=ORIENTED_EDGE ( 'NONE', *, *, #91068, .F. ) ;
#34873=CIRCLE ( 'NONE', #59070, 7.999911143031724237 ) ;
#34879=AXIS2_PLACEMENT_3D ( 'NONE', #3502, #32394, #3034 ) ;
#34882=VERTEX_POINT ( 'NONE', #89164 ) ;
#34891=VERTEX_POINT ( 'NONE', #67431 ) ;
#34895=ORIENTED_EDGE ( 'NONE', *, *, #9842, .T. ) ;
#34896=FACE_OUTER_BOUND ( 'NONE', #36857, .T. ) ;
#34898=CARTESIAN_POINT ( 'NONE',  ( 201.2104617360081704, 15.00000000000000000, 9.000000000000001776 ) ) ;
#34905=CARTESIAN_POINT ( 'NONE',  ( 158.6539576904058606, 293.9636489450775230, 11.60392986742922439 ) ) ;
#34907=ORIENTED_EDGE ( 'NONE', *, *, #89600, .F. ) ;
#34908=ORIENTED_EDGE ( 'NONE', *, *, #48014, .T. ) ;
#34909=DIRECTION ( 'NONE',  ( -0.2456588035076310295, 0.9693563597868428694, 0.000000000000000000 ) ) ;
#34923=CARTESIAN_POINT ( 'NONE',  ( 196.7028786247088306, 293.4605932342957431, -7.988019280608678940 ) ) ;
#34937=ADVANCED_FACE ( 'NONE', ( #53192 ), #75910, .F. ) ;
#34938=CARTESIAN_POINT ( 'NONE',  ( 151.7006524173675928, 129.9758505473876369, -12.49999999999999822 ) ) ;
#34940=DIRECTION ( 'NONE',  ( 0.000000000000000000, 0.000000000000000000, 1.000000000000000000 ) ) ;
#34945=AXIS2_PLACEMENT_3D ( 'NONE', #78309, #55124, #19136 ) ;
#34950=AXIS2_PLACEMENT_3D ( 'NONE', #36961, #15647, #1903 ) ;
#34954=CARTESIAN_POINT ( 'NONE',  ( 195.6296657338482419, 40.56040261944446002, 14.76007111301385777 ) ) ;
#34963=CARTESIAN_POINT ( 'NONE',  ( 205.7381008070597943, 1.000000000000000000, -6.999999999999991118 ) ) ;
#34965=CARTESIAN_POINT ( 'NONE',  ( 209.0108701966262004, 28.85123441772958230, 12.07129462079433324 ) ) ;
#34980=ORIENTED_EDGE ( 'NONE', *, *, #22274, .T. ) ;
#34986=CARTESIAN_POINT ( 'NONE',  ( 175.2296996224750103, 250.5000000000000568, 0.000000000000000000 ) ) ;
#34990=EDGE_CURVE ( 'NONE', #12630, #55975, #83589, .T. ) ;
#35022=VERTEX_POINT ( 'NONE', #10567 ) ;
#35023=ORIENTED_EDGE ( 'NONE', *, *, #33104, .T. ) ;
#35024=DIRECTION ( 'NONE',  ( -0.000000000000000000, 1.000000000000000000, -0.000000000000000000 ) ) ;
#35057=CARTESIAN_POINT ( 'NONE',  ( 153.7700350902760533, 129.6490463903464274, 11.80126012119838208 ) ) ;
#35059=DIRECTION ( 'NONE',  ( -0.000000000000000000, -1.000000000000000000, -0.000000000000000000 ) ) ;
#35069=VECTOR ( 'NONE', #27820, 1000.000000000000000 ) ;
#35070=ORIENTED_EDGE ( 'NONE', *, *, #12828, .T. ) ;
#35071=DIRECTION ( 'NONE',  ( 0.000000000000000000, 1.000000000000000000, -0.000000000000000000 ) ) ;
#35072=AXIS2_PLACEMENT_3D ( 'NONE', #52610, #73936, #23747 ) ;
#35087=DIRECTION ( 'NONE',  ( 0.000000000000000000, 0.000000000000000000, -1.000000000000000000 ) ) ;
#35093=ADVANCED_FACE ( 'NONE', ( #39432 ), #55472, .T. ) ;
#35101=EDGE_LOOP ( 'NONE', ( #31038, #63576, #8335, #18175 ) ) ;
#35103=ORIENTED_EDGE ( 'NONE', *, *, #46621, .T. ) ;
#35121=ORIENTED_EDGE ( 'NONE', *, *, #44275, .F. ) ;
#35129=CARTESIAN_POINT ( 'NONE',  ( 196.0143093133015384, 24.42324672360810212, 11.99999999999998757 ) ) ;
#35141=AXIS2_PLACEMENT_3D ( 'NONE', #46792, #75694, #3738 ) ;
#35147=AXIS2_PLACEMENT_3D ( 'NONE', #15478, #44349, #73259 ) ;
#35149=CIRCLE ( 'NONE', #6375, 7.999911143031724237 ) ;
#35152=VERTEX_POINT ( 'NONE', #6289 ) ;
#35159=DIRECTION ( 'NONE',  ( -0.000000000000000000, -0.000000000000000000, 1.000000000000000000 ) ) ;
#35169=DIRECTION ( 'NONE',  ( 0.000000000000000000, 0.000000000000000000, 1.000000000000000000 ) ) ;
#35172=CARTESIAN_POINT ( 'NONE',  ( 175.2296996224750103, 21.00000000000000000, 15.00000000000000000 ) ) ;
#35182=ORIENTED_EDGE ( 'NONE', *, *, #999, .F. ) ;
#35187=ORIENTED_EDGE ( 'NONE', *, *, #7720, .T. ) ;
#35197=ORIENTED_EDGE ( 'NONE', *, *, #584, .F. ) ;
#35201=ADVANCED_FACE ( 'NONE', ( #18618 ), #12946, .F. ) ;
#35204=CARTESIAN_POINT ( 'NONE',  ( 204.6539576904058606, 293.9636489450775230, 0.000000000000000000 ) ) ;
#35207=CIRCLE ( 'NONE', #24582, 2.842139515347646750 ) ;
#35213=AXIS2_PLACEMENT_3D ( 'NONE', #68717, #33185, #10460 ) ;
#35218=AXIS2_PLACEMENT_3D ( 'NONE', #40261, #83356, #63038 ) ;
#35223=ORIENTED_EDGE ( 'NONE', *, *, #42272, .T. ) ;
#35226=ORIENTED_EDGE ( 'NONE', *, *, #21048, .F. ) ;
#35229=ADVANCED_FACE ( 'NONE', ( #4408 ), #70236, .T. ) ;
#35244=ORIENTED_EDGE ( 'NONE', *, *, #75328, .T. ) ;
#35248=AXIS2_PLACEMENT_3D ( 'NONE', #15745, #1992, #37496 ) ;
#35254=ORIENTED_EDGE ( 'NONE', *, *, #53031, .F. ) ;
#35261=PLANE ( 'NONE',  #68392 ) ;
#35266=CARTESIAN_POINT ( 'NONE',  ( 153.6539576904058038, 130.0000000000000568, 12.50000000000000000 ) ) ;
#35267=AXIS2_PLACEMENT_3D ( 'NONE', #73818, #24544, #46312 ) ;
#35276=CIRCLE ( 'NONE', #70097, 24.00000000000001421 ) ;
#35279=CARTESIAN_POINT ( 'NONE',  ( 156.4851178187871312, 0.000000000000000000, -7.000000000000000888 ) ) ;
#35283=CARTESIAN_POINT ( 'NONE',  ( 175.2296996224750103, 20.99999999999998934, 0.000000000000000000 ) ) ;
#35287=CARTESIAN_POINT ( 'NONE',  ( 199.1087447750284980, 64.61450673763175701, -10.46317447812566570 ) ) ;
#35297=AXIS2_PLACEMENT_3D ( 'NONE', #5120, #47716, #33051 ) ;
#35301=DIRECTION ( 'NONE',  ( 0.000000000000000000, 1.000000000000000000, 0.000000000000000000 ) ) ;
#35302=CARTESIAN_POINT ( 'NONE',  ( 209.2540529155442073, 37.08890681920322407, 12.07129462079485904 ) ) ;
#35305=DIRECTION ( 'NONE',  ( 0.000000000000000000, 0.000000000000000000, -1.000000000000000000 ) ) ;
#35309=AXIS2_PLACEMENT_3D ( 'NONE', #86652, #72927, #22270 ) ;
#35337=AXIS2_PLACEMENT_3D ( 'NONE', #27721, #34814, #42366 ) ;
#35348=CIRCLE ( 'NONE', #8093, 4.000000000000003553 ) ;
#35349=CARTESIAN_POINT ( 'NONE',  ( 184.7149167944524493, 8.542400036368780647, 10.00000000000000178 ) ) ;
#35358=AXIS2_PLACEMENT_3D ( 'NONE', #78710, #58345, #57415 ) ;
#35363=EDGE_LOOP ( 'NONE', ( #36389, #4379, #85043, #25890 ) ) ;
#35367=ORIENTED_EDGE ( 'NONE', *, *, #88464, .F. ) ;
#35369=VECTOR ( 'NONE', #38763, 1000.000000000000000 ) ;
#35371=EDGE_CURVE ( 'NONE', #37103, #78803, #73076, .T. ) ;
#35372=CARTESIAN_POINT ( 'NONE',  ( 150.6539576904058606, 293.9636489450775230, 0.000000000000000000 ) ) ;
#35379=CARTESIAN_POINT ( 'NONE',  ( 209.9972545312790544, 27.55378999303206200, 10.50000000000000000 ) ) ;
#35380=DIRECTION ( 'NONE',  ( 0.000000000000000000, 1.000000000000000000, 0.000000000000000000 ) ) ;
#35383=DIRECTION ( 'NONE',  ( 0.000000000000000000, 0.000000000000000000, -1.000000000000000000 ) ) ;
#35384=ORIENTED_EDGE ( 'NONE', *, *, #86333, .T. ) ;
#35385=FACE_OUTER_BOUND ( 'NONE', #71152, .T. ) ;
#35399=CARTESIAN_POINT ( 'NONE',  ( 200.3186454232214828, 275.5000000000000568, -3.421094783296264374 ) ) ;
#35400=CARTESIAN_POINT ( 'NONE',  ( 220.4471435719830197, 34.91984470236808136, -7.000000000000000888 ) ) ;
#35412=ADVANCED_FACE ( 'NONE', ( #26183 ), #19549, .F. ) ;
#35414=DIRECTION ( 'NONE',  ( 0.000000000000000000, -1.000000000000000000, -0.000000000000000000 ) ) ;
#35420=AXIS2_PLACEMENT_3D ( 'NONE', #4504, #90198, #32922 ) ;
#35430=CARTESIAN_POINT ( 'NONE',  ( 196.1222352346529192, 41.73615019500982726, 13.73113889404878485 ) ) ;
#35441=ORIENTED_EDGE ( 'NONE', *, *, #9521, .F. ) ;
#35442=CARTESIAN_POINT ( 'NONE',  ( 153.1901962297558839, 19.73438857711721894, 11.80184082123541423 ) ) ;
#35443=CIRCLE ( 'NONE', #88333, 3.842139515347647638 ) ;
#35445=CYLINDRICAL_SURFACE ( 'NONE', #45899, 1.000000000000000888 ) ;
#35455=ORIENTED_EDGE ( 'NONE', *, *, #63047, .F. ) ;
#35456=CARTESIAN_POINT ( 'NONE',  ( 195.7178114849801318, 40.54307234874452348, 13.60494157104296953 ) ) ;
#35467=CARTESIAN_POINT ( 'NONE',  ( 197.4476397837911463, 67.35440902555335185, -10.31415233767359929 ) ) ;
#35468=DIRECTION ( 'NONE',  ( -0.000000000000000000, -1.000000000000000000, -0.000000000000000000 ) ) ;
#35469=CARTESIAN_POINT ( 'NONE',  ( 189.4188515237862589, 293.9636489450775798, -9.103929867429222611 ) ) ;
#35478=ADVANCED_FACE ( 'NONE', ( #62672 ), #42248, .F. ) ;
#35479=ORIENTED_EDGE ( 'NONE', *, *, #48515, .T. ) ;
#35490=DIRECTION ( 'NONE',  ( 0.000000000000000000, 0.000000000000000000, 1.000000000000000000 ) ) ;
#35514=B_SPLINE_CURVE_WITH_KNOTS ( 'NONE', 3,
 ( #28092, #20516, #65021, #85366 ),
 .UNSPECIFIED., .F., .F.,
 ( 4, 4 ),
 ( 0.000000000000000000, 0.0006940106885258007230 ),
 .UNSPECIFIED. ) ;
#35522=CARTESIAN_POINT ( 'NONE',  ( 189.9243309297870610, 250.5000000000000568, 20.22542485937349355 ) ) ;
#35525=AXIS2_PLACEMENT_3D ( 'NONE', #26859, #41511, #56702 ) ;
#35533=FACE_OUTER_BOUND ( 'NONE', #86014, .T. ) ;
#35543=EDGE_CURVE ( 'NONE', #12291, #72750, #59494, .T. ) ;
#35545=CARTESIAN_POINT ( 'NONE',  ( 201.2104617360081704, 250.0000000000000568, 15.00000000000000000 ) ) ;
#35547=CARTESIAN_POINT ( 'NONE',  ( 197.3691676728705033, 70.32516635541138328, -11.79160090895328139 ) ) ;
#35558=ORIENTED_EDGE ( 'NONE', *, *, #24079, .T. ) ;
#35559=CARTESIAN_POINT ( 'NONE',  ( 183.0442525570908288, 264.6571197653884155, 7.500000000000000000 ) ) ;
#35561=DIRECTION ( 'NONE',  ( 0.000000000000000000, 1.000000000000000000, 0.000000000000000000 ) ) ;
#35587=VERTEX_POINT ( 'NONE', #71161 ) ;
#35594=VERTEX_POINT ( 'NONE', #5826 ) ;
#35611=ADVANCED_FACE ( 'NONE', ( #78266 ), #84487, .T. ) ;
#35615=CARTESIAN_POINT ( 'NONE',  ( 194.3388778885402814, 26.65530528383262521, 14.52131005158982369 ) ) ;
#35639=AXIS2_PLACEMENT_3D ( 'NONE', #45789, #51501, #30674 ) ;
#35642=CARTESIAN_POINT ( 'NONE',  ( 160.5350683151633291, 250.5000000000000568, 24.72542485937379197 ) ) ;
#35647=EDGE_CURVE ( 'NONE', #59134, #24951, #82175, .T. ) ;
#35652=DIRECTION ( 'NONE',  ( 0.000000000000000000, 0.000000000000000000, 1.000000000000000000 ) ) ;
#35655=CARTESIAN_POINT ( 'NONE',  ( 165.2424497756046549, 275.0000000000000568, 22.91843887563435445 ) ) ;
#35656=CARTESIAN_POINT ( 'NONE',  ( 157.4221907153413724, 15.99782226686453868, -9.062927103449267108 ) ) ;
#35669=CARTESIAN_POINT ( 'NONE',  ( 197.7335303680046650, 24.96166607582781083, 12.00000000000000178 ) ) ;
#35681=ORIENTED_EDGE ( 'NONE', *, *, #25637, .T. ) ;
#35687=CARTESIAN_POINT ( 'NONE',  ( 197.8563597697584839, 24.47698789593438917, 12.00000000000000178 ) ) ;
#35701=VERTEX_POINT ( 'NONE', #85808 ) ;
#35704=ORIENTED_EDGE ( 'NONE', *, *, #71157, .T. ) ;
#35722=ORIENTED_EDGE ( 'NONE', *, *, #43350, .F. ) ;
#35729=ORIENTED_EDGE ( 'NONE', *, *, #31528, .F. ) ;
#35731=ORIENTED_EDGE ( 'NONE', *, *, #8208, .T. ) ;
#35747=EDGE_CURVE ( 'NONE', #30213, #34891, #73146, .T. ) ;
#35752=DIRECTION ( 'NONE',  ( 0.000000000000000000, -1.000000000000000000, 0.000000000000000000 ) ) ;
#35756=LINE ( 'NONE', #84984, #36817 ) ;
#35759=CARTESIAN_POINT ( 'NONE',  ( 140.6539576904058606, 275.0000000000000568, 11.50000000000000000 ) ) ;
#35766=EDGE_CURVE ( 'NONE', #37280, #16726, #30578, .T. ) ;
#35774=LINE ( 'NONE', #64687, #81691 ) ;
#35817=ORIENTED_EDGE ( 'NONE', *, *, #59917, .T. ) ;
#35825=ORIENTED_EDGE ( 'NONE', *, *, #70691, .T. ) ;
#35830=CARTESIAN_POINT ( 'NONE',  ( 154.4601611254703641, 20.78894139178057543, -13.92477262272432448 ) ) ;
#35839=FACE_BOUND ( 'NONE', #59264, .T. ) ;
#35841=EDGE_LOOP ( 'NONE', ( #35070, #13567, #18117, #24878 ) ) ;
#35843=ORIENTED_EDGE ( 'NONE', *, *, #52765, .F. ) ;
#35848=EDGE_CURVE ( 'NONE', #46065, #79497, #39841, .T. ) ;
#35859=CARTESIAN_POINT ( 'NONE',  ( 193.4805262621761699, 275.8411434044543284, 16.89623125813409033 ) ) ;
#35860=CARTESIAN_POINT ( 'NONE',  ( 175.2296996224750103, 250.0000000000000568, 0.000000000000000000 ) ) ;
#35874=CARTESIAN_POINT ( 'NONE',  ( 160.5350683151633291, 215.0000000000000568, 20.22542485937379908 ) ) ;
#35883=CARTESIAN_POINT ( 'NONE',  ( 197.0195873853737965, 40.95756171125039202, 12.27312447568957232 ) ) ;
#35886=CARTESIAN_POINT ( 'NONE',  ( 207.5150402071092799, 1.051285333831500024, 7.457902384259533335 ) ) ;
#35889=CARTESIAN_POINT ( 'NONE',  ( 200.6103193995254230, 250.5000000000000568, -2.464576988612312114 ) ) ;
#35900=FACE_OUTER_BOUND ( 'NONE', #38229, .T. ) ;
#35911=ORIENTED_EDGE ( 'NONE', *, *, #45009, .F. ) ;
#35918=EDGE_LOOP ( 'NONE', ( #71927, #49914, #83083, #5909 ) ) ;
#35924=CARTESIAN_POINT ( 'NONE',  ( 199.0345205062965590, 66.35750757917867304, -8.036855303410847640 ) ) ;
#35942=EDGE_CURVE ( 'NONE', #5341, #90630, #8114, .T. ) ;
#35945=VERTEX_POINT ( 'NONE', #44578 ) ;
#35959=ORIENTED_EDGE ( 'NONE', *, *, #87554, .F. ) ;
#35960=VERTEX_POINT ( 'NONE', #93383 ) ;
#35961=CARTESIAN_POINT ( 'NONE',  ( 207.7755975652984830, 28.53818587417392294, 12.00000000000000000 ) ) ;
#35975=CARTESIAN_POINT ( 'NONE',  ( 197.1844320129423807, 70.43964897667966341, -15.08154681515735085 ) ) ;
#35976=CARTESIAN_POINT ( 'NONE',  ( 180.7287904564219332, 250.0000000000000568, -24.90000000000002345 ) ) ;
#35987=CARTESIAN_POINT ( 'NONE',  ( 187.8995604928813918, 43.86402690510830382, 15.00000000000000000 ) ) ;
#35999=EDGE_CURVE ( 'NONE', #1988, #52326, #63050, .T. ) ;
#36000=CARTESIAN_POINT ( 'NONE',  ( 198.9494509394918396, 68.47434140769267685, -9.196269295805851840 ) ) ;
#36012=EDGE_LOOP ( 'NONE', ( #86330, #63469, #6944 ) ) ;
#36013=DIRECTION ( 'NONE',  ( -0.3024135303179394940, -0.9531768234072001134, 0.000000000000000000 ) ) ;
#36015=CARTESIAN_POINT ( 'NONE',  ( 156.4851178187871312, 1.000000000000000000, 7.000000000000000000 ) ) ;
#36029=DIRECTION ( 'NONE',  ( 1.000000000000000000, 0.000000000000000000, 0.000000000000000000 ) ) ;
#36031=AXIS2_PLACEMENT_3D ( 'NONE', #44042, #28928, #15183 ) ;
#36056=CARTESIAN_POINT ( 'NONE',  ( 185.4166944662832179, 249.5000000000000568, 23.37680765314684095 ) ) ;
#36069=CARTESIAN_POINT ( 'NONE',  ( 195.0378959947337592, 25.05079320569620904, 13.55224814914091525 ) ) ;
#36102=( BOUNDED_SURFACE ( )  B_SPLINE_SURFACE ( 3, 2, ( 
 ( #2752, #83203, #3690 ),
 ( #89359, #25450, #11711 ),
 ( #53873, #10769, #4153 ),
 ( #46284, #75188, #90298 ),
 ( #33023, #24516, #40564 ),
 ( #18350, #32092, #53397 ) ),
 .UNSPECIFIED., .F., .F., .F. ) 
 B_SPLINE_SURFACE_WITH_KNOTS ( ( 4, 2, 4 ),
 ( 3, 3 ),
 ( 0.000000000000000000, 0.2633701841259441512, 0.5267403682518883024 ),
 ( 0.000000000000000000, 1.000000000000000000 ),
 .UNSPECIFIED. ) 
 GEOMETRIC_REPRESENTATION_ITEM ( )  RATIONAL_B_SPLINE_SURFACE ( (
 ( 1.000000000000000000, 0.9475641245298915827, 1.000000000000000000),
 ( 1.000000000000000000, 0.9475658968925606551, 1.000000000000000000),
 ( 1.000000000000000000, 0.9451322790880675173, 1.000000000000000000),
 ( 1.000000000000000000, 0.9354614375526318915, 1.000000000000000000),
 ( 1.000000000000000000, 0.9282241625909629645, 1.000000000000000000),
 ( 1.000000000000000000, 0.9186651033962672797, 1.000000000000000000) ) ) 
 REPRESENTATION_ITEM ( '' )  SURFACE ( )  );
#36103=CARTESIAN_POINT ( 'NONE',  ( 175.2296996224750103, 150.9142415853029036, 0.000000000000000000 ) ) ;
#36106=DIRECTION ( 'NONE',  ( -1.000000000000000000, 0.000000000000000000, 0.000000000000000000 ) ) ;
#36107=CARTESIAN_POINT ( 'NONE',  ( 159.4851178187871312, 14.99999999999999467, -9.000000000000001776 ) ) ;
#36113=( BOUNDED_CURVE ( )  B_SPLINE_CURVE ( 3, ( #41160, #34571, #26530, #6162 ),
 .UNSPECIFIED., .F., .F. ) 
 B_SPLINE_CURVE_WITH_KNOTS ( ( 4, 4 ),
 ( 1.570796326794895004, 2.004620063563922638 ),
 .UNSPECIFIED. ) 
 CURVE ( )  GEOMETRIC_REPRESENTATION_ITEM ( )  RATIONAL_B_SPLINE_CURVE ( ( 1.000000000000000000, 0.9843778111405747655, 0.9843778111405747655, 1.000000000000000000 ) ) 
 REPRESENTATION_ITEM ( '' )  );
#36117=EDGE_LOOP ( 'NONE', ( #61801, #48868, #37538, #71657 ) ) ;
#36122=ORIENTED_EDGE ( 'NONE', *, *, #12195, .T. ) ;
#36130=EDGE_LOOP ( 'NONE', ( #28487, #92464, #83435, #3421, #67289, #77404 ) ) ;
#36134=CARTESIAN_POINT ( 'NONE',  ( 202.1700622694972083, 300.2031883395015939, -5.006794249105121608 ) ) ;
#36151=ORIENTED_EDGE ( 'NONE', *, *, #81715, .F. ) ;
#36154=ORIENTED_EDGE ( 'NONE', *, *, #17632, .F. ) ;
#36169=EDGE_CURVE ( 'NONE', #25231, #69141, #33804, .T. ) ;
#36172=ADVANCED_FACE ( 'NONE', ( #15717 ), #44105, .F. ) ;
#36174=VERTEX_POINT ( 'NONE', #73010 ) ;
#36181=ORIENTED_EDGE ( 'NONE', *, *, #8683, .T. ) ;
#36184=EDGE_LOOP ( 'NONE', ( #41872, #21049, #75414, #88913 ) ) ;
#36193=CARTESIAN_POINT ( 'NONE',  ( 156.4851178187871312, 0.000000000000000000, 7.000000000000000000 ) ) ;
#36204=EDGE_CURVE ( 'NONE', #13726, #3915, #25777, .T. ) ;
#36205=CARTESIAN_POINT ( 'NONE',  ( 155.7140808774799723, 21.00000000000000000, 15.62500000000000000 ) ) ;
#36212=DIRECTION ( 'NONE',  ( -0.000000000000000000, -0.000000000000000000, 1.000000000000000000 ) ) ;
#36216=DIRECTION ( 'NONE',  ( -0.8660254037844404840, 0.000000000000000000, -0.4999999999999968359 ) ) ;
#36286=CARTESIAN_POINT ( 'NONE',  ( 196.6762265213135947, 24.45209518732023568, 12.85352576531901292 ) ) ;
#36290=CIRCLE ( 'NONE', #18177, 7.500000000000013323 ) ;
#36294=CARTESIAN_POINT ( 'NONE',  ( 208.4784300167292201, 27.68468858954510736, 14.12814564770236991 ) ) ;
#36295=FACE_OUTER_BOUND ( 'NONE', #50091, .T. ) ;
#36297=CARTESIAN_POINT ( 'NONE',  ( 185.4166944662832179, 215.0000000000000568, 23.37680765314684095 ) ) ;
#36300=ORIENTED_EDGE ( 'NONE', *, *, #53136, .T. ) ;
#36301=DIRECTION ( 'NONE',  ( 1.000000000000000000, 0.000000000000000000, 0.000000000000000000 ) ) ;
#36316=DIRECTION ( 'NONE',  ( 0.000000000000000000, 0.000000000000000000, 1.000000000000000000 ) ) ;
#36317=EDGE_CURVE ( 'NONE', #38347, #68325, #65603, .T. ) ;
#36339=LINE ( 'NONE', #14120, #92808 ) ;
#36342=DIRECTION ( 'NONE',  ( 0.000000000000000000, 0.000000000000000000, -1.000000000000000000 ) ) ;
#36344=ADVANCED_FACE ( 'NONE', ( #81947 ), #2442, .F. ) ;
#36354=AXIS2_PLACEMENT_3D ( 'NONE', #6563, #5628, #42043 ) ;
#36356=B_SPLINE_CURVE_WITH_KNOTS ( 'NONE', 3,
 ( #21151, #57162, #56216, #35830, #63342, #27809 ),
 .UNSPECIFIED., .F., .F.,
 ( 4, 2, 4 ),
 ( 0.000000000000000000, 0.001588326293797077092, 0.003176652587594154184 ),
 .UNSPECIFIED. ) ;
#36358=EDGE_LOOP ( 'NONE', ( #19150, #54542, #38939, #56183 ) ) ;
#36361=FACE_OUTER_BOUND ( 'NONE', #64581, .T. ) ;
#36371=EDGE_LOOP ( 'NONE', ( #54611, #52907, #75468, #7871 ) ) ;
#36372=DIRECTION ( 'NONE',  ( -0.000000000000000000, -0.000000000000000000, 1.000000000000000000 ) ) ;
#36378=ADVANCED_FACE ( 'NONE', ( #17105 ), #10912, .T. ) ;
#36384=CARTESIAN_POINT ( 'NONE',  ( 197.6900603589809009, 68.42838418738361383, -10.08352334802372496 ) ) ;
#36385=LINE ( 'NONE', #51049, #73489 ) ;
#36389=ORIENTED_EDGE ( 'NONE', *, *, #53514, .F. ) ;
#36406=CARTESIAN_POINT ( 'NONE',  ( 175.2296996224750103, 133.0000000000000000, 0.000000000000000000 ) ) ;
#36421=VERTEX_POINT ( 'NONE', #74386 ) ;
#36422=DIRECTION ( 'NONE',  ( 0.000000000000000000, 0.000000000000000000, 1.000000000000000000 ) ) ;
#36433=CIRCLE ( 'NONE', #71258, 2.999999999999997780 ) ;
#36438=DIRECTION ( 'NONE',  ( 0.000000000000000000, 1.000000000000000000, 0.000000000000000000 ) ) ;
#36450=CARTESIAN_POINT ( 'NONE',  ( 202.8019728163925492, 61.40723988820082013, 8.999999999999994671 ) ) ;
#36458=DIRECTION ( 'NONE',  ( -5.880589007913310608E-16, 0.000000000000000000, 1.000000000000000000 ) ) ;
#36461=CARTESIAN_POINT ( 'NONE',  ( 175.2296996224750103, 134.0000000000000284, 0.000000000000000000 ) ) ;
#36462=FACE_OUTER_BOUND ( 'NONE', #25091, .T. ) ;
#36468=ADVANCED_FACE ( 'NONE', ( #3351 ), #446, .T. ) ;
#36471=ORIENTED_EDGE ( 'NONE', *, *, #88813, .F. ) ;
#36487=LINE ( 'NONE', #85741, #2770 ) ;
#36488=EDGE_CURVE ( 'NONE', #40445, #76858, #32306, .T. ) ;
#36500=ORIENTED_EDGE ( 'NONE', *, *, #69967, .F. ) ;
#36505=EDGE_CURVE ( 'NONE', #75307, #73161, #51773, .T. ) ;
#36515=CARTESIAN_POINT ( 'NONE',  ( 208.1233865313629394, 36.80875831278186183, 13.45150779440604794 ) ) ;
#36526=ORIENTED_EDGE ( 'NONE', *, *, #36918, .T. ) ;
#36527=DIRECTION ( 'NONE',  ( 0.000000000000000000, 1.000000000000000000, 0.000000000000000000 ) ) ;
#36538=CARTESIAN_POINT ( 'NONE',  ( 204.6539576904058606, 287.9062406767683910, -5.225551010890931103 ) ) ;
#36553=CARTESIAN_POINT ( 'NONE',  ( 199.3803347170859865, 17.19615242270659294, -9.999999999999994671 ) ) ;
#36562=CIRCLE ( 'NONE', #65334, 2.999999999999993783 ) ;
#36564=DIRECTION ( 'NONE',  ( 0.000000000000000000, 1.000000000000000000, 0.000000000000000000 ) ) ;
#36567=CARTESIAN_POINT ( 'NONE',  ( 208.0514444522711131, 35.78458379568167658, 14.36594018319230592 ) ) ;
#36568=DIRECTION ( 'NONE',  ( -1.000000000000000000, 0.000000000000000000, 0.000000000000000000 ) ) ;
#36576=ADVANCED_FACE ( 'NONE', ( #56374 ), #88185, .T. ) ;
#36578=ORIENTED_EDGE ( 'NONE', *, *, #43123, .F. ) ;
#36583=VERTEX_POINT ( 'NONE', #61602 ) ;
#36590=VERTEX_POINT ( 'NONE', #5714 ) ;
#36594=CARTESIAN_POINT ( 'NONE',  ( 196.7032892706336895, 294.4729419525710341, -7.987695993747508716 ) ) ;
#36597=FACE_OUTER_BOUND ( 'NONE', #18935, .T. ) ;
#36611=ORIENTED_EDGE ( 'NONE', *, *, #84552, .T. ) ;
#36614=ORIENTED_EDGE ( 'NONE', *, *, #19380, .F. ) ;
#36623=AXIS2_PLACEMENT_3D ( 'NONE', #92071, #4048, #32918 ) ;
#36634=ORIENTED_EDGE ( 'NONE', *, *, #54849, .F. ) ;
#36636=TOROIDAL_SURFACE ( 'NONE', #20008, 24.50000000000000355, 0.5000000000000000000 ) ;
#36645=ADVANCED_FACE ( 'NONE', ( #12831 ), #19901, .T. ) ;
#36655=DIRECTION ( 'NONE',  ( 0.000000000000000000, 0.000000000000000000, 1.000000000000000000 ) ) ;
#36658=( BOUNDED_CURVE ( )  B_SPLINE_CURVE ( 3, ( #46829, #82824, #93213, #35469 ),
 .UNSPECIFIED., .F., .F. ) 
 B_SPLINE_CURVE_WITH_KNOTS ( ( 4, 4 ),
 ( 4.712388980384695003, 7.853981633974477461 ),
 .UNSPECIFIED. ) 
 CURVE ( )  GEOMETRIC_REPRESENTATION_ITEM ( )  RATIONAL_B_SPLINE_CURVE ( ( 1.000000000000000000, 0.3333333333333369231, 0.3333333333333369231, 1.000000000000000000 ) ) 
 REPRESENTATION_ITEM ( '' )  );
#36661=CARTESIAN_POINT ( 'NONE',  ( 207.9853864603112470, 36.43026381062074393, 14.84047931273563847 ) ) ;
#36662=( BOUNDED_SURFACE ( )  B_SPLINE_SURFACE ( 3, 2, ( 
 ( #92182, #27337, #5098 ),
 ( #13605, #56224, #69957 ),
 ( #43849, #36294, #29673 ),
 ( #64755, #65211, #79406 ),
 ( #315, #21628, #93580 ),
 ( #87398, #15927, #1244 ),
 ( #7413, #6499, #14542 ),
 ( #72292, #29199, #80309 ) ),
 .UNSPECIFIED., .F., .F., .F. ) 
 B_SPLINE_SURFACE_WITH_KNOTS ( ( 4, 2, 2, 4 ),
 ( 3, 3 ),
 ( 0.005169333131382364971, 0.006119585499877708973, 0.006594711684125380974, 0.007069837868373052975 ),
 ( 0.000000000000000000, 0.8323599711382757560 ),
 .UNSPECIFIED. ) 
 GEOMETRIC_REPRESENTATION_ITEM ( )  RATIONAL_B_SPLINE_SURFACE ( (
 ( 1.000000000000000000, 0.7562074088418379025, 0.9182612059639423396),
 ( 1.000000000000000000, 0.7715893842249162971, 0.9234184755582816040),
 ( 1.000000000000000000, 0.7884922460007639522, 0.9290856680301792236),
 ( 1.000000000000000000, 0.8086550841627961894, 0.9358458655730139686),
 ( 1.000000000000000000, 0.8144484737901919180, 0.9377882735817015813),
 ( 1.000000000000000000, 0.8225010067395548408, 0.9404881272937839487),
 ( 1.000000000000000000, 0.8247405859259469008, 0.9412390135326735852),
 ( 1.000000000000000000, 0.8247174150534301029, 0.9412312448011987964) ) ) 
 REPRESENTATION_ITEM ( '' )  SURFACE ( )  );
#36668=DIRECTION ( 'NONE',  ( 1.000000000000000000, 0.000000000000000000, -0.000000000000000000 ) ) ;
#36671=CARTESIAN_POINT ( 'NONE',  ( 194.3522748274950231, 20.00000000000003908, 14.59659268673782506 ) ) ;
#36674=CARTESIAN_POINT ( 'NONE',  ( 198.6884013828325521, 64.61450673763174279, -9.555809373750800972 ) ) ;
#36686=CIRCLE ( 'NONE', #88103, 0.4999999999999989453 ) ;
#36691=CARTESIAN_POINT ( 'NONE',  ( 208.5780117385097014, 37.30339377898572195, 12.92477606492831477 ) ) ;
#36693=EDGE_CURVE ( 'NONE', #30954, #72640, #77201, .T. ) ;
#36695=EDGE_CURVE ( 'NONE', #49216, #48324, #79171, .T. ) ;
#36698=CIRCLE ( 'NONE', #39702, 1.000000000000000888 ) ;
#36715=B_SPLINE_CURVE_WITH_KNOTS ( 'NONE', 3,
 ( #72329, #93615, #351, #34938, #42018, #56746 ),
 .UNSPECIFIED., .F., .F.,
 ( 4, 2, 4 ),
 ( 0.000000000000000000, 0.0005961333682660641207, 0.001192266736532128241 ),
 .UNSPECIFIED. ) ;
#36747=VERTEX_POINT ( 'NONE', #78155 ) ;
#36748=CARTESIAN_POINT ( 'NONE',  ( 139.1539576904058606, 275.5000000000000568, -10.49999999999999822 ) ) ;
#36749=AXIS2_PLACEMENT_3D ( 'NONE', #41054, #62418, #10797 ) ;
#36752=AXIS2_PLACEMENT_3D ( 'NONE', #29330, #93248, #36422 ) ;
#36759=AXIS2_PLACEMENT_3D ( 'NONE', #47035, #60812, #19578 ) ;
#36764=VERTEX_POINT ( 'NONE', #47832 ) ;
#36767=CIRCLE ( 'NONE', #32238, 0.5000000000000004441 ) ;
#36777=VECTOR ( 'NONE', #15963, 1000.000000000000000 ) ;
#36783=AXIS2_PLACEMENT_3D ( 'NONE', #54393, #3755, #69543 ) ;
#36791=DIRECTION ( 'NONE',  ( 0.000000000000000000, 1.000000000000000000, 0.000000000000000000 ) ) ;
#36798=DIRECTION ( 'NONE',  ( -0.000000000000000000, -0.000000000000000000, -1.000000000000000000 ) ) ;
#36817=VECTOR ( 'NONE', #7329, 1000.000000000000000 ) ;
#36821=EDGE_CURVE ( 'NONE', #24854, #31130, #3835, .T. ) ;
#36822=AXIS2_PLACEMENT_3D ( 'NONE', #52500, #52964, #81377 ) ;
#36825=CARTESIAN_POINT ( 'NONE',  ( 197.3616393129065898, 72.09241014521839475, 11.67163425240527452 ) ) ;
#36826=TOROIDAL_SURFACE ( 'NONE', #36752, 24.50000000000000355, 0.5000000000000000000 ) ;
#36828=CARTESIAN_POINT ( 'NONE',  ( 185.8264795993290193, 250.5000000000000568, 23.09031830825835385 ) ) ;
#36834=CIRCLE ( 'NONE', #71667, 0.5000000000000004441 ) ;
#36837=UNCERTAINTY_MEASURE_WITH_UNIT (LENGTH_MEASURE( 1.000000000000000082E-05 ), #76509, 'distance_accuracy_value', 'NONE');
#36839=EDGE_LOOP ( 'NONE', ( #77606, #15709, #75972, #24644 ) ) ;
#36840=CARTESIAN_POINT ( 'NONE',  ( 196.0351550650564434, 41.34106363718652943, 11.96389409883855848 ) ) ;
#36851=DIRECTION ( 'NONE',  ( 0.000000000000000000, 0.000000000000000000, -1.000000000000000000 ) ) ;
#36853=DIRECTION ( 'NONE',  ( 1.000000000000000000, 0.000000000000000000, 0.000000000000000000 ) ) ;
#36857=EDGE_LOOP ( 'NONE', ( #18090, #39877 ) ) ;
#36887=ORIENTED_EDGE ( 'NONE', *, *, #60388, .T. ) ;
#36889=CARTESIAN_POINT ( 'NONE',  ( 195.8507069399275053, 41.77510181472468531, 14.13525600223613310 ) ) ;
#36904=CARTESIAN_POINT ( 'NONE',  ( 153.6949411230407918, 20.34881949282723923, -12.70049028465532182 ) ) ;
#36913=CARTESIAN_POINT ( 'NONE',  ( 183.0442525570908288, 296.7472757692770529, -7.499999999999996447 ) ) ;
#36916=AXIS2_PLACEMENT_3D ( 'NONE', #43824, #15904, #80286 ) ;
#36918=EDGE_CURVE ( 'NONE', #75392, #52994, #77675, .T. ) ;
#36919=CARTESIAN_POINT ( 'NONE',  ( 175.2296996224750103, 160.0000000000000568, -10.55076157886938937 ) ) ;
#36921=CARTESIAN_POINT ( 'NONE',  ( 150.8012326218627948, 131.0000000000000568, 11.50000000000000000 ) ) ;
#36934=DIRECTION ( 'NONE',  ( 0.000000000000000000, 1.000000000000000000, 0.000000000000000000 ) ) ;
#36943=ORIENTED_EDGE ( 'NONE', *, *, #81253, .T. ) ;
#36944=CARTESIAN_POINT ( 'NONE',  ( 200.4871970924047275, 61.71654497091388691, -9.999999999999998224 ) ) ;
#36961=CARTESIAN_POINT ( 'NONE',  ( 185.4166944662832179, 250.5000000000000568, 23.37680765314684450 ) ) ;
#36974=TOROIDAL_SURFACE ( 'NONE', #88330, 1.000000000000000000, 0.5000000000000000000 ) ;
#36998=ORIENTED_EDGE ( 'NONE', *, *, #38856, .T. ) ;
#36999=CARTESIAN_POINT ( 'NONE',  ( 194.6960821673052919, 25.58662921606750018, 14.03832098086475710 ) ) ;
#37022=CARTESIAN_POINT ( 'NONE',  ( 195.2074068093847075, 24.86248909206367941, 13.30112067542677146 ) ) ;
#37028=DIRECTION ( 'NONE',  ( 0.000000000000000000, 0.000000000000000000, -1.000000000000000000 ) ) ;
#37030=CARTESIAN_POINT ( 'NONE',  ( 197.7335303680046650, 24.96166607582782859, 12.00000000000001599 ) ) ;
#37033=CARTESIAN_POINT ( 'NONE',  ( 195.3536225096696342, 25.92713179672681179, 14.83384749020537718 ) ) ;
#37034=CYLINDRICAL_SURFACE ( 'NONE', #18572, 25.00000000000000355 ) ;
#37042=EDGE_CURVE ( 'NONE', #33465, #50614, #20389, .T. ) ;
#37046=CARTESIAN_POINT ( 'NONE',  ( 208.6208076322478746, 32.98517505407394168, 10.50000000000000000 ) ) ;
#37050=( GEOMETRIC_REPRESENTATION_CONTEXT ( 3 ) GLOBAL_UNCERTAINTY_ASSIGNED_CONTEXT ( ( #65568 ) ) GLOBAL_UNIT_ASSIGNED_CONTEXT ( ( #41729, #13350, #533 ) ) REPRESENTATION_CONTEXT ( 'NONE', 'WORKASPACE' ) );
#37055=VECTOR ( 'NONE', #85639, 1000.000000000000000 ) ;
#37064=CARTESIAN_POINT ( 'NONE',  ( 155.0741174296433371, 18.62644422905808383, 11.41100038914543902 ) ) ;
#37067=DIRECTION ( 'NONE',  ( 1.000000000000000000, -0.000000000000000000, 0.000000000000000000 ) ) ;
#37081=ORIENTED_EDGE ( 'NONE', *, *, #80410, .F. ) ;
#37084=ORIENTED_EDGE ( 'NONE', *, *, #93228, .T. ) ;
#37103=VERTEX_POINT ( 'NONE', #4292 ) ;
#37114=ORIENTED_EDGE ( 'NONE', *, *, #27099, .T. ) ;
#37125=CARTESIAN_POINT ( 'NONE',  ( 157.5411741086738004, 250.0000000000000568, 16.22085278731065472 ) ) ;
#37128=VECTOR ( 'NONE', #93669, 1000.000000000000114 ) ;
#37131=DIRECTION ( 'NONE',  ( -0.000000000000000000, -1.000000000000000000, -0.000000000000000000 ) ) ;
#37140=DIRECTION ( 'NONE',  ( -0.000000000000000000, -0.000000000000000000, -1.000000000000000000 ) ) ;
#37142=CARTESIAN_POINT ( 'NONE',  ( 158.3977298502249766, 17.52828139914420191, -10.67961748035033587 ) ) ;
#37181=DIRECTION ( 'NONE',  ( -1.000000000000000000, -0.000000000000000000, -0.000000000000000000 ) ) ;
#37191=CIRCLE ( 'NONE', #49288, 24.00000000000000355 ) ;
#37217=DIRECTION ( 'NONE',  ( 0.9452808130703184153, -0.000000000000000000, -0.3262578496237564796 ) ) ;
#37222=ADVANCED_FACE ( 'NONE', ( #11861 ), #5254, .T. ) ;
#37223=DIRECTION ( 'NONE',  ( 0.000000000000000000, 0.000000000000000000, 1.000000000000000000 ) ) ;
#37224=EDGE_CURVE ( 'NONE', #69256, #92724, #76610, .T. ) ;
#37225=DIRECTION ( 'NONE',  ( 0.000000000000000000, 1.000000000000000000, 0.000000000000000000 ) ) ;
#37230=ORIENTED_EDGE ( 'NONE', *, *, #18442, .T. ) ;
#37231=DIRECTION ( 'NONE',  ( 0.000000000000000000, -0.000000000000000000, 1.000000000000000000 ) ) ;
#37244=CARTESIAN_POINT ( 'NONE',  ( 210.2447652224009573, 1.019566348684628698, -7.291626467228960351 ) ) ;
#37257=DIRECTION ( 'NONE',  ( 0.000000000000000000, 0.000000000000000000, 1.000000000000000000 ) ) ;
#37259=CARTESIAN_POINT ( 'NONE',  ( 219.8344101925596021, 0.000000000000000000, -7.000000000000000888 ) ) ;
#37265=CARTESIAN_POINT ( 'NONE',  ( 208.1147618731698401, 29.48222340873819292, 14.79012820594046218 ) ) ;
#37280=VERTEX_POINT ( 'NONE', #27971 ) ;
#37281=CARTESIAN_POINT ( 'NONE',  ( 198.9495682819174647, 68.47409081099804951, 9.196090786366733383 ) ) ;
#37304=DIRECTION ( 'NONE',  ( 0.4999999999999967248, 0.8660254037844404840, 0.000000000000000000 ) ) ;
#37305=CARTESIAN_POINT ( 'NONE',  ( 0.000000000000000000, 0.000000000000000000, 13.99999999999999112 ) ) ;
#37322=DIRECTION ( 'NONE',  ( -0.000000000000000000, -1.000000000000000000, -0.000000000000000000 ) ) ;
#37326=CARTESIAN_POINT ( 'NONE',  ( 196.7806748523260012, 214.5000000000000568, -12.67104836398113576 ) ) ;
#37336=CARTESIAN_POINT ( 'NONE',  ( 197.8059408385280165, 70.97274906999653865, -10.93303304242674656 ) ) ;
#37340=ORIENTED_EDGE ( 'NONE', *, *, #77632, .T. ) ;
#37341=VERTEX_POINT ( 'NONE', #20848 ) ;
#37342=CARTESIAN_POINT ( 'NONE',  ( 200.2454457599218927, 15.96501597607006850, -10.07064028581557835 ) ) ;
#37364=DIRECTION ( 'NONE',  ( 0.000000000000000000, 0.000000000000000000, -1.000000000000000000 ) ) ;
#37390=ORIENTED_EDGE ( 'NONE', *, *, #81666, .T. ) ;
#37391=CARTESIAN_POINT ( 'NONE',  ( 201.2104617360081704, 60.19600395700752671, -9.999999999999998224 ) ) ;
#37394=LINE ( 'NONE', #59675, #45829 ) ;
#37406=DIRECTION ( 'NONE',  ( -0.3024135303179394940, -0.9531768234072001134, 0.000000000000000000 ) ) ;
#37410=LINE ( 'NONE', #30319, #22837 ) ;
#37427=ORIENTED_EDGE ( 'NONE', *, *, #24079, .F. ) ;
#37435=CARTESIAN_POINT ( 'NONE',  ( 185.4166944662832179, 275.5000000000000568, 23.37680765314684450 ) ) ;
#37438=EDGE_CURVE ( 'NONE', #85642, #69004, #5153, .T. ) ;
#37446=ORIENTED_EDGE ( 'NONE', *, *, #90775, .F. ) ;
#37447=CARTESIAN_POINT ( 'NONE',  ( 220.4471435719830197, 34.91984470236808136, -7.000000000000000888 ) ) ;
#37456=LINE ( 'NONE', #51658, #61137 ) ;
#37470=CARTESIAN_POINT ( 'NONE',  ( 153.8059597141930510, 20.39660080186459723, 12.88664367905129104 ) ) ;
#37476=DIRECTION ( 'NONE',  ( -1.000000000000000000, 0.000000000000000000, 0.000000000000000000 ) ) ;
#37481=CARTESIAN_POINT ( 'NONE',  ( 195.0811277904324754, 27.48493576247232895, 15.19607843137254477 ) ) ;
#37492=VERTEX_POINT ( 'NONE', #43094 ) ;
#37493=FACE_OUTER_BOUND ( 'NONE', #39336, .T. ) ;
#37496=DIRECTION ( 'NONE',  ( 0.000000000000000000, 0.000000000000000000, 1.000000000000000000 ) ) ;
#37508=DIRECTION ( 'NONE',  ( 0.000000000000000000, 0.000000000000000000, -1.000000000000000000 ) ) ;
#37524=ORIENTED_EDGE ( 'NONE', *, *, #67573, .F. ) ;
#37527=EDGE_LOOP ( 'NONE', ( #7874, #51537, #75848, #15666 ) ) ;
#37538=ORIENTED_EDGE ( 'NONE', *, *, #28382, .T. ) ;
#37549=ORIENTED_EDGE ( 'NONE', *, *, #84148, .F. ) ;
#37556=ORIENTED_EDGE ( 'NONE', *, *, #69734, .T. ) ;
#37557=CARTESIAN_POINT ( 'NONE',  ( 157.2832821354283794, 16.68119283998523272, 9.201835683359835372 ) ) ;
#37561=ORIENTED_EDGE ( 'NONE', *, *, #55070, .F. ) ;
#37569=ADVANCED_FACE ( 'NONE', ( #93275 ), #76178, .T. ) ;
#37573=CARTESIAN_POINT ( 'NONE',  ( 193.9646936176701786, 21.00000000000000000, -15.00000000000000000 ) ) ;
#37578=DIRECTION ( 'NONE',  ( 0.000000000000000000, 0.000000000000000000, -1.000000000000000000 ) ) ;
#37584=CARTESIAN_POINT ( 'NONE',  ( 164.2231345125756263, 296.7472757692770529, 7.499999999999996447 ) ) ;
#37587=CARTESIAN_POINT ( 'NONE',  ( 165.2494399300530290, 8.542400036368780647, -9.000000000000001776 ) ) ;
#37590=DIRECTION ( 'NONE',  ( -0.000000000000000000, -1.000000000000000000, -0.000000000000000000 ) ) ;
#37594=CARTESIAN_POINT ( 'NONE',  ( 197.3133474189782248, 42.36571313990103960, 12.74999999999998757 ) ) ;
#37606=DIRECTION ( 'NONE',  ( 1.000000000000000000, -0.000000000000000000, -0.000000000000000000 ) ) ;
#37625=ADVANCED_FACE ( 'NONE', ( #71999 ), #7118, .T. ) ;
#37647=ADVANCED_FACE ( 'NONE', ( #6181 ), #3469, .F. ) ;
#37650=LINE ( 'NONE', #81671, #73222 ) ;
#37664=VERTEX_POINT ( 'NONE', #15142 ) ;
#37665=FACE_OUTER_BOUND ( 'NONE', #42279, .T. ) ;
#37677=EDGE_LOOP ( 'NONE', ( #56184, #87929, #19257, #43737 ) ) ;
#37678=CARTESIAN_POINT ( 'NONE',  ( 197.3133474189782248, 24.42324672360810212, 12.74999999999999112 ) ) ;
#37681=ADVANCED_FACE ( 'NONE', ( #8025 ), #80770, .F. ) ;
#37701=DIRECTION ( 'NONE',  ( 0.000000000000000000, 0.000000000000000000, 1.000000000000000000 ) ) ;
#37702=CARTESIAN_POINT ( 'NONE',  ( 164.7123623445222904, 2.999999999999999112, 9.000000000000001776 ) ) ;
#37707=DIRECTION ( 'NONE',  ( 0.9693563597868444237, 0.2456588035076248677, 0.000000000000000000 ) ) ;
#37710=CARTESIAN_POINT ( 'NONE',  ( 159.4851178187871312, 0.000000000000000000, 7.000000000000000000 ) ) ;
#37732=ORIENTED_EDGE ( 'NONE', *, *, #4248, .F. ) ;
#37733=CARTESIAN_POINT ( 'NONE',  ( 197.8752062525135500, 68.08088840871901937, 11.26666408104508577 ) ) ;
#37744=ORIENTED_EDGE ( 'NONE', *, *, #66611, .T. ) ;
#37745=CARTESIAN_POINT ( 'NONE',  ( 195.8198161289002712, 42.34889664205514492, 12.33687207710887357 ) ) ;
#37753=AXIS2_PLACEMENT_3D ( 'NONE', #53934, #32635, #33546 ) ;
#37762=ORIENTED_EDGE ( 'NONE', *, *, #58566, .T. ) ;
#37788=CARTESIAN_POINT ( 'NONE',  ( 197.7953982265470927, 19.09807621135331246, 10.91506350946108839 ) ) ;
#37792=ORIENTED_EDGE ( 'NONE', *, *, #17570, .T. ) ;
#37808=FACE_OUTER_BOUND ( 'NONE', #39837, .T. ) ;
#37817=CARTESIAN_POINT ( 'NONE',  ( 175.2296996224750103, 250.0000000000000568, 0.000000000000000000 ) ) ;
#37823=AXIS2_PLACEMENT_3D ( 'NONE', #25971, #46806, #61525 ) ;
#37824=DIRECTION ( 'NONE',  ( 1.000000000000000000, 0.000000000000000000, 0.000000000000000000 ) ) ;
#37846=CARTESIAN_POINT ( 'NONE',  ( 165.4421947725420523, 250.0000000000000568, 22.46007009812166544 ) ) ;
#37849=DIRECTION ( 'NONE',  ( -1.000000000000000000, 0.000000000000000000, 0.000000000000000000 ) ) ;
#37860=ORIENTED_EDGE ( 'NONE', *, *, #28287, .T. ) ;
#37875=EDGE_LOOP ( 'NONE', ( #40306, #14205, #44535, #3978 ) ) ;
#37883=ORIENTED_EDGE ( 'NONE', *, *, #30742, .F. ) ;
#37890=CARTESIAN_POINT ( 'NONE',  ( 207.8064396648212551, 36.74001737686529623, 13.57731244650625690 ) ) ;
#37902=DIRECTION ( 'NONE',  ( -0.7957555401921962979, -0.6056179655966504871, 0.000000000000000000 ) ) ;
#37929=CYLINDRICAL_SURFACE ( 'NONE', #15405, 6.000000000000005329 ) ;
#37931=DIRECTION ( 'NONE',  ( 0.000000000000000000, 1.000000000000000000, 0.000000000000000000 ) ) ;
#37934=DIRECTION ( 'NONE',  ( 1.000000000000000000, 0.000000000000000000, 1.224646799147353207E-16 ) ) ;
#37935=FACE_OUTER_BOUND ( 'NONE', #55830, .T. ) ;
#37944=ORIENTED_EDGE ( 'NONE', *, *, #11892, .F. ) ;
#37949=CYLINDRICAL_SURFACE ( 'NONE', #91098, 5.000000000000000888 ) ;
#37962=CARTESIAN_POINT ( 'NONE',  ( 159.0442047513580235, 16.65459343288188521, 10.27557066714185119 ) ) ;
#37965=CARTESIAN_POINT ( 'NONE',  ( 157.4851178187871312, 15.00000000000000000, 7.000000000000000888 ) ) ;
#37992=ORIENTED_EDGE ( 'NONE', *, *, #55196, .T. ) ;
#37993=B_SPLINE_CURVE_WITH_KNOTS ( 'NONE', 3,
 ( #89995, #75341, #33651, #10457 ),
 .UNSPECIFIED., .F., .F.,
 ( 4, 4 ),
 ( 2.907926436840383405E-17, 9.632970524407232079E-05 ),
 .UNSPECIFIED. ) ;
#38003=EDGE_LOOP ( 'NONE', ( #42815, #69715, #79264, #75142, #84567, #32330 ) ) ;
#38010=ORIENTED_EDGE ( 'NONE', *, *, #22499, .F. ) ;
#38011=CARTESIAN_POINT ( 'NONE',  ( 159.4851178187871312, 14.99999999999999467, 9.000000000000001776 ) ) ;
#38015=EDGE_LOOP ( 'NONE', ( #3085, #63888, #10385, #57156, #32848, #82813 ) ) ;
#38023=AXIS2_PLACEMENT_3D ( 'NONE', #51796, #73600, #2094 ) ;
#38027=CARTESIAN_POINT ( 'NONE',  ( 193.8285826777556906, 214.7033826592484900, 16.75079304138583325 ) ) ;
#38030=CIRCLE ( 'NONE', #90927, 5.000000000000000888 ) ;
#38041=CARTESIAN_POINT ( 'NONE',  ( 156.4851178187871312, 15.00000000000000000, -10.00000000000000000 ) ) ;
#38044=DIRECTION ( 'NONE',  ( -1.110223024625156383E-14, 0.000000000000000000, 1.000000000000000000 ) ) ;
#38048=CARTESIAN_POINT ( 'NONE',  ( 199.2296996224750103, 68.12454877777268791, 0.000000000000000000 ) ) ;
#38066=CARTESIAN_POINT ( 'NONE',  ( 198.1425780972542157, 15.00000000000000000, -10.00000000000000000 ) ) ;
#38069=CARTESIAN_POINT ( 'NONE',  ( 208.3435665664548253, 37.37777598216731434, 12.00000000000000000 ) ) ;
#38083=EDGE_CURVE ( 'NONE', #63583, #26188, #44930, .T. ) ;
#38087=CARTESIAN_POINT ( 'NONE',  ( 175.2296996224750103, 161.0000000000000853, -9.550761578869391144 ) ) ;
#38099=TOROIDAL_SURFACE ( 'NONE', #72932, 1.000000000000000000, 0.5000000000000000000 ) ;
#38102=ORIENTED_EDGE ( 'NONE', *, *, #60850, .T. ) ;
#38123=EDGE_LOOP ( 'NONE', ( #16201, #12681, #38915, #36614 ) ) ;
#38124=CARTESIAN_POINT ( 'NONE',  ( 155.7140808774800007, 20.99999999999998934, -15.62500000000000711 ) ) ;
#38130=CARTESIAN_POINT ( 'NONE',  ( 222.2216768131362130, 37.54180348216212337, -7.000000000000000888 ) ) ;
#38135=ORIENTED_EDGE ( 'NONE', *, *, #85924, .T. ) ;
#38136=CARTESIAN_POINT ( 'NONE',  ( 164.2231345125756263, 275.0000000000000568, 20.22542485937379908 ) ) ;
#38145=AXIS2_PLACEMENT_3D ( 'NONE', #54683, #13042, #19644 ) ;
#38152=CIRCLE ( 'NONE', #18499, 24.00000000000001066 ) ;
#38153=CARTESIAN_POINT ( 'NONE',  ( 0.000000000000000000, 3.000000000000000000, 7.000000000000000000 ) ) ;
#38155=AXIS2_PLACEMENT_3D ( 'NONE', #76371, #12432, #92419 ) ;
#38163=DIRECTION ( 'NONE',  ( 0.000000000000000000, 0.000000000000000000, 1.000000000000000000 ) ) ;
#38164=FACE_OUTER_BOUND ( 'NONE', #38003, .T. ) ;
#38171=EDGE_CURVE ( 'NONE', #3443, #77260, #38294, .T. ) ;
#38173=CARTESIAN_POINT ( 'NONE',  ( 197.3748232817349049, 250.5000000000000568, -12.45182892472559821 ) ) ;
#38186=AXIS2_PLACEMENT_3D ( 'NONE', #66405, #45998, #10474 ) ;
#38195=ADVANCED_FACE ( 'NONE', ( #73831 ), #23641, .T. ) ;
#38199=CARTESIAN_POINT ( 'NONE',  ( 200.1417227593101416, 66.37791233065237861, 9.866782148935371310 ) ) ;
#38201=CARTESIAN_POINT ( 'NONE',  ( 175.2296996224750103, 214.5000000000000568, 0.000000000000000000 ) ) ;
#38214=AXIS2_PLACEMENT_3D ( 'NONE', #89619, #24307, #46081 ) ;
#38225=CARTESIAN_POINT ( 'NONE',  ( 175.2296996224750103, 20.99999999999998934, 0.000000000000000000 ) ) ;
#38229=EDGE_LOOP ( 'NONE', ( #14718, #76352, #68658 ) ) ;
#38230=VECTOR ( 'NONE', #7683, 1000.000000000000000 ) ;
#38249=VECTOR ( 'NONE', #16417, 1000.000000000000114 ) ;
#38259=VECTOR ( 'NONE', #12971, 1000.000000000000000 ) ;
#38261=VERTEX_POINT ( 'NONE', #30746 ) ;
#38262=EDGE_LOOP ( 'NONE', ( #81295, #42747 ) ) ;
#38263=CARTESIAN_POINT ( 'NONE',  ( 198.0894686820296897, 18.12099305396623450, -11.05388702472888163 ) ) ;
#38287=CARTESIAN_POINT ( 'NONE',  ( 153.6987871352777404, 19.48326534539592458, 11.45812909364015297 ) ) ;
#38294=LINE ( 'NONE', #66278, #35369 ) ;
#38304=AXIS2_PLACEMENT_3D ( 'NONE', #41430, #66505, #80694 ) ;
#38307=LINE ( 'NONE', #83256, #11291 ) ;
#38313=VECTOR ( 'NONE', #90435, 1000.000000000000000 ) ;
#38318=ORIENTED_EDGE ( 'NONE', *, *, #51997, .F. ) ;
#38320=VECTOR ( 'NONE', #45746, 1000.000000000000000 ) ;
#38323=FACE_OUTER_BOUND ( 'NONE', #17517, .T. ) ;
#38334=DIRECTION ( 'NONE',  ( 0.000000000000000000, 0.000000000000000000, 1.000000000000000000 ) ) ;
#38335=ADVANCED_FACE ( 'NONE', ( #9409 ), #88946, .T. ) ;
#38336=DIRECTION ( 'NONE',  ( 0.000000000000000000, 1.000000000000000000, 0.000000000000000000 ) ) ;
#38339=DIRECTION ( 'NONE',  ( 0.000000000000000000, 1.000000000000000000, 0.000000000000000000 ) ) ;
#38347=VERTEX_POINT ( 'NONE', #60569 ) ;
#38363=CARTESIAN_POINT ( 'NONE',  ( 209.6160175266639669, 36.70030375927228761, 13.08022668053253668 ) ) ;
#38375=ORIENTED_EDGE ( 'NONE', *, *, #9862, .F. ) ;
#38376=CARTESIAN_POINT ( 'NONE',  ( 195.4471090089123777, 26.99502172241844633, 13.95936681960324854 ) ) ;
#38378=AXIS2_PLACEMENT_3D ( 'NONE', #84644, #62433, #90338 ) ;
#38388=AXIS2_PLACEMENT_3D ( 'NONE', #41654, #70571, #40235 ) ;
#38392=EDGE_CURVE ( 'NONE', #69141, #84950, #79959, .T. ) ;
#38393=EDGE_CURVE ( 'NONE', #135, #23299, #52042, .T. ) ;
#38396=AXIS2_PLACEMENT_3D ( 'NONE', #40517, #76545, #46699 ) ;
#38403=CARTESIAN_POINT ( 'NONE',  ( 196.2154913428680914, 25.52575416299670152, 11.66205930223015308 ) ) ;
#38410=DIRECTION ( 'NONE',  ( 0.000000000000000000, 0.000000000000000000, -1.000000000000000000 ) ) ;
#38412=DIRECTION ( 'NONE',  ( -1.000000000000000000, -0.000000000000000000, -0.000000000000000000 ) ) ;
#38415=CARTESIAN_POINT ( 'NONE',  ( 200.5094052069776467, 41.41475569182169636, 9.999999999999998224 ) ) ;
#38425=ORIENTED_EDGE ( 'NONE', *, *, #54408, .T. ) ;
#38430=CARTESIAN_POINT ( 'NONE',  ( 196.4890680266781828, 25.15197166163899922, 13.65125671900674753 ) ) ;
#38434=VECTOR ( 'NONE', #52505, 1000.000000000000000 ) ;
#38444=AXIS2_PLACEMENT_3D ( 'NONE', #7181, #19972, #57386 ) ;
#38445=CARTESIAN_POINT ( 'NONE',  ( 165.7865175155837676, 3.000000000000000000, 9.000000000000001776 ) ) ;
#38446=DIRECTION ( 'NONE',  ( 0.000000000000000000, 0.000000000000000000, 1.000000000000000000 ) ) ;
#38448=CARTESIAN_POINT ( 'NONE',  ( 161.2494399300530290, 8.542400036368780647, 10.00000000000000000 ) ) ;
#38450=CIRCLE ( 'NONE', #38388, 4.499999999999990230 ) ;
#38461=AXIS2_PLACEMENT_3D ( 'NONE', #90474, #19473, #41707 ) ;
#38465=VERTEX_POINT ( 'NONE', #17934 ) ;
#38468=ORIENTED_EDGE ( 'NONE', *, *, #93160, .F. ) ;
#38478=ORIENTED_EDGE ( 'NONE', *, *, #3777, .F. ) ;
#38489=ADVANCED_FACE ( 'NONE', ( #61506 ), #41408, .T. ) ;
#38498=CARTESIAN_POINT ( 'NONE',  ( 157.3811296300183642, 16.14910309754966278, 7.138650918358441899 ) ) ;
#38503=ORIENTED_EDGE ( 'NONE', *, *, #28819, .T. ) ;
#38519=CARTESIAN_POINT ( 'NONE',  ( 200.1126601882107252, 275.0000000000000568, -2.416251949619912853 ) ) ;
#38527=CARTESIAN_POINT ( 'NONE',  ( 196.4265994039971304, 19.73582633127739427, 13.26925245973608547 ) ) ;
#38529=AXIS2_PLACEMENT_3D ( 'NONE', #63322, #49548, #93100 ) ;
#38531=CARTESIAN_POINT ( 'NONE',  ( 175.2296996224750103, 140.2072866198470251, 0.000000000000000000 ) ) ;
#38534=AXIS2_PLACEMENT_3D ( 'NONE', #23678, #74809, #66767 ) ;
#38535=DIRECTION ( 'NONE',  ( 1.000000000000000000, 0.000000000000000000, 0.000000000000000000 ) ) ;
#38551=CYLINDRICAL_SURFACE ( 'NONE', #56038, 4.025000000000000355 ) ;
#38554=CARTESIAN_POINT ( 'NONE',  ( 189.9243309297870610, 250.0000000000000568, 20.22542485937349355 ) ) ;
#38583=ORIENTED_EDGE ( 'NONE', *, *, #3450, .F. ) ;
#38585=ORIENTED_EDGE ( 'NONE', *, *, #3741, .F. ) ;
#38606=ORIENTED_EDGE ( 'NONE', *, *, #38392, .F. ) ;
#38607=CARTESIAN_POINT ( 'NONE',  ( 197.9736226834741615, 68.21442376052006296, -9.114149584028082174 ) ) ;
#38609=EDGE_CURVE ( 'NONE', #11817, #17165, #62610, .T. ) ;
#38618=CARTESIAN_POINT ( 'NONE',  ( 175.2296996224750103, 160.0000000000000568, 10.55076157886938937 ) ) ;
#38620=EDGE_CURVE ( 'NONE', #70265, #69489, #55792, .T. ) ;
#38627=CARTESIAN_POINT ( 'NONE',  ( 190.2832783574276903, 8.542400036368780647, -9.000000000000001776 ) ) ;
#38633=CARTESIAN_POINT ( 'NONE',  ( 165.0427047786672290, 250.5000000000000568, 23.37680765314704701 ) ) ;
#38660=LINE ( 'NONE', #45749, #69949 ) ;
#38673=VERTEX_POINT ( 'NONE', #53914 ) ;
#38676=CARTESIAN_POINT ( 'NONE',  ( 209.6287663260176259, 29.00782453271233408, 12.09245862095555601 ) ) ;
#38685=VERTEX_POINT ( 'NONE', #91274 ) ;
#38686=LINE ( 'NONE', #54757, #22905 ) ;
#38695=DIRECTION ( 'NONE',  ( -0.000000000000000000, -1.000000000000000000, -0.000000000000000000 ) ) ;
#38696=DIRECTION ( 'NONE',  ( -0.000000000000000000, -1.000000000000000000, -0.000000000000000000 ) ) ;
#38713=DIRECTION ( 'NONE',  ( 1.000000000000000000, 0.000000000000000000, -0.000000000000000000 ) ) ;
#38716=ADVANCED_FACE ( 'NONE', ( #3732 ), #86777, .T. ) ;
#38717=DIRECTION ( 'NONE',  ( 1.110223024625155531E-13, 0.000000000000000000, 1.000000000000000000 ) ) ;
#38718=FACE_OUTER_BOUND ( 'NONE', #83972, .T. ) ;
#38730=ORIENTED_EDGE ( 'NONE', *, *, #69429, .F. ) ;
#38731=ORIENTED_EDGE ( 'NONE', *, *, #30742, .T. ) ;
#38732=CARTESIAN_POINT ( 'NONE',  ( 195.4937503561064887, 41.24039232090726870, 14.64184794398896194 ) ) ;
#38745=EDGE_CURVE ( 'NONE', #30715, #26935, #53535, .T. ) ;
#38748=CARTESIAN_POINT ( 'NONE',  ( 197.1098461824585968, 214.8820409514499090, -12.42446933126073816 ) ) ;
#38749=CARTESIAN_POINT ( 'NONE',  ( 155.8658175007533657, 19.96629232096022122, -14.32310887264409160 ) ) ;
#38763=DIRECTION ( 'NONE',  ( -0.6056179655966478226, 0.7957555401921982963, -0.000000000000000000 ) ) ;
#38773=LINE ( 'NONE', #74782, #49145 ) ;
#38783=ORIENTED_EDGE ( 'NONE', *, *, #15328, .T. ) ;
#38787=DIRECTION ( 'NONE',  ( 0.000000000000000000, -0.000000000000000000, 1.000000000000000000 ) ) ;
#38798=CARTESIAN_POINT ( 'NONE',  ( 175.2296996224750103, 250.0000000000000568, 0.000000000000000000 ) ) ;
#38801=FACE_OUTER_BOUND ( 'NONE', #24373, .T. ) ;
#38804=DIRECTION ( 'NONE',  ( -0.000000000000000000, -1.000000000000000000, 0.000000000000000000 ) ) ;
#38812=ORIENTED_EDGE ( 'NONE', *, *, #64104, .F. ) ;
#38820=ORIENTED_EDGE ( 'NONE', *, *, #9944, .F. ) ;
#38826=CYLINDRICAL_SURFACE ( 'NONE', #91430, 9.103929867429224387 ) ;
#38838=VECTOR ( 'NONE', #84692, 1000.000000000000000 ) ;
#38856=EDGE_CURVE ( 'NONE', #64501, #55580, #42927, .T. ) ;
#38858=CARTESIAN_POINT ( 'NONE',  ( 159.4851178187871312, 17.02694846567612075, 9.999999999999998224 ) ) ;
#38860=CARTESIAN_POINT ( 'NONE',  ( 194.2870706637141325, 27.48493576247232184, 14.58823529411763431 ) ) ;
#38872=CARTESIAN_POINT ( 'NONE',  ( 221.8344101925596306, 1.000000000000000222, -7.000000000000000888 ) ) ;
#38881=ORIENTED_EDGE ( 'NONE', *, *, #34457, .T. ) ;
#38897=CARTESIAN_POINT ( 'NONE',  ( 155.5427215445328386, 17.93151222991971139, 8.507834038804169552 ) ) ;
#38915=ORIENTED_EDGE ( 'NONE', *, *, #54472, .T. ) ;
#38923=CARTESIAN_POINT ( 'NONE',  ( 195.4197218357614361, 19.73101387165973364, -13.32484321907415747 ) ) ;
#38928=ORIENTED_EDGE ( 'NONE', *, *, #63047, .T. ) ;
#38939=ORIENTED_EDGE ( 'NONE', *, *, #19590, .T. ) ;
#38946=ORIENTED_EDGE ( 'NONE', *, *, #14513, .F. ) ;
#38947=DIRECTION ( 'NONE',  ( 0.000000000000000000, 0.000000000000000000, 1.000000000000000000 ) ) ;
#38962=FACE_OUTER_BOUND ( 'NONE', #14336, .T. ) ;
#38967=CARTESIAN_POINT ( 'NONE',  ( 150.8012326218627948, 131.0000000000000568, 11.50000000000000000 ) ) ;
#38970=ADVANCED_FACE ( 'NONE', ( #55331 ), #55014, .T. ) ;
#38993=ORIENTED_EDGE ( 'NONE', *, *, #58451, .F. ) ;
#38999=CARTESIAN_POINT ( 'NONE',  ( 189.9243309297870610, 250.0000000000000568, 20.22542485937349355 ) ) ;
#39017=DIRECTION ( 'NONE',  ( -0.000000000000000000, -0.000000000000000000, -1.000000000000000000 ) ) ;
#39026=ADVANCED_FACE ( 'NONE', ( #61958 ), #50499, .T. ) ;
#39031=ORIENTED_EDGE ( 'NONE', *, *, #57561, .T. ) ;
#39033=ORIENTED_EDGE ( 'NONE', *, *, #71157, .F. ) ;
#39039=VECTOR ( 'NONE', #24132, 1000.000000000000000 ) ;
#39065=PLANE ( 'NONE',  #47484 ) ;
#39087=CARTESIAN_POINT ( 'NONE',  ( 197.0471578326374527, 42.02301189210707122, 12.21301650322624432 ) ) ;
#39092=CARTESIAN_POINT ( 'NONE',  ( 151.6916247871641303, 20.99999999999999645, -4.896253172919318608 ) ) ;
#39095=CARTESIAN_POINT ( 'NONE',  ( 175.2296996224750103, 20.99999999999998934, 0.000000000000000000 ) ) ;
#39096=VECTOR ( 'NONE', #63622, 1000.000000000000000 ) ;
#39109=( BOUNDED_SURFACE ( )  B_SPLINE_SURFACE ( 3, 2, ( 
 ( #33768, #62680, #19556 ),
 ( #48422, #32374, #11040 ),
 ( #61274, #25261, #83007 ),
 ( #39910, #68830, #86743 ),
 ( #42724, #12954, #21905 ),
 ( #27608, #21426, #49381 ),
 ( #29001, #72110, #7226 ),
 ( #79664, #20965, #77804 ) ),
 .UNSPECIFIED., .F., .F., .F. ) 
 B_SPLINE_SURFACE_WITH_KNOTS ( ( 4, 2, 2, 4 ),
 ( 3, 3 ),
 ( 0.005169333131380775964, 0.006119585499875557916, 0.006594711684122948891, 0.007069837868370339000 ),
 ( 0.1676400288617256873, 1.000000000000000000 ),
 .UNSPECIFIED. ) 
 GEOMETRIC_REPRESENTATION_ITEM ( )  RATIONAL_B_SPLINE_SURFACE ( (
 ( 0.9182612059639421176, 0.7562074088418391238, 1.000000000000000000),
 ( 0.9234184755582998116, 0.7715893842249726964, 1.000000000000000000),
 ( 0.9290856680301433634, 0.7884922460006588141, 1.000000000000000000),
 ( 0.9358458655730186315, 0.8086550841628119546, 1.000000000000000000),
 ( 0.9377882735816500670, 0.8144484737900394844, 1.000000000000000000),
 ( 0.9404881272938196979, 0.8225010067396629765, 1.000000000000000000),
 ( 0.9412390135326376139, 0.8247405859258407634, 1.000000000000000000),
 ( 0.9412312448011985744, 0.8247174150534309911, 1.000000000000000000) ) ) 
 REPRESENTATION_ITEM ( '' )  SURFACE ( )  );
#39117=( BOUNDED_SURFACE ( )  B_SPLINE_SURFACE ( 3, 2, ( 
 ( #76987, #41443, #41916 ),
 ( #12116, #85007, #20161 ),
 ( #40961, #36691, #43336 ),
 ( #87334, #78854, #35302 ),
 ( #93058, #14004, #79343 ),
 ( #85942, #73619, #72685 ) ),
 .UNSPECIFIED., .F., .F., .F. ) 
 B_SPLINE_SURFACE_WITH_KNOTS ( ( 4, 2, 4 ),
 ( 3, 3 ),
 ( 0.005169333131380775964, 0.006119585499875832002, 0.007069837868370888040 ),
 ( 0.4216207772072607107, 1.000000000000000000 ),
 .UNSPECIFIED. ) 
 GEOMETRIC_REPRESENTATION_ITEM ( )  RATIONAL_B_SPLINE_SURFACE ( (
 ( 0.8571520539184378507, 0.8305966477414123972, 1.000000000000000000),
 ( 0.8661649758441183344, 0.8412850701495542260, 1.000000000000000000),
 ( 0.8760690466613034744, 0.8530303058596961918, 1.000000000000000000),
 ( 0.8918213438905483459, 0.8717109521665329375, 1.000000000000000000),
 ( 0.8974258578414069376, 0.8783573442015528698, 1.000000000000000000),
 ( 0.8972948393364401642, 0.8782019693812764816, 1.000000000000000000) ) ) 
 REPRESENTATION_ITEM ( '' )  SURFACE ( )  );
#39125=FACE_OUTER_BOUND ( 'NONE', #36184, .T. ) ;
#39137=DIRECTION ( 'NONE',  ( -0.000000000000000000, -0.000000000000000000, -1.000000000000000000 ) ) ;
#39144=B_SPLINE_CURVE_WITH_KNOTS ( 'NONE', 3,
 ( #90645, #10667, #25807, #54687, #83561, #84042, #40456, #10196 ),
 .UNSPECIFIED., .F., .F.,
 ( 4, 2, 2, 4 ),
 ( 5.346692419836454808E-16, 0.001939204242612728663, 0.002908806363918823353, 0.003878408485224918260 ),
 .UNSPECIFIED. ) ;
#39147=CARTESIAN_POINT ( 'NONE',  ( 183.0442525570908288, 264.6571197653884155, -7.500000000000000000 ) ) ;
#39148=CARTESIAN_POINT ( 'NONE',  ( 154.1270911980395226, 19.37729811922127610, -12.09914501918770924 ) ) ;
#39166=CARTESIAN_POINT ( 'NONE',  ( 140.6539576904058606, 250.5000000000000568, -10.49999999999999822 ) ) ;
#39169=CARTESIAN_POINT ( 'NONE',  ( 153.9755810662746569, 128.3195885613610869, 13.16651113973756715 ) ) ;
#39170=AXIS2_PLACEMENT_3D ( 'NONE', #17235, #44701, #80690 ) ;
#39182=VERTEX_POINT ( 'NONE', #86981 ) ;
#39183=DIRECTION ( 'NONE',  ( 2.220446049250312686E-15, 0.000000000000000000, 1.000000000000000000 ) ) ;
#39197=CARTESIAN_POINT ( 'NONE',  ( 156.4851178187871312, 69.18068689461284748, -7.000000000000000888 ) ) ;
#39198=CARTESIAN_POINT ( 'NONE',  ( 154.5739546116916472, 19.95362051968762529, -14.09237539257703276 ) ) ;
#39209=FACE_OUTER_BOUND ( 'NONE', #15781, .T. ) ;
#39211=CARTESIAN_POINT ( 'NONE',  ( 195.2403266774578583, 20.74618149458048677, 13.25394924001932395 ) ) ;
#39220=DIRECTION ( 'NONE',  ( -0.2156506209390900430, 0.000000000000000000, -0.9764705882352960886 ) ) ;
#39229=AXIS2_PLACEMENT_3D ( 'NONE', #22368, #88144, #51698 ) ;
#39232=VERTEX_POINT ( 'NONE', #85591 ) ;
#39233=CARTESIAN_POINT ( 'NONE',  ( 197.7335303680046650, 24.96166607582781083, 12.00000000000000000 ) ) ;
#39235=CARTESIAN_POINT ( 'NONE',  ( 175.2296996224750103, 149.6461846693799487, -24.00000000000001066 ) ) ;
#39251=CARTESIAN_POINT ( 'NONE',  ( 156.9186793294233837, 275.7877658745666167, 16.89624193776998595 ) ) ;
#39254=FACE_OUTER_BOUND ( 'NONE', #52663, .T. ) ;
#39255=CARTESIAN_POINT ( 'NONE',  ( 195.6468468325649326, 26.28259184625311207, 14.75238424381223723 ) ) ;
#39269=SHAPE_DEFINITION_REPRESENTATION ( #59426, #80896 ) ;
#39274=FACE_OUTER_BOUND ( 'NONE', #49551, .T. ) ;
#39279=CARTESIAN_POINT ( 'NONE',  ( 196.7383257810085695, 24.47698789593440694, 10.99999999999999112 ) ) ;
#39300=DIRECTION ( 'NONE',  ( 0.000000000000000000, 1.000000000000000000, 0.000000000000000000 ) ) ;
#39302=CIRCLE ( 'NONE', #4589, 24.00000000000001066 ) ;
#39313=B_SPLINE_CURVE_WITH_KNOTS ( 'NONE', 3,
 ( #32695, #48276, #12308, #34101 ),
 .UNSPECIFIED., .F., .F.,
 ( 4, 4 ),
 ( 6.973502068242161363E-17, 0.001032852107770819081 ),
 .UNSPECIFIED. ) ;
#39314=CARTESIAN_POINT ( 'NONE',  ( 209.3503997127169214, 0.03340139000135424613, 7.446935725088736469 ) ) ;
#39336=EDGE_LOOP ( 'NONE', ( #84928, #37732, #50799, #8347 ) ) ;
#39340=DIRECTION ( 'NONE',  ( -0.7981962569173468580, -5.551115123125764401E-14, 0.6023974895724060197 ) ) ;
#39351=FACE_BOUND ( 'NONE', #3795, .T. ) ;
#39356=CARTESIAN_POINT ( 'NONE',  ( 193.6552470326849402, 275.0000000000000568, 16.89672165344822119 ) ) ;
#39374=ORIENTED_EDGE ( 'NONE', *, *, #66535, .F. ) ;
#39378=EDGE_CURVE ( 'NONE', #76413, #90266, #91342, .T. ) ;
#39381=CARTESIAN_POINT ( 'NONE',  ( 194.7453183674699915, 19.99999999999999645, -15.62499999999999112 ) ) ;
#39404=VERTEX_POINT ( 'NONE', #7004 ) ;
#39405=CARTESIAN_POINT ( 'NONE',  ( 212.4629471475955427, 32.98517505407394168, 13.08022668053247095 ) ) ;
#39409=ORIENTED_EDGE ( 'NONE', *, *, #49120, .F. ) ;
#39425=FACE_OUTER_BOUND ( 'NONE', #6035, .T. ) ;
#39432=FACE_OUTER_BOUND ( 'NONE', #88048, .T. ) ;
#39435=CARTESIAN_POINT ( 'NONE',  ( 219.8344101925596021, 35.72494958537217968, -7.000000000000000000 ) ) ;
#39437=CARTESIAN_POINT ( 'NONE',  ( 158.9078607026157499, 16.88031981475993959, -10.36078569760457491 ) ) ;
#39439=CARTESIAN_POINT ( 'NONE',  ( 140.6539576904058606, 275.5000000000000568, -12.50000000000000000 ) ) ;
#39452=EDGE_LOOP ( 'NONE', ( #25431, #60983, #64404, #4012 ) ) ;
#39457=ORIENTED_EDGE ( 'NONE', *, *, #25669, .F. ) ;
#39459=DIRECTION ( 'NONE',  ( 0.9998346970812741485, 0.000000000000000000, -0.01818181818182024179 ) ) ;
#39485=EDGE_CURVE ( 'NONE', #48324, #68290, #83801, .T. ) ;
#39488=ORIENTED_EDGE ( 'NONE', *, *, #67721, .T. ) ;
#39499=AXIS2_PLACEMENT_3D ( 'NONE', #52891, #24017, #16920 ) ;
#39516=CARTESIAN_POINT ( 'NONE',  ( 196.1347706148621057, 72.64529849370360637, -11.79135490535123942 ) ) ;
#39522=CARTESIAN_POINT ( 'NONE',  ( 205.7786681169002350, 32.98517505407394168, 10.00000000000000000 ) ) ;
#39530=CARTESIAN_POINT ( 'NONE',  ( 153.8045584215660710, 20.39561363287349849, -12.88435682625986267 ) ) ;
#39537=ADVANCED_FACE ( 'NONE', ( #63854 ), #42976, .F. ) ;
#39554=AXIS2_PLACEMENT_3D ( 'NONE', #14543, #86946, #43850 ) ;
#39566=VECTOR ( 'NONE', #35414, 1000.000000000000000 ) ;
#39578=ORIENTED_EDGE ( 'NONE', *, *, #12627, .F. ) ;
#39579=CARTESIAN_POINT ( 'NONE',  ( 198.0538618622170191, 70.37887259939165574, 10.53035661854988270 ) ) ;
#39581=CARTESIAN_POINT ( 'NONE',  ( 175.2296996224750103, 275.0000000000000568, 24.00000000000000355 ) ) ;
#39601=EDGE_CURVE ( 'NONE', #77887, #1585, #49608, .T. ) ;
#39617=EDGE_CURVE ( 'NONE', #13346, #78803, #67202, .T. ) ;
#39618=ORIENTED_EDGE ( 'NONE', *, *, #88318, .T. ) ;
#39626=CARTESIAN_POINT ( 'NONE',  ( 180.4306473129080359, 214.7033776542919270, -24.48382199637807943 ) ) ;
#39627=CIRCLE ( 'NONE', #59343, 24.50000000000000355 ) ;
#39629=AXIS2_PLACEMENT_3D ( 'NONE', #83605, #9845, #1349 ) ;
#39638=CARTESIAN_POINT ( 'NONE',  ( 194.2870706637141325, 39.56299966811847924, 14.58823529411763431 ) ) ;
#39642=CARTESIAN_POINT ( 'NONE',  ( 196.8865788344785699, 19.32388290151978438, 12.43054049968610997 ) ) ;
#39670=( BOUNDED_CURVE ( )  B_SPLINE_CURVE ( 3, ( #9281, #81264, #44810, #30155 ),
 .UNSPECIFIED., .F., .F. ) 
 B_SPLINE_CURVE_WITH_KNOTS ( ( 4, 4 ),
 ( 4.712388980384688786, 5.759586531581284419 ),
 .UNSPECIFIED. ) 
 CURVE ( )  GEOMETRIC_REPRESENTATION_ITEM ( )  RATIONAL_B_SPLINE_CURVE ( ( 1.000000000000000000, 0.9106836025229594345, 0.9106836025229594345, 1.000000000000000000 ) ) 
 REPRESENTATION_ITEM ( '' )  );
#39671=FACE_OUTER_BOUND ( 'NONE', #1068, .T. ) ;
#39673=EDGE_CURVE ( 'NONE', #26249, #76130, #72783, .T. ) ;
#39674=DIRECTION ( 'NONE',  ( 0.000000000000000000, -1.000000000000000000, 0.000000000000000000 ) ) ;
#39692=ORIENTED_EDGE ( 'NONE', *, *, #55527, .F. ) ;
#39693=LINE ( 'NONE', #69541, #49867 ) ;
#39694=AXIS2_PLACEMENT_3D ( 'NONE', #6491, #84601, #21153 ) ;
#39696=CARTESIAN_POINT ( 'NONE',  ( 140.6539576904058606, 249.5000000000000568, 12.50000000000000000 ) ) ;
#39702=AXIS2_PLACEMENT_3D ( 'NONE', #65376, #488, #43561 ) ;
#39717=CARTESIAN_POINT ( 'NONE',  ( 170.2297021224755724, 215.0000000000000568, -25.00499999999998835 ) ) ;
#39718=CARTESIAN_POINT ( 'NONE',  ( 175.2296996224750103, 249.5000000000000568, 0.000000000000000000 ) ) ;
#39726=VERTEX_POINT ( 'NONE', #92687 ) ;
#39735=ORIENTED_EDGE ( 'NONE', *, *, #62500, .T. ) ;
#39737=DIRECTION ( 'NONE',  ( 0.000000000000000000, 0.000000000000000000, 1.000000000000000000 ) ) ;
#39742=FACE_OUTER_BOUND ( 'NONE', #42578, .T. ) ;
#39754=CARTESIAN_POINT ( 'NONE',  ( 194.1581894022642416, 20.00000000000000000, -14.79860320208535107 ) ) ;
#39756=CIRCLE ( 'NONE', #36749, 0.9999999999999977796 ) ;
#39759=EDGE_CURVE ( 'NONE', #84950, #13726, #78504, .T. ) ;
#39763=CIRCLE ( 'NONE', #59479, 5.568361562975243650 ) ;
#39765=PLANE ( 'NONE',  #5160 ) ;
#39766=AXIS2_PLACEMENT_3D ( 'NONE', #2419, #30357, #17078 ) ;
#39777=AXIS2_PLACEMENT_3D ( 'NONE', #76852, #11978, #63143 ) ;
#39778=ADVANCED_FACE ( 'NONE', ( #1739 ), #87434, .T. ) ;
#39779=DIRECTION ( 'NONE',  ( 0.000000000000000000, 0.000000000000000000, -1.000000000000000000 ) ) ;
#39781=DIRECTION ( 'NONE',  ( -0.000000000000000000, 1.000000000000000000, -0.000000000000000000 ) ) ;
#39784=VECTOR ( 'NONE', #52031, 1000.000000000000000 ) ;
#39789=CARTESIAN_POINT ( 'NONE',  ( 201.2104617360081704, 41.21457449016151031, 10.00000000000000000 ) ) ;
#39791=VECTOR ( 'NONE', #10834, 1000.000000000000000 ) ;
#39792=CARTESIAN_POINT ( 'NONE',  ( 155.7140808774800007, 21.00000000000000000, 15.62500000000000000 ) ) ;
#39794=CARTESIAN_POINT ( 'NONE',  ( 201.0592549708492243, 40.73798607845792930, 9.999999999999998224 ) ) ;
#39805=ORIENTED_EDGE ( 'NONE', *, *, #55943, .F. ) ;
#39806=DIRECTION ( 'NONE',  ( -1.000000000000000000, -0.000000000000000000, 0.000000000000000000 ) ) ;
#39809=DIRECTION ( 'NONE',  ( 0.9531768234071978929, -0.3024135303179465439, -0.000000000000000000 ) ) ;
#39821=CARTESIAN_POINT ( 'NONE',  ( 156.1688672180385709, 17.06233518523205106, 10.31625060074216726 ) ) ;
#39822=CARTESIAN_POINT ( 'NONE',  ( 152.6878475589607262, 19.85941866395974031, -8.897000670449973114 ) ) ;
#39831=AXIS2_PLACEMENT_3D ( 'NONE', #51802, #15371, #74519 ) ;
#39837=EDGE_LOOP ( 'NONE', ( #36526, #92299, #64421, #82263 ) ) ;
#39841=CIRCLE ( 'NONE', #92800, 0.5000000000000004441 ) ;
#39851=VERTEX_POINT ( 'NONE', #45270 ) ;
#39854=CIRCLE ( 'NONE', #18733, 3.842139515347647638 ) ;
#39859=DIRECTION ( 'NONE',  ( 1.000000000000000000, 0.000000000000000000, 0.000000000000000000 ) ) ;
#39868=VECTOR ( 'NONE', #51027, 1000.000000000000114 ) ;
#39873=DIRECTION ( 'NONE',  ( -0.000000000000000000, -0.000000000000000000, -1.000000000000000000 ) ) ;
#39877=ORIENTED_EDGE ( 'NONE', *, *, #67912, .T. ) ;
#39885=DIRECTION ( 'NONE',  ( -0.000000000000000000, -0.000000000000000000, -1.000000000000000000 ) ) ;
#39896=LINE ( 'NONE', #38519, #26120 ) ;
#39899=EDGE_CURVE ( 'NONE', #26691, #6854, #16880, .T. ) ;
#39902=DIRECTION ( 'NONE',  ( -1.000000000000000000, 0.000000000000000000, 0.000000000000000000 ) ) ;
#39903=CARTESIAN_POINT ( 'NONE',  ( 195.4602890156073443, 20.04204674317102430, 14.69963036182647720 ) ) ;
#39905=AXIS2_PLACEMENT_3D ( 'NONE', #5468, #6395, #34800 ) ;
#39907=CARTESIAN_POINT ( 'NONE',  ( 152.4536156746142410, 275.0000000000000568, 11.50000000000000000 ) ) ;
#39910=CARTESIAN_POINT ( 'NONE',  ( 208.6643680990008534, 36.42852971205770984, 14.80559097128779911 ) ) ;
#39912=DIRECTION ( 'NONE',  ( 0.000000000000000000, 0.000000000000000000, 1.000000000000000000 ) ) ;
#39915=CARTESIAN_POINT ( 'NONE',  ( 157.0248177074734315, 17.42562647115670060, -9.460300111311761739 ) ) ;
#39927=AXIS2_PLACEMENT_3D ( 'NONE', #88580, #39300, #10899 ) ;
#39934=DIRECTION ( 'NONE',  ( -0.000000000000000000, -0.000000000000000000, -1.000000000000000000 ) ) ;
#39950=CARTESIAN_POINT ( 'NONE',  ( 185.2169494693457921, 250.5000000000000568, 22.91843887563416615 ) ) ;
#39963=ORIENTED_EDGE ( 'NONE', *, *, #56745, .F. ) ;
#39972=B_SPLINE_CURVE_WITH_KNOTS ( 'NONE', 3,
 ( #55103, #55578, #20043, #19118, #5397, #84426, #34262, #63169 ),
 .UNSPECIFIED., .F., .F.,
 ( 4, 2, 2, 4 ),
 ( 0.000000000000000000, 0.0009268394340039834076, 0.001390259151005943669, 0.001853678868007904148 ),
 .UNSPECIFIED. ) ;
#40012=CARTESIAN_POINT ( 'NONE',  ( 153.4730978675979998, 20.31600801108083587, 12.31661104704794951 ) ) ;
#40020=EDGE_CURVE ( 'NONE', #6020, #6460, #54951, .T. ) ;
#40031=EDGE_CURVE ( 'NONE', #4210, #16726, #23526, .T. ) ;
#40044=DIRECTION ( 'NONE',  ( 0.000000000000000000, 0.000000000000000000, -1.000000000000000000 ) ) ;
#40054=CIRCLE ( 'NONE', #68819, 4.999999999999990230 ) ;
#40070=AXIS2_PLACEMENT_3D ( 'NONE', #11248, #9840, #90294 ) ;
#40072=ORIENTED_EDGE ( 'NONE', *, *, #10248, .F. ) ;
#40073=CARTESIAN_POINT ( 'NONE',  ( 175.2296996224749250, 275.5000000000000568, -29.99999999999998224 ) ) ;
#40082=CARTESIAN_POINT ( 'NONE',  ( 195.0629117428269126, 293.9636489450776367, -54.00000000000000000 ) ) ;
#40083=CARTESIAN_POINT ( 'NONE',  ( 154.5815831708048336, 19.45636901171593180, -12.71858327454078363 ) ) ;
#40087=ORIENTED_EDGE ( 'NONE', *, *, #18823, .T. ) ;
#40097=VERTEX_POINT ( 'NONE', #38173 ) ;
#40102=CARTESIAN_POINT ( 'NONE',  ( 185.3457823239910738, 214.6360786829742437, 22.87680765314584264 ) ) ;
#40104=CARTESIAN_POINT ( 'NONE',  ( 150.7108941768076420, 20.99999999999999645, 5.100416763304269629 ) ) ;
#40105=EDGE_CURVE ( 'NONE', #87677, #83522, #1280, .T. ) ;
#40116=ORIENTED_EDGE ( 'NONE', *, *, #46756, .T. ) ;
#40117=ORIENTED_EDGE ( 'NONE', *, *, #60551, .F. ) ;
#40135=AXIS2_PLACEMENT_3D ( 'NONE', #784, #21614, #51411 ) ;
#40146=CARTESIAN_POINT ( 'NONE',  ( 152.4536156746142410, 275.0000000000000568, -14.50000000000000000 ) ) ;
#40148=DIRECTION ( 'NONE',  ( -0.000000000000000000, -1.000000000000000000, -0.000000000000000000 ) ) ;
#40154=DIRECTION ( 'NONE',  ( 0.000000000000000000, 1.000000000000000000, 0.000000000000000000 ) ) ;
#40157=CARTESIAN_POINT ( 'NONE',  ( 207.1738322328983770, 30.51833626076158978, 15.03205023725369038 ) ) ;
#40164=B_SPLINE_CURVE_WITH_KNOTS ( 'NONE', 3,
 ( #60924, #82216, #9298, #67561 ),
 .UNSPECIFIED., .F., .F.,
 ( 4, 4 ),
 ( 0.000000000000000000, 9.632970524405273739E-05 ),
 .UNSPECIFIED. ) ;
#40189=CARTESIAN_POINT ( 'NONE',  ( 196.3765075725969211, 25.23352658328733256, 13.80344107416052957 ) ) ;
#40192=ADVANCED_FACE ( 'NONE', ( #23046 ), #58594, .T. ) ;
#40199=AXIS2_PLACEMENT_3D ( 'NONE', #37305, #29292, #80864 ) ;
#40209=ORIENTED_EDGE ( 'NONE', *, *, #49529, .F. ) ;
#40210=DIRECTION ( 'NONE',  ( -0.6249999999999938938, -1.354168079406255383E-15, 0.7806247497998046736 ) ) ;
#40215=CARTESIAN_POINT ( 'NONE',  ( 184.1778392089217107, 3.000000000000000888, 9.000000000000001776 ) ) ;
#40226=CARTESIAN_POINT ( 'NONE',  ( 200.9103445561495960, 65.54396272403066348, 5.212391550061751921 ) ) ;
#40228=( BOUNDED_CURVE ( )  B_SPLINE_CURVE ( 3, ( #93044, #28201, #16303, #15848 ),
 .UNSPECIFIED., .F., .F. ) 
 B_SPLINE_CURVE_WITH_KNOTS ( ( 4, 4 ),
 ( 4.278565243615663150, 4.712388980384691450 ),
 .UNSPECIFIED. ) 
 CURVE ( )  GEOMETRIC_REPRESENTATION_ITEM ( )  RATIONAL_B_SPLINE_CURVE ( ( 1.000000000000000000, 0.9843778111405747655, 0.9843778111405747655, 1.000000000000000000 ) ) 
 REPRESENTATION_ITEM ( '' )  );
#40235=DIRECTION ( 'NONE',  ( 0.000000000000000000, 0.000000000000000000, 1.000000000000000000 ) ) ;
#40247=CARTESIAN_POINT ( 'NONE',  ( 197.9445473535685380, 71.72765703694831529, 10.67027600767679019 ) ) ;
#40249=CARTESIAN_POINT ( 'NONE',  ( 189.9243309297870610, 275.5000000000000568, 20.22542485937349355 ) ) ;
#40257=CARTESIAN_POINT ( 'NONE',  ( 154.7659666677267580, 19.56018909072085066, 12.94946946941272437 ) ) ;
#40259=DIRECTION ( 'NONE',  ( 0.000000000000000000, 1.000000000000000000, 0.000000000000000000 ) ) ;
#40261=CARTESIAN_POINT ( 'NONE',  ( 186.6539576904058890, 293.9636489450775230, 0.000000000000000000 ) ) ;
#40272=ORIENTED_EDGE ( 'NONE', *, *, #4411, .F. ) ;
#40273=CARTESIAN_POINT ( 'NONE',  ( 208.6208076322478746, 32.98517505407394168, 10.00000000000000000 ) ) ;
#40287=FACE_OUTER_BOUND ( 'NONE', #41324, .T. ) ;
#40288=EDGE_CURVE ( 'NONE', #85305, #55107, #44337, .T. ) ;
#40289=CARTESIAN_POINT ( 'NONE',  ( 185.4863495377425977, 214.7658868572315498, 22.87680765314782860 ) ) ;
#40296=ADVANCED_FACE ( 'NONE', ( #46214 ), #88831, .T. ) ;
#40304=ORIENTED_EDGE ( 'NONE', *, *, #42665, .T. ) ;
#40306=ORIENTED_EDGE ( 'NONE', *, *, #28382, .F. ) ;
#40311=CARTESIAN_POINT ( 'NONE',  ( 193.9646936176702070, 19.99999999999999645, -14.99999999999999467 ) ) ;
#40323=LINE ( 'NONE', #25214, #58155 ) ;
#40328=ORIENTED_EDGE ( 'NONE', *, *, #7928, .T. ) ;
#40335=ORIENTED_EDGE ( 'NONE', *, *, #25145, .T. ) ;
#40346=CARTESIAN_POINT ( 'NONE',  ( 197.4878715644970555, 25.93102243561465414, 12.00000000000000000 ) ) ;
#40351=CARTESIAN_POINT ( 'NONE',  ( 209.3190042249899250, 30.23012903947021002, 15.12480380540110225 ) ) ;
#40361=CARTESIAN_POINT ( 'NONE',  ( 208.6208076322478746, 32.98517505407394168, 10.50000000000000000 ) ) ;
#40365=DIRECTION ( 'NONE',  ( 0.000000000000000000, 0.000000000000000000, -1.000000000000000000 ) ) ;
#40367=EDGE_LOOP ( 'NONE', ( #4252, #12887, #11919, #7860 ) ) ;
#40368=CARTESIAN_POINT ( 'NONE',  ( 159.2635086430405806, 16.19322481500868705, -10.13850573484308804 ) ) ;
#40370=CARTESIAN_POINT ( 'NONE',  ( 155.0193446949349152, 20.65816215000725720, 12.95286603764679256 ) ) ;
#40382=ORIENTED_EDGE ( 'NONE', *, *, #56881, .F. ) ;
#40385=DIRECTION ( 'NONE',  ( -0.000000000000000000, -1.000000000000000000, -0.000000000000000000 ) ) ;
#40387=EDGE_LOOP ( 'NONE', ( #76359, #71253, #83430, #35479 ) ) ;
#40389=DIRECTION ( 'NONE',  ( 0.000000000000000000, 1.000000000000000000, 0.000000000000000000 ) ) ;
#40401=EDGE_CURVE ( 'NONE', #79261, #4223, #89676, .T. ) ;
#40404=DIRECTION ( 'NONE',  ( -0.000000000000000000, 0.000000000000000000, -1.000000000000000000 ) ) ;
#40417=ORIENTED_EDGE ( 'NONE', *, *, #79684, .F. ) ;
#40437=ORIENTED_EDGE ( 'NONE', *, *, #45647, .F. ) ;
#40443=ORIENTED_EDGE ( 'NONE', *, *, #53476, .F. ) ;
#40445=VERTEX_POINT ( 'NONE', #73267 ) ;
#40456=CARTESIAN_POINT ( 'NONE',  ( 194.9499353771399512, 21.00000000000000711, -15.36943343683466168 ) ) ;
#40470=CARTESIAN_POINT ( 'NONE',  ( 196.0143093133015384, 73.40565171261611965, 12.00000000000000888 ) ) ;
#40478=( NAMED_UNIT ( * ) SI_UNIT ( $, .STERADIAN. ) SOLID_ANGLE_UNIT ( ) );
#40479=FACE_OUTER_BOUND ( 'NONE', #67946, .T. ) ;
#40483=EDGE_CURVE ( 'NONE', #68325, #33225, #29218, .T. ) ;
#40485=CARTESIAN_POINT ( 'NONE',  ( 152.0194914954574870, 20.99319818809533089, -6.266237208439005890 ) ) ;
#40494=DIRECTION ( 'NONE',  ( -1.000000000000000000, 0.000000000000000000, 0.000000000000000000 ) ) ;
#40498=CARTESIAN_POINT ( 'NONE',  ( 195.8725848201698341, 20.33787691583836121, -12.24547402278110475 ) ) ;
#40512=AXIS2_PLACEMENT_3D ( 'NONE', #12870, #4801, #78192 ) ;
#40517=CARTESIAN_POINT ( 'NONE',  ( 175.2296996224750103, 275.5000000000000568, 0.000000000000000000 ) ) ;
#40529=ORIENTED_EDGE ( 'NONE', *, *, #84969, .T. ) ;
#40540=DIRECTION ( 'NONE',  ( 0.000000000000000000, 0.000000000000000000, 1.000000000000000000 ) ) ;
#40545=ORIENTED_EDGE ( 'NONE', *, *, #93286, .F. ) ;
#40555=VERTEX_POINT ( 'NONE', #68008 ) ;
#40560=CARTESIAN_POINT ( 'NONE',  ( 185.2169494693457921, 214.5000000000000568, 22.91843887563416615 ) ) ;
#40562=EDGE_CURVE ( 'NONE', #2640, #11817, #24924, .T. ) ;
#40563=DIRECTION ( 'NONE',  ( 0.000000000000000000, 1.000000000000000000, 0.000000000000000000 ) ) ;
#40564=CARTESIAN_POINT ( 'NONE',  ( 197.0359635097987336, 71.72764050496320465, 10.24344765925977185 ) ) ;
#40571=CARTESIAN_POINT ( 'NONE',  ( 165.2494399300530290, 8.542400036368780647, 9.000000000000001776 ) ) ;
#40573=CARTESIAN_POINT ( 'NONE',  ( 194.7497628521415152, 41.36675632506837985, 13.96383658842646014 ) ) ;
#40575=ORIENTED_EDGE ( 'NONE', *, *, #49238, .F. ) ;
#40576=ORIENTED_EDGE ( 'NONE', *, *, #53799, .T. ) ;
#40577=CARTESIAN_POINT ( 'NONE',  ( 200.1633050441426747, 15.87263057655181520, 10.05743975622734787 ) ) ;
#40584=CIRCLE ( 'NONE', #20957, 25.00000000000000355 ) ;
#40593=CARTESIAN_POINT ( 'NONE',  ( 195.5719271795211682, 40.32756825300102577, 13.76475510248965684 ) ) ;
#40615=CARTESIAN_POINT ( 'NONE',  ( 195.8990914565195567, 41.11444846156542354, 14.40741235656477848 ) ) ;
#40624=VERTEX_POINT ( 'NONE', #65352 ) ;
#40625=FACE_OUTER_BOUND ( 'NONE', #64878, .T. ) ;
#40636=ORIENTED_EDGE ( 'NONE', *, *, #47942, .T. ) ;
#40640=CARTESIAN_POINT ( 'NONE',  ( 197.5461146820061060, 68.31320778629316237, -9.184551779179372488 ) ) ;
#40643=ORIENTED_EDGE ( 'NONE', *, *, #4507, .F. ) ;
#40646=CIRCLE ( 'NONE', #5897, 25.00000000000000355 ) ;
#40648=FACE_OUTER_BOUND ( 'NONE', #20665, .T. ) ;
#40658=EDGE_LOOP ( 'NONE', ( #93690, #70994, #37524, #38730 ) ) ;
#40670=CARTESIAN_POINT ( 'NONE',  ( 179.1465552314772083, 8.542400036368780647, 9.000000000000001776 ) ) ;
#40675=CARTESIAN_POINT ( 'NONE',  ( 200.5254236182467764, 215.0000000000001705, -2.961736701814141171 ) ) ;
#40685=EDGE_LOOP ( 'NONE', ( #91567, #82011, #82294, #69445 ) ) ;
#40686=CARTESIAN_POINT ( 'NONE',  ( 180.5131398354828320, 276.0000000000000568, -23.92352941176473635 ) ) ;
#40708=CARTESIAN_POINT ( 'NONE',  ( 196.8409580319986674, 73.46773880466290052, 12.56795567929779622 ) ) ;
#40710=VECTOR ( 'NONE', #64231, 1000.000000000000000 ) ;
#40711=DIRECTION ( 'NONE',  ( 0.000000000000000000, 1.000000000000000000, 0.000000000000000000 ) ) ;
#40719=ADVANCED_FACE ( 'NONE', ( #64436 ), #24675, .T. ) ;
#40721=EDGE_CURVE ( 'NONE', #53411, #14181, #41284, .T. ) ;
#40722=CARTESIAN_POINT ( 'NONE',  ( 156.1760182705776288, 20.00000000000000000, 14.66829968254666738 ) ) ;
#40724=CARTESIAN_POINT ( 'NONE',  ( 202.1676623822758359, 287.7243935111420683, -5.007149546673600682 ) ) ;
#40735=ORIENTED_EDGE ( 'NONE', *, *, #59920, .F. ) ;
#40739=DIRECTION ( 'NONE',  ( 0.2456588035076220367, -0.9693563597868450898, 0.000000000000000000 ) ) ;
#40773=DIRECTION ( 'NONE',  ( 0.000000000000000000, 0.000000000000000000, 1.000000000000000000 ) ) ;
#40777=ORIENTED_EDGE ( 'NONE', *, *, #69768, .T. ) ;
#40791=ORIENTED_EDGE ( 'NONE', *, *, #29697, .F. ) ;
#40798=ORIENTED_EDGE ( 'NONE', *, *, #13973, .T. ) ;
#40799=CARTESIAN_POINT ( 'NONE',  ( 164.2231345125756263, 296.7472757692770529, -7.499999999999996447 ) ) ;
#40810=CARTESIAN_POINT ( 'NONE',  ( 175.2296996224749250, 215.0000000000000568, -24.99999999999999289 ) ) ;
#40815=CARTESIAN_POINT ( 'NONE',  ( 208.8036087770903748, 29.39224792112960927, 14.71645718445160966 ) ) ;
#40825=CARTESIAN_POINT ( 'NONE',  ( 187.8995604928813918, 43.86402690510830382, 12.00000000000000000 ) ) ;
#40826=DIRECTION ( 'NONE',  ( -0.2456588035076248677, 0.9693563597868444237, 0.000000000000000000 ) ) ;
#40830=ADVANCED_FACE ( 'NONE', ( #72435 ), #14221, .F. ) ;
#40833=ORIENTED_EDGE ( 'NONE', *, *, #17917, .F. ) ;
#40836=CARTESIAN_POINT ( 'NONE',  ( 154.7659666677267865, 20.47222690886501439, 12.53936336329526391 ) ) ;
#40849=CIRCLE ( 'NONE', #21218, 0.5000000000000004441 ) ;
#40852=AXIS2_PLACEMENT_3D ( 'NONE', #90572, #40385, #62207 ) ;
#40854=DIRECTION ( 'NONE',  ( 0.9693563597868444237, 0.2456588035076248677, -0.000000000000000000 ) ) ;
#40856=ORIENTED_EDGE ( 'NONE', *, *, #38609, .T. ) ;
#40872=LINE ( 'NONE', #76895, #33371 ) ;
#40906=ORIENTED_EDGE ( 'NONE', *, *, #34635, .F. ) ;
#40912=ORIENTED_EDGE ( 'NONE', *, *, #71404, .T. ) ;
#40914=ORIENTED_EDGE ( 'NONE', *, *, #41255, .T. ) ;
#40918=CIRCLE ( 'NONE', #56109, 7.999911143031724237 ) ;
#40922=CARTESIAN_POINT ( 'NONE',  ( 153.6987871352711466, 19.48326534539917887, -11.45812909362559928 ) ) ;
#40927=DIRECTION ( 'NONE',  ( 0.000000000000000000, 0.000000000000000000, 1.000000000000000000 ) ) ;
#40929=EDGE_CURVE ( 'NONE', #35152, #81908, #51903, .T. ) ;
#40935=CARTESIAN_POINT ( 'NONE',  ( 152.4536156746142410, 276.0000000000000568, 14.50000000000000000 ) ) ;
#40946=( NAMED_UNIT ( * ) PLANE_ANGLE_UNIT ( ) SI_UNIT ( $, .RADIAN. ) );
#40950=ADVANCED_FACE ( 'NONE', ( #71035 ), #13181, .F. ) ;
#40960=CARTESIAN_POINT ( 'NONE',  ( 164.6329196456214277, 275.0000000000000568, 23.09031830825856701 ) ) ;
#40961=CARTESIAN_POINT ( 'NONE',  ( 208.3303265509962330, 36.67066202700165434, 13.52119360038354401 ) ) ;
#40964=CARTESIAN_POINT ( 'NONE',  ( 183.0442525570908288, 300.2961574867697436, -7.500000000000000000 ) ) ;
#40982=CARTESIAN_POINT ( 'NONE',  ( 204.6539576904058606, 300.0210572133868823, -5.225551010890672643 ) ) ;
#40983=TOROIDAL_SURFACE ( 'NONE', #31964, 3.342139515347635204, 0.5000000000000000000 ) ;
#41002=DIRECTION ( 'NONE',  ( 0.000000000000000000, 1.000000000000000000, 0.000000000000000000 ) ) ;
#41003=DIRECTION ( 'NONE',  ( 1.000000000000000000, -0.000000000000000000, -0.000000000000000000 ) ) ;
#41007=ORIENTED_EDGE ( 'NONE', *, *, #5504, .T. ) ;
#41021=PLANE ( 'NONE',  #8391 ) ;
#41032=FACE_OUTER_BOUND ( 'NONE', #68034, .T. ) ;
#41036=CARTESIAN_POINT ( 'NONE',  ( 196.2760846862221058, 19.11198087481172081, 12.12215979492540896 ) ) ;
#41040=EDGE_CURVE ( 'NONE', #13153, #6020, #32245, .T. ) ;
#41046=AXIS2_PLACEMENT_3D ( 'NONE', #71142, #11497, #26644 ) ;
#41050=AXIS2_PLACEMENT_3D ( 'NONE', #14805, #78274, #41792 ) ;
#41053=DIRECTION ( 'NONE',  ( 0.000000000000000000, 0.000000000000000000, -1.000000000000000000 ) ) ;
#41054=CARTESIAN_POINT ( 'NONE',  ( 154.1415209985679269, 20.37991841447901464, 11.45812909362557441 ) ) ;
#41056=CIRCLE ( 'NONE', #7835, 2.842139515347646750 ) ;
#41068=DIRECTION ( 'NONE',  ( 0.000000000000000000, 0.000000000000000000, -1.000000000000000000 ) ) ;
#41078=CARTESIAN_POINT ( 'NONE',  ( 157.7277585059063938, 1.242640687119286103, -10.00000000000000355 ) ) ;
#41081=CARTESIAN_POINT ( 'NONE',  ( 195.5826719941578347, 41.40013651751736745, 14.51828210624160675 ) ) ;
#41089=CARTESIAN_POINT ( 'NONE',  ( 153.1687287787850948, 19.71439303874801752, 10.22517819559350727 ) ) ;
#41091=CARTESIAN_POINT ( 'NONE',  ( 189.9243309297870610, 275.0000000000000568, 15.22542485937351664 ) ) ;
#41112=CIRCLE ( 'NONE', #50270, 24.50000000000000000 ) ;
#41113=DIRECTION ( 'NONE',  ( 0.000000000000000000, 1.000000000000000000, 0.000000000000000000 ) ) ;
#41114=CARTESIAN_POINT ( 'NONE',  ( 0.000000000000000000, 0.000000000000000000, -9.000000000000001776 ) ) ;
#41115=CARTESIAN_POINT ( 'NONE',  ( 195.4637550158223576, 27.11842685737634184, 15.00000000000008704 ) ) ;
#41136=VERTEX_POINT ( 'NONE', #9872 ) ;
#41137=CARTESIAN_POINT ( 'NONE',  ( 156.4947056272797852, 21.00000000000000000, -15.00000000000000000 ) ) ;
#41151=VERTEX_POINT ( 'NONE', #87532 ) ;
#41152=DIRECTION ( 'NONE',  ( 0.000000000000000000, -1.000000000000000000, 0.000000000000000000 ) ) ;
#41160=CARTESIAN_POINT ( 'NONE',  ( 202.8019728163925492, 61.40723988820079171, -7.000000000000000888 ) ) ;
#41179=VECTOR ( 'NONE', #51072, 1000.000000000000000 ) ;
#41187=AXIS2_PLACEMENT_3D ( 'NONE', #30126, #8341, #37223 ) ;
#41191=ADVANCED_FACE ( 'NONE', ( #37808 ), #60550, .T. ) ;
#41192=CARTESIAN_POINT ( 'NONE',  ( 160.5350683151633291, 275.5000000000000568, 20.22542485937379908 ) ) ;
#41219=CYLINDRICAL_SURFACE ( 'NONE', #49024, 24.99999999999999645 ) ;
#41234=EDGE_LOOP ( 'NONE', ( #54153, #22267, #58546, #87067 ) ) ;
#41246=CIRCLE ( 'NONE', #474, 4.000000000000003553 ) ;
#41249=AXIS2_PLACEMENT_3D ( 'NONE', #48863, #69716, #75879 ) ;
#41254=DIRECTION ( 'NONE',  ( -3.330669073875469227E-15, 0.000000000000000000, 1.000000000000000000 ) ) ;
#41255=EDGE_CURVE ( 'NONE', #61775, #70776, #54948, .T. ) ;
#41256=VECTOR ( 'NONE', #56510, 1000.000000000000000 ) ;
#41260=EDGE_CURVE ( 'NONE', #1135, #27540, #89389, .T. ) ;
#41262=ORIENTED_EDGE ( 'NONE', *, *, #6894, .F. ) ;
#41264=CIRCLE ( 'NONE', #4999, 0.4999999999999923395 ) ;
#41270=ORIENTED_EDGE ( 'NONE', *, *, #14110, .T. ) ;
#41273=VECTOR ( 'NONE', #1347, 1000.000000000000000 ) ;
#41284=CIRCLE ( 'NONE', #74562, 7.500000000000012434 ) ;
#41307=CARTESIAN_POINT ( 'NONE',  ( 159.0442047513576824, 16.65459343288188165, -10.27557066714188139 ) ) ;
#41312=CARTESIAN_POINT ( 'NONE',  ( 154.9307753191121435, 19.94580804509866567, -10.40578999956973405 ) ) ;
#41319=CIRCLE ( 'NONE', #53440, 4.000000000000003553 ) ;
#41323=MECHANICAL_DESIGN_GEOMETRIC_PRESENTATION_REPRESENTATION('',(#17149),#48918);
#41324=EDGE_LOOP ( 'NONE', ( #83660, #79692, #31644, #80954 ) ) ;
#41330=ORIENTED_EDGE ( 'NONE', *, *, #51459, .T. ) ;
#41335=AXIS2_PLACEMENT_3D ( 'NONE', #41667, #25589, #54473 ) ;
#41338=EDGE_CURVE ( 'NONE', #88799, #63820, #45818, .T. ) ;
#41349=DIRECTION ( 'NONE',  ( 0.000000000000000000, 1.000000000000000000, 0.000000000000000000 ) ) ;
#41351=CIRCLE ( 'NONE', #2110, 3.000000000000000888 ) ;
#41368=ORIENTED_EDGE ( 'NONE', *, *, #74810, .T. ) ;
#41382=EDGE_CURVE ( 'NONE', #14856, #66468, #80639, .T. ) ;
#41391=ORIENTED_EDGE ( 'NONE', *, *, #29603, .T. ) ;
#41393=ORIENTED_EDGE ( 'NONE', *, *, #19155, .T. ) ;
#41395=AXIS2_PLACEMENT_3D ( 'NONE', #10315, #4622, #33495 ) ;
#41401=CARTESIAN_POINT ( 'NONE',  ( 175.2296996224750103, 250.0000000000000568, 0.000000000000000000 ) ) ;
#41408=TOROIDAL_SURFACE ( 'NONE', #626, 4.499999999999993783, 0.5000000000000000000 ) ;
#41426=CARTESIAN_POINT ( 'NONE',  ( 161.2244399300530233, 8.542400036368780647, 10.00000000000000000 ) ) ;
#41430=CARTESIAN_POINT ( 'NONE',  ( 159.4851178187871312, 15.00000000000000000, 6.999999999999998224 ) ) ;
#41443=CARTESIAN_POINT ( 'NONE',  ( 208.0393982316568326, 37.47427918878998554, 12.98477611641282614 ) ) ;
#41446=DIRECTION ( 'NONE',  ( -0.000000000000000000, -1.000000000000000000, -0.000000000000000000 ) ) ;
#41462=TOROIDAL_SURFACE ( 'NONE', #684, 24.16304133878946558, 4.003189038634632269 ) ;
#41464=CARTESIAN_POINT ( 'NONE',  ( 155.0786878258427066, 18.48484813926865655, 9.250287988714237741 ) ) ;
#41472=VECTOR ( 'NONE', #48189, 1000.000000000000000 ) ;
#41488=CARTESIAN_POINT ( 'NONE',  ( 196.8803347170859865, 73.40565171261609123, -12.49999999999998579 ) ) ;
#41489=CARTESIAN_POINT ( 'NONE',  ( 153.7700350902760533, 129.6490463903463990, -11.80126012119838030 ) ) ;
#41498=EDGE_CURVE ( 'NONE', #66468, #88799, #87995, .T. ) ;
#41502=AXIS2_PLACEMENT_3D ( 'NONE', #31713, #60605, #1431 ) ;
#41504=ORIENTED_EDGE ( 'NONE', *, *, #79580, .T. ) ;
#41508=EDGE_LOOP ( 'NONE', ( #7403, #32668, #75859, #52877, #42314 ) ) ;
#41511=DIRECTION ( 'NONE',  ( -0.000000000000000000, -1.000000000000000000, -0.000000000000000000 ) ) ;
#41513=CARTESIAN_POINT ( 'NONE',  ( 156.6695768423687696, 18.03393767896977451, 8.087387968559804463 ) ) ;
#41519=CARTESIAN_POINT ( 'NONE',  ( 196.1227023549103592, 275.0000000000000568, -11.81026827902096521 ) ) ;
#41520=CARTESIAN_POINT ( 'NONE',  ( 152.4536156746142410, 275.0000000000000568, -11.50000000000000355 ) ) ;
#41524=CARTESIAN_POINT ( 'NONE',  ( 184.7149167944524493, 8.542400036368780647, -9.000000000000001776 ) ) ;
#41537=EDGE_CURVE ( 'NONE', #50728, #28948, #55776, .T. ) ;
#41539=CARTESIAN_POINT ( 'NONE',  ( 193.6552470326849402, 275.5000000000000568, 16.89672165344822119 ) ) ;
#41579=CARTESIAN_POINT ( 'NONE',  ( 175.2296996224750103, 140.2072866198470251, 24.00000000000002132 ) ) ;
#41592=CARTESIAN_POINT ( 'NONE',  ( 194.8488057663960831, 40.40495866097701594, 13.83703082863031497 ) ) ;
#41595=CYLINDRICAL_SURFACE ( 'NONE', #88412, 0.5000000000000000000 ) ;
#41597=EDGE_CURVE ( 'NONE', #85293, #38685, #71619, .T. ) ;
#41598=ORIENTED_EDGE ( 'NONE', *, *, #34788, .F. ) ;
#41604=CARTESIAN_POINT ( 'NONE',  ( 196.9312215853254600, 70.66127120904285164, -10.51348395302562722 ) ) ;
#41605=DIRECTION ( 'NONE',  ( -0.7957555401921962979, -0.6056179655966504871, 0.000000000000000000 ) ) ;
#41606=DIRECTION ( 'NONE',  ( -0.000000000000000000, -1.000000000000000000, -0.000000000000000000 ) ) ;
#41627=ORIENTED_EDGE ( 'NONE', *, *, #82958, .T. ) ;
#41631=ADVANCED_FACE ( 'NONE', ( #53899 ), #70045, .T. ) ;
#41640=CIRCLE ( 'NONE', #841, 0.4999999999999998335 ) ;
#41644=ORIENTED_EDGE ( 'NONE', *, *, #46824, .T. ) ;
#41646=CARTESIAN_POINT ( 'NONE',  ( 194.8949733755876252, 19.89707320078522557, -13.96765070539848530 ) ) ;
#41654=CARTESIAN_POINT ( 'NONE',  ( 189.9243309297870610, 250.0000000000000568, 20.22542485937349355 ) ) ;
#41660=DIRECTION ( 'NONE',  ( 0.000000000000000000, 1.000000000000000000, 0.000000000000000000 ) ) ;
#41667=CARTESIAN_POINT ( 'NONE',  ( 175.2296996224750103, 128.0000000000000568, 0.000000000000000000 ) ) ;
#41669=DIRECTION ( 'NONE',  ( 0.000000000000000000, 0.000000000000000000, 1.000000000000000000 ) ) ;
#41680=DIRECTION ( 'NONE',  ( 0.000000000000000000, 0.000000000000000000, -1.000000000000000000 ) ) ;
#41688=EDGE_CURVE ( 'NONE', #86306, #72022, #61491, .T. ) ;
#41691=VERTEX_POINT ( 'NONE', #76616 ) ;
#41692=CARTESIAN_POINT ( 'NONE',  ( 221.4259212729440094, 36.93618551656547311, -7.000000000000000888 ) ) ;
#41694=CARTESIAN_POINT ( 'NONE',  ( 186.2362647323748206, 250.5000000000000568, 22.80382896336985965 ) ) ;
#41707=DIRECTION ( 'NONE',  ( -1.000000000000000000, 0.000000000000000000, 0.000000000000000000 ) ) ;
#41709=EDGE_CURVE ( 'NONE', #6120, #24267, #47234, .T. ) ;
#41724=VERTEX_POINT ( 'NONE', #3234 ) ;
#41729=( LENGTH_UNIT ( ) NAMED_UNIT ( * ) SI_UNIT ( .MILLI., .METRE. ) );
#41734=VERTEX_POINT ( 'NONE', #11739 ) ;
#41741=CARTESIAN_POINT ( 'NONE',  ( 175.2296996224750103, 20.99999999999998934, 0.000000000000000000 ) ) ;
#41751=EDGE_CURVE ( 'NONE', #86547, #63082, #39854, .T. ) ;
#41754=EDGE_LOOP ( 'NONE', ( #52556, #93444, #4944, #15802 ) ) ;
#41755=FACE_OUTER_BOUND ( 'NONE', #37677, .T. ) ;
#41758=ADVANCED_FACE ( 'NONE', ( #19777 ), #91259, .F. ) ;
#41767=DIRECTION ( 'NONE',  ( 1.000000000000000000, 0.000000000000000000, 0.000000000000000000 ) ) ;
#41773=CARTESIAN_POINT ( 'NONE',  ( 199.0743954165634761, 275.0000000000000568, -2.725891136377206703 ) ) ;
#41783=CARTESIAN_POINT ( 'NONE',  ( 180.7287904564219332, 215.0000000000000568, -24.90000000000002345 ) ) ;
#41792=DIRECTION ( 'NONE',  ( 0.000000000000000000, 0.000000000000000000, 1.000000000000000000 ) ) ;
#41794=CARTESIAN_POINT ( 'NONE',  ( 139.1539576904058606, 276.0000000000000568, 10.50000000000000000 ) ) ;
#41797=CARTESIAN_POINT ( 'NONE',  ( 175.2296996224750103, 275.5000000000000568, 0.000000000000000000 ) ) ;
#41810=CARTESIAN_POINT ( 'NONE',  ( 209.2568086740250237, 34.98978593258875236, 12.09245862095555601 ) ) ;
#41827=DIRECTION ( 'NONE',  ( -1.000000000000000000, 0.000000000000000000, 0.000000000000000000 ) ) ;
#41871=EDGE_CURVE ( 'NONE', #13111, #30328, #48944, .T. ) ;
#41872=ORIENTED_EDGE ( 'NONE', *, *, #27827, .T. ) ;
#41879=CARTESIAN_POINT ( 'NONE',  ( 151.7498149058220918, 20.88232504567557513, -8.615841630442520938 ) ) ;
#41884=CARTESIAN_POINT ( 'NONE',  ( 154.1407330040854333, 250.5000000000000568, 13.42592592592592915 ) ) ;
#41891=CARTESIAN_POINT ( 'NONE',  ( 175.2296996224750103, 246.0000000000001137, 0.000000000000000000 ) ) ;
#41899=DIRECTION ( 'NONE',  ( -0.6632250457539263788, -5.193207171581228641E-15, 0.7484200282493129741 ) ) ;
#41903=CYLINDRICAL_SURFACE ( 'NONE', #8105, 4.000000000000003553 ) ;
#41916=CARTESIAN_POINT ( 'NONE',  ( 208.0393982316568326, 37.47427918878999265, 11.99999999999999822 ) ) ;
#41918=EDGE_CURVE ( 'NONE', #46489, #27188, #74627, .T. ) ;
#41921=CARTESIAN_POINT ( 'NONE',  ( 203.5977283565847813, 62.01285785379744198, 7.000000000000000000 ) ) ;
#41938=CARTESIAN_POINT ( 'NONE',  ( 155.4202369374260400, 19.37982107812020871, 12.54055055082743309 ) ) ;
#41958=FACE_OUTER_BOUND ( 'NONE', #29857, .T. ) ;
#41959=DIRECTION ( 'NONE',  ( 0.000000000000000000, 0.000000000000000000, 1.000000000000000000 ) ) ;
#41972=ORIENTED_EDGE ( 'NONE', *, *, #31412, .T. ) ;
#41976=ORIENTED_EDGE ( 'NONE', *, *, #3596, .F. ) ;
#41977=CARTESIAN_POINT ( 'NONE',  ( 212.4629471475955427, 32.98517505407394168, 9.000000000000001776 ) ) ;
#41979=CARTESIAN_POINT ( 'NONE',  ( 175.2296996224750103, 142.2541816238762920, 24.00000000000001066 ) ) ;
#41985=CARTESIAN_POINT ( 'NONE',  ( 154.5567693064130026, 20.34893504152563537, 12.19321973754205857 ) ) ;
#41989=ORIENTED_EDGE ( 'NONE', *, *, #56745, .T. ) ;
#41990=CYLINDRICAL_SURFACE ( 'NONE', #67113, 4.999999999999978684 ) ;
#42004=CARTESIAN_POINT ( 'NONE',  ( 199.0061125298537377, 250.0000000000000568, -7.725424859374024678 ) ) ;
#42005=CYLINDRICAL_SURFACE ( 'NONE', #2003, 6.000000000000000000 ) ;
#42018=CARTESIAN_POINT ( 'NONE',  ( 151.4990405259949569, 130.0000000000000568, -12.50000000000000178 ) ) ;
#42020=CARTESIAN_POINT ( 'NONE',  ( 196.7320021107339301, 20.33855172480464546, 12.75691961062094570 ) ) ;
#42021=AXIS2_PLACEMENT_3D ( 'NONE', #76524, #11647, #90683 ) ;
#42029=EDGE_CURVE ( 'NONE', #45543, #1135, #4637, .T. ) ;
#42034=CARTESIAN_POINT ( 'NONE',  ( 196.0553440093420079, 41.98397561837970215, 13.83198452061308359 ) ) ;
#42043=DIRECTION ( 'NONE',  ( 0.000000000000000000, 0.000000000000000000, 1.000000000000000000 ) ) ;
#42045=CARTESIAN_POINT ( 'NONE',  ( 140.6539576904058606, 275.5000000000000568, -10.49999999999999822 ) ) ;
#42056=EDGE_LOOP ( 'NONE', ( #19746, #56213, #30811, #89105, #15538, #50356, #87713 ) ) ;
#42057=CARTESIAN_POINT ( 'NONE',  ( 194.7685530992919780, 41.40013651751808510, 13.93755082198983075 ) ) ;
#42062=ORIENTED_EDGE ( 'NONE', *, *, #42403, .T. ) ;
#42069=CARTESIAN_POINT ( 'NONE',  ( 185.0172044724083946, 250.5000000000000568, 22.46007009812148070 ) ) ;
#42070=CARTESIAN_POINT ( 'NONE',  ( 200.4644824113734671, 275.0000000000000568, -2.942835885954290465 ) ) ;
#42089=LINE ( 'NONE', #93691, #87701 ) ;
#42103=EDGE_LOOP ( 'NONE', ( #20443, #45557, #80130, #5430 ) ) ;
#42104=ORIENTED_EDGE ( 'NONE', *, *, #21510, .T. ) ;
#42113=DIRECTION ( 'NONE',  ( -0.000000000000000000, -0.000000000000000000, -1.000000000000000000 ) ) ;
#42119=DIRECTION ( 'NONE',  ( -0.000000000000000000, -1.000000000000000000, -0.000000000000000000 ) ) ;
#42120=DIRECTION ( 'NONE',  ( -0.000000000000000000, 0.000000000000000000, -1.000000000000000000 ) ) ;
#42126=EDGE_CURVE ( 'NONE', #76803, #64817, #32499, .T. ) ;
#42128=EDGE_CURVE ( 'NONE', #78327, #83522, #9593, .T. ) ;
#42142=CARTESIAN_POINT ( 'NONE',  ( 198.1245416649653919, 70.21476723776075346, -10.41797401930329592 ) ) ;
#42157=LINE ( 'NONE', #63991, #74572 ) ;
#42165=EDGE_CURVE ( 'NONE', #5311, #13346, #8124, .T. ) ;
#42170=( BOUNDED_CURVE ( )  B_SPLINE_CURVE ( 3, ( #34708, #64567, #92931, #49384 ),
 .UNSPECIFIED., .F., .F. ) 
 B_SPLINE_CURVE_WITH_KNOTS ( ( 4, 4 ),
 ( 3.141592653589793116, 4.289818581637806716 ),
 .UNSPECIFIED. ) 
 CURVE ( )  GEOMETRIC_REPRESENTATION_ITEM ( )  RATIONAL_B_SPLINE_CURVE ( ( 1.000000000000000000, 0.8931162488198155502, 0.8931162488198155502, 1.000000000000000000 ) ) 
 REPRESENTATION_ITEM ( '' )  );
#42173=CARTESIAN_POINT ( 'NONE',  ( 208.6208076322478746, 32.98517505407394168, 12.09245862095555601 ) ) ;
#42185=ORIENTED_EDGE ( 'NONE', *, *, #91432, .F. ) ;
#42196=ORIENTED_EDGE ( 'NONE', *, *, #47322, .T. ) ;
#42216=ORIENTED_EDGE ( 'NONE', *, *, #36169, .F. ) ;
#42217=FACE_OUTER_BOUND ( 'NONE', #74124, .T. ) ;
#42222=CIRCLE ( 'NONE', #22557, 24.50000000000000355 ) ;
#42239=ORIENTED_EDGE ( 'NONE', *, *, #74648, .F. ) ;
#42248=PLANE ( 'NONE',  #39777 ) ;
#42254=CARTESIAN_POINT ( 'NONE',  ( 193.5407187895461618, 250.2122328390418602, 16.89624193607488323 ) ) ;
#42258=CARTESIAN_POINT ( 'NONE',  ( 208.6208076322478746, 32.98517505407394168, 14.26380412667038655 ) ) ;
#42261=B_SPLINE_CURVE_WITH_KNOTS ( 'NONE', 3,
 ( #82921, #17145, #46468, #23320 ),
 .UNSPECIFIED., .F., .F.,
 ( 4, 4 ),
 ( 0.000000000000000000, 9.632970524406852609E-05 ),
 .UNSPECIFIED. ) ;
#42262=DIRECTION ( 'NONE',  ( 0.000000000000000000, 0.000000000000000000, -1.000000000000000000 ) ) ;
#42271=ADVANCED_FACE ( 'NONE', ( #34463 ), #32320, .F. ) ;
#42272=EDGE_CURVE ( 'NONE', #71428, #23799, #68551, .T. ) ;
#42279=EDGE_LOOP ( 'NONE', ( #30953, #31415, #37114, #2735 ) ) ;
#42281=ORIENTED_EDGE ( 'NONE', *, *, #58419, .T. ) ;
#42290=ORIENTED_EDGE ( 'NONE', *, *, #40031, .F. ) ;
#42294=EDGE_CURVE ( 'NONE', #74338, #66586, #55027, .T. ) ;
#42307=CARTESIAN_POINT ( 'NONE',  ( 175.2296996224750103, 133.0000000000000000, 0.000000000000000000 ) ) ;
#42314=ORIENTED_EDGE ( 'NONE', *, *, #73681, .T. ) ;
#42333=ORIENTED_EDGE ( 'NONE', *, *, #46568, .T. ) ;
#42339=EDGE_LOOP ( 'NONE', ( #18780, #32200, #23130, #90074, #67636 ) ) ;
#42342=B_SPLINE_CURVE_WITH_KNOTS ( 'NONE', 3,
 ( #1180, #15859, #58026, #50903, #28213, #58488 ),
 .UNSPECIFIED., .F., .F.,
 ( 4, 2, 4 ),
 ( -4.472146915458784344E-06, 0.0004206930844425981289, 0.0008458583158006550539 ),
 .UNSPECIFIED. ) ;
#42349=DIRECTION ( 'NONE',  ( -0.000000000000000000, -0.000000000000000000, 1.000000000000000000 ) ) ;
#42354=DIRECTION ( 'NONE',  ( 0.000000000000000000, 1.000000000000000000, -0.000000000000000000 ) ) ;
#42358=CIRCLE ( 'NONE', #31817, 5.000000000000000888 ) ;
#42366=DIRECTION ( 'NONE',  ( 0.000000000000000000, 0.000000000000000000, 1.000000000000000000 ) ) ;
#42369=DIRECTION ( 'NONE',  ( -0.000000000000000000, -0.000000000000000000, 1.000000000000000000 ) ) ;
#42373=CARTESIAN_POINT ( 'NONE',  ( 198.0449163674539079, 67.45573463390418567, -11.11900013380403962 ) ) ;
#42385=FACE_OUTER_BOUND ( 'NONE', #61061, .T. ) ;
#42389=CARTESIAN_POINT ( 'NONE',  ( 222.0386546523673985, 36.13108063356137478, -7.000000000000000888 ) ) ;
#42395=EDGE_CURVE ( 'NONE', #28813, #34201, #64135, .T. ) ;
#42403=EDGE_CURVE ( 'NONE', #37341, #32542, #59502, .T. ) ;
#42417=ORIENTED_EDGE ( 'NONE', *, *, #41382, .T. ) ;
#42426=VECTOR ( 'NONE', #20060, 1000.000000000000000 ) ;
#42429=LINE ( 'NONE', #21133, #56543 ) ;
#42430=CARTESIAN_POINT ( 'NONE',  ( 153.0292788520805232, 130.2722548028652909, -11.54371207238995645 ) ) ;
#42432=CIRCLE ( 'NONE', #30338, 2.000000000000010658 ) ;
#42434=ORIENTED_EDGE ( 'NONE', *, *, #42126, .T. ) ;
#42443=VERTEX_POINT ( 'NONE', #48312 ) ;
#42447=ORIENTED_EDGE ( 'NONE', *, *, #48576, .F. ) ;
#42449=FACE_OUTER_BOUND ( 'NONE', #21985, .T. ) ;
#42450=CARTESIAN_POINT ( 'NONE',  ( 194.3144103428324172, 249.5000000000000568, 16.91223866672520515 ) ) ;
#42456=EDGE_CURVE ( 'NONE', #9812, #19395, #37993, .T. ) ;
#42457=LINE ( 'NONE', #91239, #89590 ) ;
#42458=ADVANCED_FACE ( 'NONE', ( #77213 ), #33182, .F. ) ;
#42459=DIRECTION ( 'NONE',  ( 0.000000000000000000, 0.000000000000000000, 1.000000000000000000 ) ) ;
#42461=VERTEX_POINT ( 'NONE', #91401 ) ;
#42463=DIRECTION ( 'NONE',  ( 0.000000000000000000, 0.000000000000000000, 1.000000000000000000 ) ) ;
#42477=CARTESIAN_POINT ( 'NONE',  ( 195.6227410709891501, 26.52170211303658576, 13.75379487587555438 ) ) ;
#42491=DIRECTION ( 'NONE',  ( 0.000000000000000000, 1.000000000000000000, 0.000000000000000000 ) ) ;
#42493=CARTESIAN_POINT ( 'NONE',  ( 195.5378547391706263, 20.94045493971685090, 14.59381989330956131 ) ) ;
#42498=AXIS2_PLACEMENT_3D ( 'NONE', #22389, #7260, #79699 ) ;
#42503=FACE_OUTER_BOUND ( 'NONE', #31457, .T. ) ;
#42517=EDGE_LOOP ( 'NONE', ( #7535, #68727, #90919, #57380 ) ) ;
#42518=CARTESIAN_POINT ( 'NONE',  ( 153.6987871352777404, 19.48326534539592103, 11.45812909364015297 ) ) ;
#42529=ORIENTED_EDGE ( 'NONE', *, *, #1899, .F. ) ;
#42535=ORIENTED_EDGE ( 'NONE', *, *, #41498, .F. ) ;
#42541=FACE_OUTER_BOUND ( 'NONE', #23189, .T. ) ;
#42542=CARTESIAN_POINT ( 'NONE',  ( 196.4364563510924881, 72.07553028462349687, -11.29011490108475080 ) ) ;
#42552=VERTEX_POINT ( 'NONE', #26072 ) ;
#42570=EDGE_CURVE ( 'NONE', #13568, #49791, #3364, .T. ) ;
#42578=EDGE_LOOP ( 'NONE', ( #17509, #31513, #21283, #41007 ) ) ;
#42618=CARTESIAN_POINT ( 'NONE',  ( 196.8803347170859865, 73.40565171261611965, -12.50000000000000178 ) ) ;
#42629=ORIENTED_EDGE ( 'NONE', *, *, #88532, .T. ) ;
#42637=AXIS2_PLACEMENT_3D ( 'NONE', #89058, #17119, #24207 ) ;
#42647=FACE_OUTER_BOUND ( 'NONE', #32199, .T. ) ;
#42660=ORIENTED_EDGE ( 'NONE', *, *, #31148, .F. ) ;
#42665=EDGE_CURVE ( 'NONE', #62986, #46709, #55444, .T. ) ;
#42669=EDGE_LOOP ( 'NONE', ( #48391, #30450 ) ) ;
#42680=ORIENTED_EDGE ( 'NONE', *, *, #42395, .F. ) ;
#42688=CARTESIAN_POINT ( 'NONE',  ( 195.7761921920649684, 26.31373072850298556, 13.59762452525894005 ) ) ;
#42691=ADVANCED_FACE ( 'NONE', ( #86053 ), #25150, .T. ) ;
#42700=CARTESIAN_POINT ( 'NONE',  ( 222.8344101925596306, 0.000000000000000000, 7.000000000000000000 ) ) ;
#42701=AXIS2_PLACEMENT_3D ( 'NONE', #74183, #11184, #9301 ) ;
#42709=AXIS2_PLACEMENT_3D ( 'NONE', #71060, #50194, #14708 ) ;
#42718=CARTESIAN_POINT ( 'NONE',  ( 153.4734828627512400, 20.31592703335031658, 12.31730288665599637 ) ) ;
#42724=CARTESIAN_POINT ( 'NONE',  ( 208.8547504194143585, 36.42232975996840594, 14.79569954156338518 ) ) ;
#42726=( BOUNDED_SURFACE ( )  B_SPLINE_SURFACE ( 3, 2, ( 
 ( #35129, #72523, #64051 ),
 ( #7643, #72078, #20930 ),
 ( #49799, #14316, #64530 ),
 ( #44080, #65443, #7194 ),
 ( #78696, #558, #29442 ),
 ( #36069, #87174, #51194 ),
 ( #15224, #13837, #57398 ),
 ( #72982, #8112, #42688 ),
 ( #36999, #6742, #1024 ),
 ( #29902, #58786, #49343 ),
 ( #92894, #28053, #71607 ),
 ( #35615, #93355, #38376 ),
 ( #30832, #73907, #67745 ),
 ( #74366, #75308, #24645 ) ),
 .UNSPECIFIED., .F., .F., .F. ) 
 B_SPLINE_SURFACE_WITH_KNOTS ( ( 4, 2, 2, 2, 2, 2, 4 ),
 ( 3, 3 ),
 ( -2.168404344971008868E-19, 0.001236320232021350003, 0.001854480348032025222, 0.002472640464042700440, 0.003090800580053375442, 0.003708960696064050877, 0.004945280928085400880 ),
 ( 0.000000000000000000, 1.000000000000000000 ),
 .UNSPECIFIED. ) 
 GEOMETRIC_REPRESENTATION_ITEM ( )  RATIONAL_B_SPLINE_SURFACE ( (
 ( 1.000000000000000000, 0.8108476219622871017, 1.000000000000000000),
 ( 1.000000000000000000, 0.8255659973200745183, 1.000000000000000000),
 ( 1.000000000000000000, 0.8395011523818814991, 1.000000000000000000),
 ( 1.000000000000000000, 0.8588211550372549796, 1.000000000000000000),
 ( 1.000000000000000000, 0.8649348442247967172, 1.000000000000000000),
 ( 1.000000000000000000, 0.8760455507362673311, 1.000000000000000000),
 ( 1.000000000000000000, 0.8810998449848480574, 1.000000000000000000),
 ( 1.000000000000000000, 0.8900036393291742565, 1.000000000000000000),
 ( 1.000000000000000000, 0.8938622710282666528, 1.000000000000000000),
 ( 1.000000000000000000, 0.8997338558213243687, 1.000000000000000000),
 ( 1.000000000000000000, 0.9018082123500091862, 1.000000000000000000),
 ( 1.000000000000000000, 0.9050182246960185584, 1.000000000000000000),
 ( 1.000000000000000000, 0.9029724514278080205, 1.000000000000000000),
 ( 1.000000000000000000, 0.8966167345234238306, 1.000000000000000000) ) ) 
 REPRESENTATION_ITEM ( '' )  SURFACE ( )  );
#42727=CARTESIAN_POINT ( 'NONE',  ( 180.7287904564219332, 250.5000000000000568, -24.90000000000003411 ) ) ;
#42730=DIRECTION ( 'NONE',  ( -0.09665007798479426093, -1.048651511008089408E-15, -0.9953184226294282677 ) ) ;
#42731=CARTESIAN_POINT ( 'NONE',  ( 157.4851178187871312, 15.19241473665941378, -8.999999999999666045 ) ) ;
#42738=( BOUNDED_CURVE ( )  B_SPLINE_CURVE ( 3, ( #80811, #88828, #89286, #51921 ),
 .UNSPECIFIED., .F., .F. ) 
 B_SPLINE_CURVE_WITH_KNOTS ( ( 4, 4 ),
 ( 3.141592653589793116, 4.712388980384689674 ),
 .UNSPECIFIED. ) 
 CURVE ( )  GEOMETRIC_REPRESENTATION_ITEM ( )  RATIONAL_B_SPLINE_CURVE ( ( 1.000000000000000000, 0.8047378541243649375, 0.8047378541243649375, 1.000000000000000000 ) ) 
 REPRESENTATION_ITEM ( '' )  );
#42742=EDGE_LOOP ( 'NONE', ( #22898, #66355, #38503, #50016 ) ) ;
#42745=CARTESIAN_POINT ( 'NONE',  ( 196.8803347170859865, 24.42324672360810212, 12.49999999999999289 ) ) ;
#42747=ORIENTED_EDGE ( 'NONE', *, *, #47247, .T. ) ;
#42762=PLANE ( 'NONE',  #10725 ) ;
#42763=AXIS2_PLACEMENT_3D ( 'NONE', #64202, #78373, #13978 ) ;
#42765=CIRCLE ( 'NONE', #39694, 5.603083949679982467 ) ;
#42771=AXIS2_PLACEMENT_3D ( 'NONE', #11410, #47370, #89998 ) ;
#42773=TOROIDAL_SURFACE ( 'NONE', #54800, 24.50000000000000355, 0.5000000000000000000 ) ;
#42777=AXIS2_PLACEMENT_3D ( 'NONE', #35889, #74072, #88273 ) ;
#42785=VERTEX_POINT ( 'NONE', #39792 ) ;
#42787=AXIS2_PLACEMENT_3D ( 'NONE', #4152, #53872, #33022 ) ;
#42805=ORIENTED_EDGE ( 'NONE', *, *, #78996, .T. ) ;
#42808=CIRCLE ( 'NONE', #38186, 2.000000000000000000 ) ;
#42814=ADVANCED_FACE ( 'NONE', ( #11872 ), #57212, .T. ) ;
#42815=ORIENTED_EDGE ( 'NONE', *, *, #68345, .T. ) ;
#42824=DIRECTION ( 'NONE',  ( 0.000000000000000000, 0.000000000000000000, 1.000000000000000000 ) ) ;
#42836=FACE_OUTER_BOUND ( 'NONE', #76659, .T. ) ;
#42850=DIRECTION ( 'NONE',  ( 1.000000000000000000, 0.000000000000000000, 0.000000000000000000 ) ) ;
#42870=CIRCLE ( 'NONE', #62492, 7.500000000000012434 ) ;
#42879=EDGE_CURVE ( 'NONE', #42461, #24392, #47432, .T. ) ;
#42894=ORIENTED_EDGE ( 'NONE', *, *, #33978, .T. ) ;
#42897=VECTOR ( 'NONE', #70810, 1000.000000000000000 ) ;
#42905=DIRECTION ( 'NONE',  ( -1.000000000000000000, 0.000000000000000000, -5.880589007913310608E-16 ) ) ;
#42911=ORIENTED_EDGE ( 'NONE', *, *, #42165, .T. ) ;
#42917=VECTOR ( 'NONE', #50893, 1000.000000000000000 ) ;
#42927=CIRCLE ( 'NONE', #8179, 24.00000000000001066 ) ;
#42929=FACE_OUTER_BOUND ( 'NONE', #10544, .T. ) ;
#42930=AXIS2_PLACEMENT_3D ( 'NONE', #15969, #8386, #8838 ) ;
#42936=FACE_OUTER_BOUND ( 'NONE', #45567, .T. ) ;
#42937=DIRECTION ( 'NONE',  ( 1.000000000000000000, 0.000000000000000000, -0.000000000000000000 ) ) ;
#42939=AXIS2_PLACEMENT_3D ( 'NONE', #63412, #86074, #65274 ) ;
#42940=ADVANCED_FACE ( 'NONE', ( #4768 ), #27813, .T. ) ;
#42941=CARTESIAN_POINT ( 'NONE',  ( 195.4781563537916043, 27.48493576247232184, 15.50000000000000000 ) ) ;
#42943=ORIENTED_EDGE ( 'NONE', *, *, #18516, .F. ) ;
#42944=DIRECTION ( 'NONE',  ( 0.000000000000000000, 0.000000000000000000, -1.000000000000000000 ) ) ;
#42960=CARTESIAN_POINT ( 'NONE',  ( 186.6539576904058890, 293.9636489450775230, -11.60392986742922261 ) ) ;
#42974=CARTESIAN_POINT ( 'NONE',  ( 138.6539576904058606, 132.0000000000000568, 10.50000000000000000 ) ) ;
#42976=CYLINDRICAL_SURFACE ( 'NONE', #30896, 2.000000000000005329 ) ;
#42980=AXIS2_PLACEMENT_3D ( 'NONE', #9632, #52261, #44688 ) ;
#42984=CARTESIAN_POINT ( 'NONE',  ( 208.6364533529840912, 29.41061770585039881, 14.73339628615688568 ) ) ;
#42992=CARTESIAN_POINT ( 'NONE',  ( 192.9182251362765328, 275.0000000000000568, 16.22085278731030300 ) ) ;
#43000=AXIS2_PLACEMENT_3D ( 'NONE', #36056, #71592, #79155 ) ;
#43004=ORIENTED_EDGE ( 'NONE', *, *, #60248, .F. ) ;
#43007=DIRECTION ( 'NONE',  ( 0.000000000000000000, 0.000000000000000000, -1.000000000000000000 ) ) ;
#43017=ORIENTED_EDGE ( 'NONE', *, *, #29167, .T. ) ;
#43018=CARTESIAN_POINT ( 'NONE',  ( 194.5467258271157220, 40.92429273362547093, 14.24314089363953961 ) ) ;
#43024=VERTEX_POINT ( 'NONE', #1746 ) ;
#43030=DIRECTION ( 'NONE',  ( -0.000000000000000000, -0.000000000000000000, -1.000000000000000000 ) ) ;
#43031=DIRECTION ( 'NONE',  ( 0.000000000000000000, 0.000000000000000000, 1.000000000000000000 ) ) ;
#43042=ORIENTED_EDGE ( 'NONE', *, *, #85122, .F. ) ;
#43064=ORIENTED_EDGE ( 'NONE', *, *, #67705, .F. ) ;
#43082=CARTESIAN_POINT ( 'NONE',  ( 180.2288731078812702, 250.5000000000000568, -24.90909090909093848 ) ) ;
#43084=CIRCLE ( 'NONE', #2259, 3.342139515347647638 ) ;
#43092=CARTESIAN_POINT ( 'NONE',  ( 208.6208076322478746, 32.98517505407394168, 13.99999999999999822 ) ) ;
#43094=CARTESIAN_POINT ( 'NONE',  ( 152.4536156746142410, 276.0000000000000568, 11.99999999999999289 ) ) ;
#43103=DIRECTION ( 'NONE',  ( -1.000000000000000000, 0.000000000000000000, 0.000000000000000000 ) ) ;
#43105=CARTESIAN_POINT ( 'NONE',  ( 200.2349812190172713, 66.43136063442170780, -7.741079165001064410 ) ) ;
#43106=CARTESIAN_POINT ( 'NONE',  ( 183.0442525570908288, 293.9636489450775230, 0.000000000000000000 ) ) ;
#43116=ORIENTED_EDGE ( 'NONE', *, *, #18686, .F. ) ;
#43117=CYLINDRICAL_SURFACE ( 'NONE', #45313, 1.499999999999998002 ) ;
#43123=EDGE_CURVE ( 'NONE', #307, #12757, #48055, .T. ) ;
#43133=CARTESIAN_POINT ( 'NONE',  ( 199.6702811234769968, 65.52214591209386185, -9.100946541886345997 ) ) ;
#43146=CIRCLE ( 'NONE', #17400, 0.4999999999999991118 ) ;
#43148=ORIENTED_EDGE ( 'NONE', *, *, #50173, .F. ) ;
#43157=ORIENTED_EDGE ( 'NONE', *, *, #40105, .F. ) ;
#43163=CARTESIAN_POINT ( 'NONE',  ( 208.6208076322478746, 32.98517505407394168, 10.50000000000000000 ) ) ;
#43175=ORIENTED_EDGE ( 'NONE', *, *, #59326, .T. ) ;
#43176=CARTESIAN_POINT ( 'NONE',  ( 189.9243309297870610, 250.5000000000000568, 20.22542485937349355 ) ) ;
#43186=DIRECTION ( 'NONE',  ( 0.000000000000000000, 1.000000000000000000, 0.000000000000000000 ) ) ;
#43202=CARTESIAN_POINT ( 'NONE',  ( 154.0637704119390321, 19.72112694978655512, 13.30738029212319340 ) ) ;
#43210=VECTOR ( 'NONE', #7861, 1000.000000000000000 ) ;
#43214=CARTESIAN_POINT ( 'NONE',  ( 196.1554417525619272, 24.76049057409047549, 13.68028117252083042 ) ) ;
#43215=LINE ( 'NONE', #27139, #92647 ) ;
#43223=EDGE_CURVE ( 'NONE', #55107, #38347, #36339, .T. ) ;
#43230=ORIENTED_EDGE ( 'NONE', *, *, #66684, .F. ) ;
#43246=DIRECTION ( 'NONE',  ( 1.000000000000000000, 0.000000000000000000, 0.000000000000000000 ) ) ;
#43260=ORIENTED_EDGE ( 'NONE', *, *, #80560, .F. ) ;
#43280=ORIENTED_EDGE ( 'NONE', *, *, #43123, .T. ) ;
#43282=AXIS2_PLACEMENT_3D ( 'NONE', #83645, #18809, #47666 ) ;
#43300=LINE ( 'NONE', #72197, #27577 ) ;
#43303=ADVANCED_FACE ( 'NONE', ( #86513 ), #48810, .T. ) ;
#43304=( BOUNDED_SURFACE ( )  B_SPLINE_SURFACE ( 3, 2, ( 
 ( #1829, #17446, #29795 ),
 ( #24065, #81353, #16503 ),
 ( #31193, #65804, #59614 ),
 ( #916, #23612, #46296 ),
 ( #51539, #38263, #22666 ),
 ( #87980, #67176, #30716 ),
 ( #31646, #60536, #2309 ),
 ( #53412, #37342, #60078 ),
 ( #16048, #45355, #74257 ),
 ( #88465, #88915, #30246 ) ),
 .UNSPECIFIED., .F., .F., .F. ) 
 B_SPLINE_SURFACE_WITH_KNOTS ( ( 4, 2, 2, 2, 4 ),
 ( 3, 3 ),
 ( 3.665191429188113137, 3.926990816987257382, 4.188790204786401183, 4.450589592585545873, 4.712388980384689674 ),
 ( 0.000000000000000000, 1.000000000000000000 ),
 .UNSPECIFIED. ) 
 GEOMETRIC_REPRESENTATION_ITEM ( )  RATIONAL_B_SPLINE_SURFACE ( (
 ( 1.000000000000000000, 0.7905694150420956579, 1.000000000000000000),
 ( 1.000000000000000000, 0.8144940228940678040, 1.000000000000000000),
 ( 1.000000000000000000, 0.8408337462336906709, 1.000000000000000000),
 ( 1.000000000000000000, 0.8912170613351929616, 1.000000000000000000),
 ( 1.000000000000000000, 0.9152160855742275114, 1.000000000000000000),
 ( 1.000000000000000000, 0.9556126078127453738, 1.000000000000000000),
 ( 1.000000000000000000, 0.9720148405105977218, 1.000000000000000000),
 ( 1.000000000000000000, 0.9942062568699685521, 1.000000000000000000),
 ( 1.000000000000000000, 1.000000000000000000, 1.000000000000000000),
 ( 1.000000000000000000, 1.000000000000000000, 1.000000000000000000) ) ) 
 REPRESENTATION_ITEM ( '' )  SURFACE ( )  );
#43320=DIRECTION ( 'NONE',  ( 1.000000000000000000, 0.000000000000000000, 0.000000000000000000 ) ) ;
#43329=EDGE_CURVE ( 'NONE', #8082, #63051, #11152, .T. ) ;
#43336=CARTESIAN_POINT ( 'NONE',  ( 208.6466510127238507, 37.28161665985707884, 12.02378101520594100 ) ) ;
#43350=EDGE_CURVE ( 'NONE', #50260, #33465, #17182, .T. ) ;
#43374=DIRECTION ( 'NONE',  ( -0.000000000000000000, 1.000000000000000000, 0.000000000000000000 ) ) ;
#43388=ORIENTED_EDGE ( 'NONE', *, *, #77420, .F. ) ;
#43390=DIRECTION ( 'NONE',  ( -1.000000000000000000, 0.000000000000000000, 0.000000000000000000 ) ) ;
#43398=CARTESIAN_POINT ( 'NONE',  ( 200.2349812190172713, 66.43136063442170780, -7.741079165001072404 ) ) ;
#43400=CARTESIAN_POINT ( 'NONE',  ( 199.0061125298537377, 275.0000000000000568, -7.725424859374024678 ) ) ;
#43404=CARTESIAN_POINT ( 'NONE',  ( 189.9243309297870610, 275.0000000000000568, 20.22542485937349355 ) ) ;
#43406=EDGE_CURVE ( 'NONE', #56036, #68290, #41351, .T. ) ;
#43419=CARTESIAN_POINT ( 'NONE',  ( 195.5690041525305105, 26.62290662055165669, 13.81123227693192135 ) ) ;
#43433=DIRECTION ( 'NONE',  ( -0.000000000000000000, -0.000000000000000000, 1.000000000000000000 ) ) ;
#43436=CARTESIAN_POINT ( 'NONE',  ( 209.1374487190023501, 30.94653725228601715, 12.00000000000000000 ) ) ;
#43442=CARTESIAN_POINT ( 'NONE',  ( 196.0351550650565002, 41.34106363718652233, 11.96389409883856381 ) ) ;
#43445=CARTESIAN_POINT ( 'NONE',  ( 156.4851178187871312, 15.00000000000000000, 7.000000000000000888 ) ) ;
#43460=CARTESIAN_POINT ( 'NONE',  ( 152.9410204041312795, 20.82809642979767872, 8.928152258827880772 ) ) ;
#43462=FACE_OUTER_BOUND ( 'NONE', #49691, .T. ) ;
#43472=EDGE_LOOP ( 'NONE', ( #55575, #68637, #35121, #53128, #16688 ) ) ;
#43473=CARTESIAN_POINT ( 'NONE',  ( 195.0026807809657612, 40.76696999206299665, 13.61341101255641206 ) ) ;
#43478=EDGE_CURVE ( 'NONE', #72750, #1023, #40164, .T. ) ;
#43486=CARTESIAN_POINT ( 'NONE',  ( 165.2494399300530290, 8.542400036368780647, 25.74970488511327815 ) ) ;
#43498=ORIENTED_EDGE ( 'NONE', *, *, #32642, .F. ) ;
#43522=ORIENTED_EDGE ( 'NONE', *, *, #54191, .T. ) ;
#43550=CARTESIAN_POINT ( 'NONE',  ( 200.7065524281625812, 64.16053070461664731, 8.800381594953616826 ) ) ;
#43558=FACE_OUTER_BOUND ( 'NONE', #15507, .T. ) ;
#43561=DIRECTION ( 'NONE',  ( 0.000000000000000000, 0.000000000000000000, 1.000000000000000000 ) ) ;
#43562=DIRECTION ( 'NONE',  ( -0.4999999999999951705, -0.8660254037844413721, 0.000000000000000000 ) ) ;
#43571=ORIENTED_EDGE ( 'NONE', *, *, #52823, .F. ) ;
#43572=LINE ( 'NONE', #35559, #61973 ) ;
#43574=DIRECTION ( 'NONE',  ( 1.000000000000000000, 0.000000000000000000, 0.000000000000000000 ) ) ;
#43586=CARTESIAN_POINT ( 'NONE',  ( 210.3152560301384142, 38.32590481451375553, 9.000000000000001776 ) ) ;
#43587=EDGE_CURVE ( 'NONE', #52690, #29052, #26232, .T. ) ;
#43590=AXIS2_PLACEMENT_3D ( 'NONE', #42173, #28466, #36029 ) ;
#43600=EDGE_LOOP ( 'NONE', ( #14048, #53166, #44308, #33846 ) ) ;
#43626=FACE_OUTER_BOUND ( 'NONE', #51024, .T. ) ;
#43641=EDGE_CURVE ( 'NONE', #50260, #65076, #88838, .T. ) ;
#43653=CIRCLE ( 'NONE', #26970, 4.025000000000000355 ) ;
#43654=DIRECTION ( 'NONE',  ( -0.9531768234071980039, 0.3024135303179465994, 0.000000000000000000 ) ) ;
#43665=CARTESIAN_POINT ( 'NONE',  ( 208.9116897969394984, 35.81612620979493755, 14.28025116719392074 ) ) ;
#43666=CARTESIAN_POINT ( 'NONE',  ( 138.6539576904058606, 275.0000000000000568, -10.49999999999999822 ) ) ;
#43691=CARTESIAN_POINT ( 'NONE',  ( 199.3264250992830569, 299.0883425075165292, -6.145502011509054618 ) ) ;
#43694=FACE_OUTER_BOUND ( 'NONE', #77824, .T. ) ;
#43709=ORIENTED_EDGE ( 'NONE', *, *, #17514, .T. ) ;
#43712=VERTEX_POINT ( 'NONE', #4088 ) ;
#43719=AXIS2_PLACEMENT_3D ( 'NONE', #27136, #75917, #18161 ) ;
#43730=EDGE_LOOP ( 'NONE', ( #73569, #37230, #68179, #91880, #45925, #10736 ) ) ;
#43737=ORIENTED_EDGE ( 'NONE', *, *, #13861, .F. ) ;
#43740=VERTEX_POINT ( 'NONE', #32027 ) ;
#43749=CARTESIAN_POINT ( 'NONE',  ( 199.0061125298537377, 250.0000000000000568, -7.725424859374024678 ) ) ;
#43760=EDGE_CURVE ( 'NONE', #44986, #71244, #33810, .T. ) ;
#43762=CARTESIAN_POINT ( 'NONE',  ( 155.8658175007603859, 19.96629232096135098, 14.32310887264949528 ) ) ;
#43765=CARTESIAN_POINT ( 'NONE',  ( 152.4536156746142410, 129.7208004331680797, 12.50000000000000000 ) ) ;
#43768=CARTESIAN_POINT ( 'NONE',  ( 165.2494399300530290, 8.542400036368780647, 9.000000000000001776 ) ) ;
#43772=CARTESIAN_POINT ( 'NONE',  ( 209.8595557040737845, 37.94592279361958731, 12.09245862095555601 ) ) ;
#43816=ADVANCED_FACE ( 'NONE', ( #53810 ), #82678, .T. ) ;
#43824=CARTESIAN_POINT ( 'NONE',  ( 175.2296996224750103, 128.0000000000000568, 0.000000000000000000 ) ) ;
#43839=DIRECTION ( 'NONE',  ( -0.000000000000000000, -1.000000000000000000, -0.000000000000000000 ) ) ;
#43840=CARTESIAN_POINT ( 'NONE',  ( 196.7820920054853957, 24.98056201567221635, 13.24702896642047278 ) ) ;
#43842=EDGE_CURVE ( 'NONE', #77289, #90976, #52627, .T. ) ;
#43843=AXIS2_PLACEMENT_3D ( 'NONE', #21815, #50690, #56885 ) ;
#43849=CARTESIAN_POINT ( 'NONE',  ( 208.6388168579736089, 27.72533456986103317, 12.02378101520651299 ) ) ;
#43850=DIRECTION ( 'NONE',  ( -0.8195702660916324156, 0.000000000000000000, -0.5729786897769331144 ) ) ;
#43855=ORIENTED_EDGE ( 'NONE', *, *, #84181, .F. ) ;
#43859=ADVANCED_FACE ( 'NONE', ( #85490 ), #56640, .T. ) ;
#43870=CARTESIAN_POINT ( 'NONE',  ( 195.7296518112975718, 19.56734160438314873, 12.91086771431476699 ) ) ;
#43885=CARTESIAN_POINT ( 'NONE',  ( 175.2296996224750103, 140.2072866198470251, 0.000000000000000000 ) ) ;
#43907=AXIS2_PLACEMENT_3D ( 'NONE', #34503, #7030, #28801 ) ;
#43910=ORIENTED_EDGE ( 'NONE', *, *, #49297, .F. ) ;
#43911=DIRECTION ( 'NONE',  ( -0.000000000000000000, -1.000000000000000000, -0.000000000000000000 ) ) ;
#43913=CARTESIAN_POINT ( 'NONE',  ( 199.0061125298537377, 275.0000000000000568, -12.72542485937401580 ) ) ;
#43923=VERTEX_POINT ( 'NONE', #5500 ) ;
#43924=CYLINDRICAL_SURFACE ( 'NONE', #27441, 3.000000000000007994 ) ;
#43934=CARTESIAN_POINT ( 'NONE',  ( 197.4836817735085219, 42.27872732282707346, 11.66666666666666785 ) ) ;
#43956=CARTESIAN_POINT ( 'NONE',  ( 196.7806748523260012, 250.0000000000000568, -12.67104836398113932 ) ) ;
#43969=ORIENTED_EDGE ( 'NONE', *, *, #21572, .T. ) ;
#43971=LINE ( 'NONE', #21284, #539 ) ;
#43976=EDGE_CURVE ( 'NONE', #13568, #64042, #46547, .T. ) ;
#43977=EDGE_CURVE ( 'NONE', #91341, #86001, #78355, .T. ) ;
#43985=VECTOR ( 'NONE', #52646, 1000.000000000000000 ) ;
#43990=CARTESIAN_POINT ( 'NONE',  ( 164.5961120329530161, 215.0000000000000568, 23.14243616685809002 ) ) ;
#44015=CARTESIAN_POINT ( 'NONE',  ( 196.1963538710215857, 305.7026273589066250, -40.00000000000000711 ) ) ;
#44024=VERTEX_POINT ( 'NONE', #13538 ) ;
#44025=DIRECTION ( 'NONE',  ( 0.000000000000000000, 1.000000000000000000, -0.000000000000000000 ) ) ;
#44037=ORIENTED_EDGE ( 'NONE', *, *, #23779, .T. ) ;
#44042=CARTESIAN_POINT ( 'NONE',  ( 140.6539576904058606, 132.0000000000000568, 12.50000000000000000 ) ) ;
#44054=ORIENTED_EDGE ( 'NONE', *, *, #72628, .T. ) ;
#44080=CARTESIAN_POINT ( 'NONE',  ( 195.3232612940492174, 24.75642484911453423, 13.12563582463413248 ) ) ;
#44105=CYLINDRICAL_SURFACE ( 'NONE', #68611, 0.5000000000000043299 ) ;
#44106=TOROIDAL_SURFACE ( 'NONE', #21489, 1.000000000000000000, 0.5000000000000000000 ) ;
#44108=CIRCLE ( 'NONE', #21492, 0.5000000000000004441 ) ;
#44116=CARTESIAN_POINT ( 'NONE',  ( 170.8178014930282700, 8.542400036368780647, 25.74970488511327815 ) ) ;
#44132=CARTESIAN_POINT ( 'NONE',  ( 156.4947056272797852, 21.00000000000000000, -15.00000000000000000 ) ) ;
#44146=DIRECTION ( 'NONE',  ( -1.000000000000000000, 0.000000000000000000, 0.000000000000000000 ) ) ;
#44149=DIRECTION ( 'NONE',  ( -0.01818181818182024526, -0.000000000000000000, -0.9998346970812742596 ) ) ;
#44158=EDGE_CURVE ( 'NONE', #10842, #23364, #77453, .T. ) ;
#44168=VERTEX_POINT ( 'NONE', #5022 ) ;
#44177=AXIS2_PLACEMENT_3D ( 'NONE', #85905, #49471, #71739 ) ;
#44181=TOROIDAL_SURFACE ( 'NONE', #45716, 1.000000000000000000, 0.5000000000000000000 ) ;
#44210=FACE_OUTER_BOUND ( 'NONE', #32450, .T. ) ;
#44215=CARTESIAN_POINT ( 'NONE',  ( 165.2494399300530290, 8.542400036368780647, 10.00000000000000000 ) ) ;
#44221=LINE ( 'NONE', #38041, #27716 ) ;
#44224=CARTESIAN_POINT ( 'NONE',  ( 204.6539576904058606, 300.0210572133868823, -59.00000000000003553 ) ) ;
#44226=CARTESIAN_POINT ( 'NONE',  ( 154.9065949031762841, 18.65395765032815234, -9.525636664970921430 ) ) ;
#44229=FACE_OUTER_BOUND ( 'NONE', #71699, .T. ) ;
#44242=VECTOR ( 'NONE', #62643, 1000.000000000000000 ) ;
#44249=VECTOR ( 'NONE', #73494, 1000.000000000000000 ) ;
#44253=CIRCLE ( 'NONE', #42709, 10.55076157886938937 ) ;
#44255=PRODUCT ( 'Pneumatic Power Actuating Cylinder', 'Pneumatic Power Actuating Cylinder', '', ( #76689 ) ) ;
#44269=EDGE_CURVE ( 'NONE', #67382, #37492, #84074, .T. ) ;
#44270=LINE ( 'NONE', #8299, #81687 ) ;
#44275=EDGE_CURVE ( 'NONE', #4269, #69256, #34373, .T. ) ;
#44278=ADVANCED_FACE ( 'NONE', ( #63278 ), #39117, .F. ) ;
#44308=ORIENTED_EDGE ( 'NONE', *, *, #81073, .F. ) ;
#44312=AXIS2_PLACEMENT_3D ( 'NONE', #91971, #64080, #44468 ) ;
#44317=DIRECTION ( 'NONE',  ( -0.9693563597868428694, -0.2456588035076310295, 1.704600374100243061E-15 ) ) ;
#44318=CARTESIAN_POINT ( 'NONE',  ( 140.6539576904058606, 130.0000000000000568, 12.50000000000000000 ) ) ;
#44320=VECTOR ( 'NONE', #21210, 1000.000000000000000 ) ;
#44324=VERTEX_POINT ( 'NONE', #60709 ) ;
#44325=CARTESIAN_POINT ( 'NONE',  ( 197.7225753183262782, 40.74748806490614328, 10.04280106464628020 ) ) ;
#44337=CIRCLE ( 'NONE', #85175, 2.000000000000007105 ) ;
#44340=CARTESIAN_POINT ( 'NONE',  ( 219.8344101925596021, 35.72494958537217968, -9.000000000000001776 ) ) ;
#44342=AXIS2_PLACEMENT_3D ( 'NONE', #68152, #61978, #75711 ) ;
#44349=DIRECTION ( 'NONE',  ( 0.5370370370370424196, -2.395818010342801312E-14, -0.8435586647355799439 ) ) ;
#44357=DIRECTION ( 'NONE',  ( 0.5000000000000032196, -0.8660254037844368202, 0.000000000000000000 ) ) ;
#44363=DIRECTION ( 'NONE',  ( -0.000000000000000000, -1.000000000000000000, -0.000000000000000000 ) ) ;
#44374=CIRCLE ( 'NONE', #35337, 24.00000000000000355 ) ;
#44377=ADVANCED_FACE ( 'NONE', ( #89086 ), #67353, .T. ) ;
#44395=CARTESIAN_POINT ( 'NONE',  ( 152.4536156746142410, 275.0000000000000568, 14.50000000000000000 ) ) ;
#44408=CARTESIAN_POINT ( 'NONE',  ( 207.8064396648212551, 36.74001737686529623, 13.57731244650625690 ) ) ;
#44420=EDGE_LOOP ( 'NONE', ( #31838, #92742, #32108, #13903 ) ) ;
#44426=DIRECTION ( 'NONE',  ( 0.6522365350567651543, -0.2069344830099842103, -0.7292226148979034095 ) ) ;
#44438=CARTESIAN_POINT ( 'NONE',  ( 199.8304385318961351, 66.96291204605094549, -8.111402028797257913 ) ) ;
#44442=VERTEX_POINT ( 'NONE', #74917 ) ;
#44443=ORIENTED_EDGE ( 'NONE', *, *, #56330, .T. ) ;
#44444=CARTESIAN_POINT ( 'NONE',  ( 196.1511317126956158, 42.06348744092182557, 13.68688499713156403 ) ) ;
#44468=DIRECTION ( 'NONE',  ( 0.000000000000000000, 0.000000000000000000, 1.000000000000000000 ) ) ;
#44470=CIRCLE ( 'NONE', #698, 5.568361562975243650 ) ;
#44477=AXIS2_PLACEMENT_3D ( 'NONE', #53060, #75318, #3338 ) ;
#44485=VECTOR ( 'NONE', #73522, 1000.000000000000000 ) ;
#44488=PLANE ( 'NONE',  #92941 ) ;
#44497=CARTESIAN_POINT ( 'NONE',  ( 202.4403316624510580, 63.53362652955771495, -6.999999999998341771 ) ) ;
#44516=DIRECTION ( 'NONE',  ( 0.000000000000000000, 1.000000000000000000, 0.000000000000000000 ) ) ;
#44517=ADVANCED_FACE ( 'NONE', ( #3876 ), #84324, .F. ) ;
#44530=CIRCLE ( 'NONE', #24879, 25.00000000000000355 ) ;
#44535=ORIENTED_EDGE ( 'NONE', *, *, #57901, .T. ) ;
#44542=LINE ( 'NONE', #73445, #18871 ) ;
#44554=DIRECTION ( 'NONE',  ( 0.000000000000000000, 0.000000000000000000, -1.000000000000000000 ) ) ;
#44563=DIRECTION ( 'NONE',  ( 0.6056179655966478226, -0.7957555401921982963, 0.000000000000000000 ) ) ;
#44578=CARTESIAN_POINT ( 'NONE',  ( 193.5162140859150668, 250.0000000000000568, 17.51463615629760895 ) ) ;
#44584=FACE_OUTER_BOUND ( 'NONE', #20592, .T. ) ;
#44586=CARTESIAN_POINT ( 'NONE',  ( 199.1087447750284980, 64.61450673763175701, -10.46317447812566570 ) ) ;
#44589=CARTESIAN_POINT ( 'NONE',  ( 195.5825507613122056, 25.45032227799513791, 14.51846093667993465 ) ) ;
#44600=EDGE_CURVE ( 'NONE', #43712, #35960, #91897, .T. ) ;
#44601=ORIENTED_EDGE ( 'NONE', *, *, #36488, .T. ) ;
#44605=CARTESIAN_POINT ( 'NONE',  ( 195.6515579107327483, 26.26913368994353348, 14.74629060332673980 ) ) ;
#44618=CARTESIAN_POINT ( 'NONE',  ( 169.7306087885279169, 249.5000000000000568, -24.89999999999998792 ) ) ;
#44620=CLOSED_SHELL ( 'NONE', ( #16198, #13204, #69298, #11489, #49402, #51333, #56872, #91623, #29850, #42271, #64220, #75500, #30698, #33856, #75088, #30940, #83301, #68366, #75852, #733, #73637, #81893, #24291, #84393, #8068, #75445, #19071 ) ) ;
#44623=CARTESIAN_POINT ( 'NONE',  ( 213.7238915819278589, 32.98517505407394168, 12.09245862095555601 ) ) ;
#44639=ORIENTED_EDGE ( 'NONE', *, *, #19673, .F. ) ;
#44642=EDGE_CURVE ( 'NONE', #74853, #45543, #69669, .T. ) ;
#44650=ORIENTED_EDGE ( 'NONE', *, *, #266, .T. ) ;
#44661=ORIENTED_EDGE ( 'NONE', *, *, #1524, .F. ) ;
#44669=DIRECTION ( 'NONE',  ( 1.000000000000000000, -0.000000000000000000, -0.000000000000000000 ) ) ;
#44682=CARTESIAN_POINT ( 'NONE',  ( 208.4306832106271088, -74.55766379199613425, 0.000000000000000000 ) ) ;
#44685=CIRCLE ( 'NONE', #23538, 11.60392986742922439 ) ;
#44688=DIRECTION ( 'NONE',  ( 0.000000000000000000, 0.000000000000000000, 1.000000000000000000 ) ) ;
#44694=CARTESIAN_POINT ( 'NONE',  ( 155.2899061951533213, 19.82375796246816435, 13.63853015639329413 ) ) ;
#44697=CARTESIAN_POINT ( 'NONE',  ( 151.6966102050380414, 129.9764884006976899, 12.50000000000000178 ) ) ;
#44699=CARTESIAN_POINT ( 'NONE',  ( 154.6019620322547041, 19.02489598991821751, -11.88315578651767979 ) ) ;
#44701=DIRECTION ( 'NONE',  ( -0.9531768234071980039, 0.3024135303179465994, 0.000000000000000000 ) ) ;
#44705=CARTESIAN_POINT ( 'NONE',  ( 180.2297292323760303, 215.0000000000001705, -24.97289011430694217 ) ) ;
#44718=CARTESIAN_POINT ( 'NONE',  ( 201.2104617360081704, 60.19600395700749829, 9.000000000000001776 ) ) ;
#44722=CARTESIAN_POINT ( 'NONE',  ( 156.4947056272797852, 20.00000000000000000, -15.00000000000000000 ) ) ;
#44755=EDGE_CURVE ( 'NONE', #13111, #41136, #10252, .T. ) ;
#44775=ORIENTED_EDGE ( 'NONE', *, *, #58549, .T. ) ;
#44776=DIRECTION ( 'NONE',  ( -1.000000000000000000, 0.000000000000000000, 0.000000000000000000 ) ) ;
#44782=FACE_OUTER_BOUND ( 'NONE', #32173, .T. ) ;
#44787=ORIENTED_EDGE ( 'NONE', *, *, #80099, .F. ) ;
#44788=DIRECTION ( 'NONE',  ( -0.000000000000000000, -0.000000000000000000, 1.000000000000000000 ) ) ;
#44799=EDGE_CURVE ( 'NONE', #86758, #70448, #69538, .T. ) ;
#44800=EDGE_CURVE ( 'NONE', #4038, #52800, #19019, .T. ) ;
#44801=CARTESIAN_POINT ( 'NONE',  ( 152.4771702478159909, 19.90416625621075752, 8.234418254360116762 ) ) ;
#44810=CARTESIAN_POINT ( 'NONE',  ( 197.1123855246548828, 18.41506350946109194, 10.91506350946109016 ) ) ;
#44817=CARTESIAN_POINT ( 'NONE',  ( 189.4188515237862589, 293.9636489450775798, -40.00000000000000711 ) ) ;
#44839=VERTEX_POINT ( 'NONE', #26102 ) ;
#44840=CARTESIAN_POINT ( 'NONE',  ( 197.0996632504151762, 71.85522536017060702, 12.14506853158196265 ) ) ;
#44851=EDGE_LOOP ( 'NONE', ( #91719, #32832, #13700, #34907, #25675 ) ) ;
#44852=DIRECTION ( 'NONE',  ( 0.000000000000000000, 0.000000000000000000, -1.000000000000000000 ) ) ;
#44884=DIRECTION ( 'NONE',  ( 0.000000000000000000, 0.000000000000000000, 1.000000000000000000 ) ) ;
#44885=LINE ( 'NONE', #66234, #85002 ) ;
#44898=ORIENTED_EDGE ( 'NONE', *, *, #24425, .T. ) ;
#44899=ORIENTED_EDGE ( 'NONE', *, *, #34695, .F. ) ;
#44900=CARTESIAN_POINT ( 'NONE',  ( 195.0934829612641295, 39.77032864624461439, 15.17998222329788760 ) ) ;
#44915=EDGE_CURVE ( 'NONE', #65773, #87468, #49609, .T. ) ;
#44924=CARTESIAN_POINT ( 'NONE',  ( 201.2104617360081704, 25.32700003806615996, 9.000000000000001776 ) ) ;
#44928=DIRECTION ( 'NONE',  ( 0.000000000000000000, 0.000000000000000000, 1.000000000000000000 ) ) ;
#44930=LINE ( 'NONE', #10345, #73221 ) ;
#44940=CARTESIAN_POINT ( 'NONE',  ( 154.9842916688210153, 128.0000000000000568, 12.88888888888890349 ) ) ;
#44950=VERTEX_POINT ( 'NONE', #47873 ) ;
#44954=DIRECTION ( 'NONE',  ( 1.000000000000000000, 0.000000000000000000, -0.000000000000000000 ) ) ;
#44963=ORIENTED_EDGE ( 'NONE', *, *, #8073, .F. ) ;
#44967=CARTESIAN_POINT ( 'NONE',  ( 175.2296996224750103, 20.99999999999998934, 24.00000000000000355 ) ) ;
#44978=ORIENTED_EDGE ( 'NONE', *, *, #29709, .T. ) ;
#44981=EDGE_CURVE ( 'NONE', #13368, #3752, #17563, .T. ) ;
#44986=VERTEX_POINT ( 'NONE', #26585 ) ;
#44993=DIRECTION ( 'NONE',  ( -1.000000000000000000, 0.000000000000000000, 0.000000000000000000 ) ) ;
#45004=ORIENTED_EDGE ( 'NONE', *, *, #92815, .T. ) ;
#45005=CYLINDRICAL_SURFACE ( 'NONE', #29266, 1.999999999999988454 ) ;
#45009=EDGE_CURVE ( 'NONE', #71244, #17165, #55475, .T. ) ;
#45015=CARTESIAN_POINT ( 'NONE',  ( 208.3080460680526755, 36.52560914003142045, 14.78771946819801109 ) ) ;
#45029=CARTESIAN_POINT ( 'NONE',  ( 196.3996634987102539, 25.59933695287653777, 11.39947427447970441 ) ) ;
#45036=CARTESIAN_POINT ( 'NONE',  ( 196.1963538710216994, 282.2246705312485915, -40.00000000000000711 ) ) ;
#45040=ADVANCED_FACE ( 'NONE', ( #85279 ), #84792, .F. ) ;
#45050=AXIS2_PLACEMENT_3D ( 'NONE', #58291, #21352, #64947 ) ;
#45051=B_SPLINE_CURVE_WITH_KNOTS ( 'NONE', 3,
 ( #16485, #40104, #32574, #60062, #67161, #53396, #11250, #25001 ),
 .UNSPECIFIED., .F., .F.,
 ( 4, 2, 2, 4 ),
 ( 0.000000000000000000, 0.004397459120518200718, 0.006596188680777302811, 0.008794918241036404905 ),
 .UNSPECIFIED. ) ;
#45052=ORIENTED_EDGE ( 'NONE', *, *, #203, .F. ) ;
#45053=DIRECTION ( 'NONE',  ( 0.000000000000000000, 0.000000000000000000, -1.000000000000000000 ) ) ;
#45056=CARTESIAN_POINT ( 'NONE',  ( 197.1933712184921603, 24.89666632552609826, 12.64285714285712992 ) ) ;
#45068=CARTESIAN_POINT ( 'NONE',  ( 157.7437329832453088, 18.12362412296306502, 11.08836552221218419 ) ) ;
#45071=DIRECTION ( 'NONE',  ( -0.000000000000000000, -0.000000000000000000, -1.000000000000000000 ) ) ;
#45087=VERTEX_POINT ( 'NONE', #56419 ) ;
#45107=ORIENTED_EDGE ( 'NONE', *, *, #13517, .T. ) ;
#45115=CARTESIAN_POINT ( 'NONE',  ( 159.4572718888341285, 15.57755555264331271, 9.020884447463151545 ) ) ;
#45118=ORIENTED_EDGE ( 'NONE', *, *, #42879, .T. ) ;
#45119=ADVANCED_FACE ( 'NONE', ( #86202 ), #20889, .T. ) ;
#45121=AXIS2_PLACEMENT_3D ( 'NONE', #92092, #41899, #56623 ) ;
#45136=PLANE ( 'NONE',  #23300 ) ;
#45139=EDGE_CURVE ( 'NONE', #25330, #31000, #79826, .T. ) ;
#45140=ADVANCED_FACE ( 'NONE', ( #6219 ), #20886, .T. ) ;
#45152=CARTESIAN_POINT ( 'NONE',  ( 175.2296996224749250, 250.0000000000000568, -24.99999999999999289 ) ) ;
#45156=CARTESIAN_POINT ( 'NONE',  ( 199.0143093133017373, 16.83012701892205598, -10.00000000000000000 ) ) ;
#45187=FACE_OUTER_BOUND ( 'NONE', #60970, .T. ) ;
#45199=ORIENTED_EDGE ( 'NONE', *, *, #80212, .T. ) ;
#45203=ADVANCED_FACE ( 'NONE', ( #47 ), #51156, .T. ) ;
#45206=B_SPLINE_CURVE_WITH_KNOTS ( 'NONE', 3,
 ( #81685, #9728, #16834, #38607, #67511, #2641, #59947, #23935, #42542, #86099, #91798, #20326 ),
 .UNSPECIFIED., .F., .F.,
 ( 4, 2, 2, 2, 2, 4 ),
 ( 0.000000000000000000, 0.002337776193942625591, 0.004675552387885251182, 0.007013328581827875906, 0.008182216678799194773, 0.009351104775770512773 ),
 .UNSPECIFIED. ) ;
#45209=DIRECTION ( 'NONE',  ( 0.000000000000000000, 0.000000000000000000, 1.000000000000000000 ) ) ;
#45222=ORIENTED_EDGE ( 'NONE', *, *, #31573, .F. ) ;
#45223=LINE ( 'NONE', #66124, #43210 ) ;
#45230=CARTESIAN_POINT ( 'NONE',  ( 159.4851178187871312, 3.000000000000000000, 10.00000000000000000 ) ) ;
#45235=ORIENTED_EDGE ( 'NONE', *, *, #86265, .F. ) ;
#45236=LINE ( 'NONE', #38136, #21773 ) ;
#45250=FACE_OUTER_BOUND ( 'NONE', #46570, .T. ) ;
#45266=ADVANCED_FACE ( 'NONE', ( #29861 ), #28468, .F. ) ;
#45270=CARTESIAN_POINT ( 'NONE',  ( 200.2349812190172713, 66.43136063442170780, -7.741079165001072404 ) ) ;
#45294=CARTESIAN_POINT ( 'NONE',  ( 197.3688982409817072, 70.32660332368789113, 11.79193394828015151 ) ) ;
#45305=ORIENTED_EDGE ( 'NONE', *, *, #65063, .T. ) ;
#45306=CARTESIAN_POINT ( 'NONE',  ( 196.6738303916082202, 40.98441723029247186, 12.63306117497344516 ) ) ;
#45313=AXIS2_PLACEMENT_3D ( 'NONE', #6204, #7140, #36013 ) ;
#45317=DIRECTION ( 'NONE',  ( 0.000000000000000000, -0.000000000000000000, 1.000000000000000000 ) ) ;
#45319=TOROIDAL_SURFACE ( 'NONE', #33309, 3.342139515347635204, 0.5000000000000000000 ) ;
#45322=EDGE_LOOP ( 'NONE', ( #85559, #61687, #4318, #91194 ) ) ;
#45349=CARTESIAN_POINT ( 'NONE',  ( 207.5217838046588099, 35.61973263570791204, 14.46447120960655752 ) ) ;
#45354=ORIENTED_EDGE ( 'NONE', *, *, #49001, .F. ) ;
#45355=CARTESIAN_POINT ( 'NONE',  ( 200.7304780712264289, 15.47998366482157984, -9.999999999999360512 ) ) ;
#45368=DIRECTION ( 'NONE',  ( 0.000000000000000000, 0.000000000000000000, -1.000000000000000000 ) ) ;
#45369=CARTESIAN_POINT ( 'NONE',  ( 196.0143093133015384, 20.19615242270663913, -11.99999999999998579 ) ) ;
#45377=DIRECTION ( 'NONE',  ( 0.000000000000000000, 1.000000000000000000, 0.000000000000000000 ) ) ;
#45381=CARTESIAN_POINT ( 'NONE',  ( 201.2104617360081704, 25.32700003806617772, 10.49999999999999822 ) ) ;
#45383=AXIS2_PLACEMENT_3D ( 'NONE', #41579, #50092, #77585 ) ;
#45384=DIRECTION ( 'NONE',  ( 0.000000000000000000, 0.000000000000000000, -1.000000000000000000 ) ) ;
#45389=AXIS2_PLACEMENT_3D ( 'NONE', #7573, #36458, #65373 ) ;
#45395=ADVANCED_FACE ( 'NONE', ( #7155 ), #51094, .T. ) ;
#45397=CARTESIAN_POINT ( 'NONE',  ( 206.8859853974219618, 30.07047180831808220, 15.00000000000000000 ) ) ;
#45407=ORIENTED_EDGE ( 'NONE', *, *, #35371, .T. ) ;
#45411=DIRECTION ( 'NONE',  ( 0.000000000000000000, 0.000000000000000000, 1.000000000000000000 ) ) ;
#45425=CARTESIAN_POINT ( 'NONE',  ( 196.0143093133015384, 73.40565171261609123, 11.99999999999998757 ) ) ;
#45428=DIRECTION ( 'NONE',  ( -0.000000000000000000, -1.000000000000000000, -0.000000000000000000 ) ) ;
#45431=EDGE_CURVE ( 'NONE', #30016, #15179, #87522, .T. ) ;
#45437=ORIENTED_EDGE ( 'NONE', *, *, #47255, .F. ) ;
#45446=ORIENTED_EDGE ( 'NONE', *, *, #3450, .T. ) ;
#45448=TOROIDAL_SURFACE ( 'NONE', #16676, 2.500000000000000000, 0.5000000000000000000 ) ;
#45454=DIRECTION ( 'NONE',  ( 0.2456588035076220367, -0.9693563597868450898, 0.000000000000000000 ) ) ;
#45465=ORIENTED_EDGE ( 'NONE', *, *, #87897, .F. ) ;
#45475=FACE_OUTER_BOUND ( 'NONE', #60016, .T. ) ;
#45485=CARTESIAN_POINT ( 'NONE',  ( 160.6539576904058606, 293.9636489450775230, 7.999911143031724237 ) ) ;
#45487=CARTESIAN_POINT ( 'NONE',  ( 197.2824889331299687, 25.87897341259697370, 12.13121414925255337 ) ) ;
#45493=CARTESIAN_POINT ( 'NONE',  ( 175.2296996224749250, 275.0000000000000568, -24.99999999999999289 ) ) ;
#45498=CARTESIAN_POINT ( 'NONE',  ( 169.7306087885279453, 250.5000000000000568, -24.89999999999999147 ) ) ;
#45508=EDGE_LOOP ( 'NONE', ( #28838, #91941, #91513, #52660 ) ) ;
#45525=CARTESIAN_POINT ( 'NONE',  ( 159.3464669004306984, 15.95758591462588249, 10.08665682397413299 ) ) ;
#45526=EDGE_CURVE ( 'NONE', #71459, #9221, #36487, .T. ) ;
#45543=VERTEX_POINT ( 'NONE', #72943 ) ;
#45546=ORIENTED_EDGE ( 'NONE', *, *, #24741, .T. ) ;
#45549=ADVANCED_FACE ( 'NONE', ( #42647 ), #71564, .F. ) ;
#45557=ORIENTED_EDGE ( 'NONE', *, *, #76503, .T. ) ;
#45567=EDGE_LOOP ( 'NONE', ( #76448, #51478 ) ) ;
#45574=ORIENTED_EDGE ( 'NONE', *, *, #9361, .T. ) ;
#45575=DIRECTION ( 'NONE',  ( -1.000000000000000000, 2.441433246481030855E-15, 0.000000000000000000 ) ) ;
#45579=EDGE_LOOP ( 'NONE', ( #92238, #72496, #17179, #13427 ) ) ;
#45584=VECTOR ( 'NONE', #14073, 1000.000000000000000 ) ;
#45588=CIRCLE ( 'NONE', #81890, 9.103929867429224387 ) ;
#45596=ORIENTED_EDGE ( 'NONE', *, *, #91565, .T. ) ;
#45597=AXIS2_PLACEMENT_3D ( 'NONE', #62801, #32949, #89759 ) ;
#45600=DIRECTION ( 'NONE',  ( 0.000000000000000000, 1.000000000000000000, 0.000000000000000000 ) ) ;
#45606=LINE ( 'NONE', #66949, #86623 ) ;
#45607=CARTESIAN_POINT ( 'NONE',  ( 196.2522475779649369, 20.68155234470936676, 13.54449592192992569 ) ) ;
#45612=LINE ( 'NONE', #59396, #92439 ) ;
#45629=CARTESIAN_POINT ( 'NONE',  ( 200.1126601882106968, 250.5000000000000568, -2.416251949619912409 ) ) ;
#45647=EDGE_CURVE ( 'NONE', #33225, #79497, #93529, .T. ) ;
#45651=FACE_OUTER_BOUND ( 'NONE', #70902, .T. ) ;
#45652=CIRCLE ( 'NONE', #56307, 24.00000000000000355 ) ;
#45663=AXIS2_PLACEMENT_3D ( 'NONE', #86279, #29937, #80575 ) ;
#45666=VERTEX_POINT ( 'NONE', #22734 ) ;
#45671=EDGE_CURVE ( 'NONE', #19571, #25512, #45885, .T. ) ;
#45672=EDGE_CURVE ( 'NONE', #50719, #15573, #91972, .T. ) ;
#45690=ORIENTED_EDGE ( 'NONE', *, *, #58679, .F. ) ;
#45691=CARTESIAN_POINT ( 'NONE',  ( 188.7149167944524493, 8.542400036368780647, 10.00000000000000178 ) ) ;
#45703=DIRECTION ( 'NONE',  ( 0.000000000000000000, 0.000000000000000000, 1.000000000000000000 ) ) ;
#45712=AXIS2_PLACEMENT_3D ( 'NONE', #77426, #12565, #70349 ) ;
#45716=AXIS2_PLACEMENT_3D ( 'NONE', #2232, #24454, #60002 ) ;
#45720=FACE_OUTER_BOUND ( 'NONE', #65284, .T. ) ;
#45722=VECTOR ( 'NONE', #35059, 1000.000000000000000 ) ;
#45730=DIRECTION ( 'NONE',  ( 0.000000000000000000, 0.000000000000000000, 1.000000000000000000 ) ) ;
#45736=DIRECTION ( 'NONE',  ( 0.000000000000000000, 0.000000000000000000, 1.000000000000000000 ) ) ;
#45739=DIRECTION ( 'NONE',  ( 2.312964634635742267E-15, 0.000000000000000000, 1.000000000000000000 ) ) ;
#45746=DIRECTION ( 'NONE',  ( 1.000000000000000000, -0.000000000000000000, -0.000000000000000000 ) ) ;
#45749=CARTESIAN_POINT ( 'NONE',  ( 154.1407330040854333, 275.0000000000000568, 13.42592592592592915 ) ) ;
#45751=( BOUNDED_CURVE ( )  B_SPLINE_CURVE ( 3, ( #91399, #26554, #24680, #39789 ),
 .UNSPECIFIED., .F., .T. ) 
 B_SPLINE_CURVE_WITH_KNOTS ( ( 4, 4 ),
 ( 3.871320309816760563, 4.712388980384689674 ),
 .UNSPECIFIED. ) 
 CURVE ( )  GEOMETRIC_REPRESENTATION_ITEM ( )  RATIONAL_B_SPLINE_CURVE ( ( 1.000000000000000000, 0.9419139527835179715, 0.9419139527835179715, 1.000000000000000000 ) ) 
 REPRESENTATION_ITEM ( '' )  );
#45760=( BOUNDED_CURVE ( )  B_SPLINE_CURVE ( 3, ( #47204, #69476, #62385, #47686 ),
 .UNSPECIFIED., .F., .F. ) 
 B_SPLINE_CURVE_WITH_KNOTS ( ( 4, 4 ),
 ( 3.141592653589793116, 4.712388980384689674 ),
 .UNSPECIFIED. ) 
 CURVE ( )  GEOMETRIC_REPRESENTATION_ITEM ( )  RATIONAL_B_SPLINE_CURVE ( ( 1.000000000000000000, 0.8047378541243649375, 0.8047378541243649375, 1.000000000000000000 ) ) 
 REPRESENTATION_ITEM ( '' )  );
#45778=CARTESIAN_POINT ( 'NONE',  ( 195.2223182338679806, 41.98397561837970215, 13.27870513978759526 ) ) ;
#45780=AXIS2_PLACEMENT_3D ( 'NONE', #86611, #21780, #13283 ) ;
#45789=CARTESIAN_POINT ( 'NONE',  ( 175.2296996224749250, 249.5000000000000568, -24.99999999999999289 ) ) ;
#45796=VECTOR ( 'NONE', #30394, 1000.000000000000000 ) ;
#45811=CARTESIAN_POINT ( 'NONE',  ( 159.4851178187871312, 3.000000000000000000, 9.000000000000001776 ) ) ;
#45816=CARTESIAN_POINT ( 'NONE',  ( 152.4536156746142410, 129.7208004331680797, 12.50000000000000000 ) ) ;
#45818=CIRCLE ( 'NONE', #64064, 3.342139515347647638 ) ;
#45826=CARTESIAN_POINT ( 'NONE',  ( 184.8939426562960193, 2.965303559109565334, -9.000000000000001776 ) ) ;
#45829=VECTOR ( 'NONE', #52532, 1000.000000000000000 ) ;
#45831=VERTEX_POINT ( 'NONE', #73867 ) ;
#45832=ORIENTED_EDGE ( 'NONE', *, *, #30385, .F. ) ;
#45833=CARTESIAN_POINT ( 'NONE',  ( 195.0811277904324186, 39.56745693038991618, 15.19607843137254477 ) ) ;
#45856=CARTESIAN_POINT ( 'NONE',  ( 153.8610353528599717, 19.40315322326054215, 11.71374297039772649 ) ) ;
#45864=AXIS2_PLACEMENT_3D ( 'NONE', #63611, #27126, #37364 ) ;
#45867=AXIS2_PLACEMENT_3D ( 'NONE', #78130, #14668, #87068 ) ;
#45873=CIRCLE ( 'NONE', #51956, 0.5000000000000004441 ) ;
#45876=DIRECTION ( 'NONE',  ( 0.000000000000000000, 0.000000000000000000, -1.000000000000000000 ) ) ;
#45885=B_SPLINE_CURVE_WITH_KNOTS ( 'NONE', 3,
 ( #59206, #30790, #61080, #17040, #23209, #16570, #89922, #73418, #25078, #67704, #2380, #45425 ),
 .UNSPECIFIED., .F., .F.,
 ( 4, 2, 2, 2, 2, 4 ),
 ( 0.000000000000000000, 0.002380535361927522270, 0.004761070723855044540, 0.007141606085782566810, 0.008331873766746348761, 0.009522141447710128978 ),
 .UNSPECIFIED. ) ;
#45887=VERTEX_POINT ( 'NONE', #88531 ) ;
#45889=AXIS2_PLACEMENT_3D ( 'NONE', #68016, #3145, #24933 ) ;
#45892=CARTESIAN_POINT ( 'NONE',  ( 169.7306087885279453, 250.5000000000000568, -24.89999999999999147 ) ) ;
#45899=AXIS2_PLACEMENT_3D ( 'NONE', #72359, #57688, #92240 ) ;
#45904=DIRECTION ( 'NONE',  ( 0.000000000000000000, 0.000000000000000000, 1.000000000000000000 ) ) ;
#45906=LINE ( 'NONE', #88984, #39039 ) ;
#45925=ORIENTED_EDGE ( 'NONE', *, *, #45647, .T. ) ;
#45927=CIRCLE ( 'NONE', #5139, 0.5000000000000000000 ) ;
#45929=B_SPLINE_CURVE_WITH_KNOTS ( 'NONE', 3,
 ( #61267, #53677, #18152, #82545, #17695, #90102, #25253, #54129 ),
 .UNSPECIFIED., .F., .F.,
 ( 4, 2, 2, 4 ),
 ( 0.000000000000000000, 0.001370196721548361165, 0.002055295082322501198, 0.002740393443096640798 ),
 .UNSPECIFIED. ) ;
#45933=CARTESIAN_POINT ( 'NONE',  ( 165.0704140682094589, 2.965303559109564890, -9.000000000000001776 ) ) ;
#45939=AXIS2_PLACEMENT_3D ( 'NONE', #82880, #46888, #39779 ) ;
#45945=ORIENTED_EDGE ( 'NONE', *, *, #25613, .T. ) ;
#45950=CIRCLE ( 'NONE', #14231, 0.5000000000000004441 ) ;
#45957=CARTESIAN_POINT ( 'NONE',  ( 207.8643778022843662, 35.72636131987241725, 15.02863188060180732 ) ) ;
#45964=CIRCLE ( 'NONE', #20311, 0.5000000000000004441 ) ;
#45971=DIRECTION ( 'NONE',  ( 1.000000000000000000, 0.000000000000000000, -0.000000000000000000 ) ) ;
#45978=EDGE_CURVE ( 'NONE', #80198, #17402, #8985, .T. ) ;
#45979=DIRECTION ( 'NONE',  ( 0.000000000000000000, 0.000000000000000000, 1.000000000000000000 ) ) ;
#45981=CARTESIAN_POINT ( 'NONE',  ( 196.0143093133017658, 19.33012701892200624, -12.49999999999967315 ) ) ;
#45985=PLANE ( 'NONE',  #59418 ) ;
#45994=ORIENTED_EDGE ( 'NONE', *, *, #17361, .T. ) ;
#45998=DIRECTION ( 'NONE',  ( -0.000000000000000000, -1.000000000000000000, -0.000000000000000000 ) ) ;
#46002=AXIS2_PLACEMENT_3D ( 'NONE', #61035, #53912, #4651 ) ;
#46011=CIRCLE ( 'NONE', #71748, 5.103083949679981579 ) ;
#46015=CARTESIAN_POINT ( 'NONE',  ( 199.2296996224750103, 68.12454877777268791, 0.000000000000000000 ) ) ;
#46017=AXIS2_PLACEMENT_3D ( 'NONE', #4608, #40563, #11710 ) ;
#46030=EDGE_LOOP ( 'NONE', ( #62204, #59342, #13492, #40912, #9704, #49632 ) ) ;
#46043=ORIENTED_EDGE ( 'NONE', *, *, #86610, .F. ) ;
#46061=CARTESIAN_POINT ( 'NONE',  ( 157.3397966316789791, 16.44589409474655639, 9.145321187104725524 ) ) ;
#46065=VERTEX_POINT ( 'NONE', #9449 ) ;
#46081=DIRECTION ( 'NONE',  ( 0.000000000000000000, 0.000000000000000000, 1.000000000000000000 ) ) ;
#46083=AXIS2_PLACEMENT_3D ( 'NONE', #1403, #52061, #22 ) ;
#46088=CARTESIAN_POINT ( 'NONE',  ( 197.5379522065468052, 250.5000000000000568, -11.97918851819044050 ) ) ;
#46092=EDGE_CURVE ( 'NONE', #90266, #50020, #60607, .T. ) ;
#46097=CARTESIAN_POINT ( 'NONE',  ( 175.2296996224750103, 275.0000000000000568, -24.00000000000000355 ) ) ;
#46114=FACE_OUTER_BOUND ( 'NONE', #82391, .T. ) ;
#46117=DIRECTION ( 'NONE',  ( -6.570707696761130958E-14, 0.000000000000000000, 1.000000000000000000 ) ) ;
#46135=CARTESIAN_POINT ( 'NONE',  ( 153.6539576904058038, 130.0000000000000568, 12.50000000000000000 ) ) ;
#46149=ORIENTED_EDGE ( 'NONE', *, *, #68345, .F. ) ;
#46175=DIRECTION ( 'NONE',  ( 0.000000000000000000, -1.000000000000000000, 0.000000000000000000 ) ) ;
#46195=DIRECTION ( 'NONE',  ( 0.000000000000000000, 0.000000000000000000, 1.000000000000000000 ) ) ;
#46205=DIRECTION ( 'NONE',  ( 0.000000000000000000, 0.000000000000000000, -1.000000000000000000 ) ) ;
#46209=EDGE_CURVE ( 'NONE', #69284, #12630, #45906, .T. ) ;
#46211=CARTESIAN_POINT ( 'NONE',  ( 209.4803090767392462, 35.69423656899339647, 14.26380412667038833 ) ) ;
#46214=FACE_OUTER_BOUND ( 'NONE', #75969, .T. ) ;
#46241=CARTESIAN_POINT ( 'NONE',  ( 207.5863589332323329, 29.28491128719180026, 13.57731244650625513 ) ) ;
#46250=ORIENTED_EDGE ( 'NONE', *, *, #67393, .F. ) ;
#46251=CARTESIAN_POINT ( 'NONE',  ( 208.6208076322478746, 32.98517505407394168, 9.000000000000001776 ) ) ;
#46281=EDGE_CURVE ( 'NONE', #16269, #19500, #57276, .T. ) ;
#46283=CARTESIAN_POINT ( 'NONE',  ( 152.4536156746142410, 129.7208004331680797, 12.50000000000000000 ) ) ;
#46284=CARTESIAN_POINT ( 'NONE',  ( 198.7350614680083538, 66.75098366858709653, 10.35296668938518216 ) ) ;
#46292=FACE_OUTER_BOUND ( 'NONE', #45579, .T. ) ;
#46296=CARTESIAN_POINT ( 'NONE',  ( 197.3380612925967057, 18.22700036951244584, -11.15593255764697567 ) ) ;
#46300=ADVANCED_FACE ( 'NONE', ( #38801 ), #24602, .T. ) ;
#46311=DIRECTION ( 'NONE',  ( -1.000000000000000000, 0.000000000000000000, 0.000000000000000000 ) ) ;
#46312=DIRECTION ( 'NONE',  ( 0.3024135303179589229, 0.9531768234071938961, 0.000000000000000000 ) ) ;
#46314=( BOUNDED_CURVE ( )  B_SPLINE_CURVE ( 3, ( #93670, #28829, #57712, #21727 ),
 .UNSPECIFIED., .F., .F. ) 
 B_SPLINE_CURVE_WITH_KNOTS ( ( 4, 4 ),
 ( 1.570796326794896558, 3.141592653589793116 ),
 .UNSPECIFIED. ) 
 CURVE ( )  GEOMETRIC_REPRESENTATION_ITEM ( )  RATIONAL_B_SPLINE_CURVE ( ( 1.000000000000000000, 0.8047378541243649375, 0.8047378541243649375, 1.000000000000000000 ) ) 
 REPRESENTATION_ITEM ( '' )  );
#46321=CARTESIAN_POINT ( 'NONE',  ( 205.7381008070598227, 0.000000000000000000, 7.000000000000000000 ) ) ;
#46324=EDGE_CURVE ( 'NONE', #3893, #48610, #16375, .T. ) ;
#46338=DIRECTION ( 'NONE',  ( 0.09665007798479340051, -0.000000000000000000, 0.9953184226294283787 ) ) ;
#46349=ORIENTED_EDGE ( 'NONE', *, *, #23350, .F. ) ;
#46367=CARTESIAN_POINT ( 'NONE',  ( 157.3400606585842354, 276.0000000000001137, 16.90038786543334126 ) ) ;
#46370=CARTESIAN_POINT ( 'NONE',  ( 196.3496553477289979, 250.0000000000000568, -12.41762739670150850 ) ) ;
#46371=CARTESIAN_POINT ( 'NONE',  ( 196.0583257291930295, 24.84528228517684667, 13.82746528162204491 ) ) ;
#46379=ORIENTED_EDGE ( 'NONE', *, *, #29058, .T. ) ;
#46389=EDGE_LOOP ( 'NONE', ( #67050, #57249, #40443, #93009 ) ) ;
#46390=ORIENTED_EDGE ( 'NONE', *, *, #62476, .F. ) ;
#46391=DIRECTION ( 'NONE',  ( -0.000000000000000000, -1.000000000000000000, -0.000000000000000000 ) ) ;
#46396=CARTESIAN_POINT ( 'NONE',  ( 150.6539576904058606, 293.9636489450775230, 0.000000000000000000 ) ) ;
#46407=ORIENTED_EDGE ( 'NONE', *, *, #17135, .F. ) ;
#46417=CARTESIAN_POINT ( 'NONE',  ( 209.2038787506929793, 35.78193936320073476, 14.26380413240767098 ) ) ;
#46429=CARTESIAN_POINT ( 'NONE',  ( 196.7383257810085695, 24.47698789593438917, 11.00000000000000355 ) ) ;
#46436=FACE_OUTER_BOUND ( 'NONE', #59367, .T. ) ;
#46438=CARTESIAN_POINT ( 'NONE',  ( 200.5336405603944456, 288.1658739788085200, -5.513969000952395838 ) ) ;
#46440=EDGE_CURVE ( 'NONE', #443, #28384, #87435, .T. ) ;
#46442=DIRECTION ( 'NONE',  ( 0.000000000000000000, 0.000000000000000000, -1.000000000000000000 ) ) ;
#46443=DIRECTION ( 'NONE',  ( 0.000000000000000000, 0.000000000000000000, 1.000000000000000000 ) ) ;
#46468=CARTESIAN_POINT ( 'NONE',  ( 185.8632872119974024, 215.0000000000001705, 23.14243616685787330 ) ) ;
#46471=DIRECTION ( 'NONE',  ( -1.000000000000000000, 0.000000000000000000, 0.000000000000000000 ) ) ;
#46478=B_SPLINE_CURVE_WITH_KNOTS ( 'NONE', 3,
 ( #5872, #34741, #26230, #76435, #92480, #4450 ),
 .UNSPECIFIED., .F., .F.,
 ( 4, 2, 4 ),
 ( 0.000000000000000000, 0.0006327419528623999100, 0.001265483905724799820 ),
 .UNSPECIFIED. ) ;
#46487=EDGE_LOOP ( 'NONE', ( #54772, #41262, #40833, #80201, #40914, #57131, #92186 ) ) ;
#46489=VERTEX_POINT ( 'NONE', #83582 ) ;
#46506=CARTESIAN_POINT ( 'NONE',  ( 159.6810783670777880, 8.542400036368780647, 9.000000000000001776 ) ) ;
#46507=EDGE_CURVE ( 'NONE', #25512, #48026, #29489, .T. ) ;
#46513=ORIENTED_EDGE ( 'NONE', *, *, #72006, .T. ) ;
#46521=CARTESIAN_POINT ( 'NONE',  ( 140.0681712527789671, 131.0000000000000568, -11.49999999999999822 ) ) ;
#46525=ORIENTED_EDGE ( 'NONE', *, *, #52600, .T. ) ;
#46540=FACE_OUTER_BOUND ( 'NONE', #49916, .T. ) ;
#46545=EDGE_CURVE ( 'NONE', #3069, #25728, #56134, .T. ) ;
#46547=CIRCLE ( 'NONE', #25399, 9.103929867429224387 ) ;
#46551=DIRECTION ( 'NONE',  ( 1.000000000000000000, 0.000000000000000000, 0.000000000000000000 ) ) ;
#46553=ORIENTED_EDGE ( 'NONE', *, *, #13732, .T. ) ;
#46554=CARTESIAN_POINT ( 'NONE',  ( 202.6531192844960287, 63.25403289339011081, 9.673168394419587202 ) ) ;
#46568=EDGE_CURVE ( 'NONE', #47159, #67960, #77888, .T. ) ;
#46570=EDGE_LOOP ( 'NONE', ( #90713, #31389, #31298, #72611, #34299, #85145 ) ) ;
#46573=CARTESIAN_POINT ( 'NONE',  ( 160.5350683151633291, 250.0000000000000568, 20.22542485937379908 ) ) ;
#46575=VERTEX_POINT ( 'NONE', #77435 ) ;
#46577=CARTESIAN_POINT ( 'NONE',  ( 197.1577115253454338, 71.52895221111288038, 12.06965615694062244 ) ) ;
#46592=DIRECTION ( 'NONE',  ( 0.9251343685759222391, -0.3490264795282477794, -0.1493550021517442705 ) ) ;
#46604=ORIENTED_EDGE ( 'NONE', *, *, #30011, .T. ) ;
#46606=EDGE_LOOP ( 'NONE', ( #9590, #57909, #59135, #56589 ) ) ;
#46612=AXIS2_PLACEMENT_3D ( 'NONE', #44967, #59689, #3286 ) ;
#46621=EDGE_CURVE ( 'NONE', #64177, #65891, #61781, .T. ) ;
#46624=ORIENTED_EDGE ( 'NONE', *, *, #9108, .F. ) ;
#46629=EDGE_LOOP ( 'NONE', ( #49456, #27064 ) ) ;
#46635=CARTESIAN_POINT ( 'NONE',  ( 150.4957602436334412, 21.00000000000000000, -3.637614988394444637 ) ) ;
#46654=CARTESIAN_POINT ( 'NONE',  ( 199.7657144415678658, 24.99747890858082044, 9.999999999999998224 ) ) ;
#46662=LINE ( 'NONE', #75566, #89723 ) ;
#46667=CARTESIAN_POINT ( 'NONE',  ( 153.8109486292483439, 20.54314272855871337, -10.84972530314838579 ) ) ;
#46670=CARTESIAN_POINT ( 'NONE',  ( 164.6329196456214277, 215.0000000000000568, 23.09031830825856346 ) ) ;
#46671=CIRCLE ( 'NONE', #10387, 22.83127060016883192 ) ;
#46683=DIRECTION ( 'NONE',  ( -0.000000000000000000, -1.000000000000000000, -0.000000000000000000 ) ) ;
#46699=DIRECTION ( 'NONE',  ( 0.000000000000000000, 0.000000000000000000, 1.000000000000000000 ) ) ;
#46709=VERTEX_POINT ( 'NONE', #62300 ) ;
#46710=LINE ( 'NONE', #68048, #86421 ) ;
#46721=CYLINDRICAL_SURFACE ( 'NONE', #5508, 6.286090667950827715 ) ;
#46739=FACE_OUTER_BOUND ( 'NONE', #10313, .T. ) ;
#46741=ADVANCED_FACE ( 'NONE', ( #19205 ), #11162, .T. ) ;
#46743=CARTESIAN_POINT ( 'NONE',  ( 138.6539576904058606, 250.5000000000000568, 10.50000000000000000 ) ) ;
#46753=DIRECTION ( 'NONE',  ( -0.000000000000000000, -1.000000000000000000, -0.000000000000000000 ) ) ;
#46755=EDGE_LOOP ( 'NONE', ( #50378, #38375, #93335, #62209 ) ) ;
#46756=EDGE_CURVE ( 'NONE', #69769, #38673, #23981, .T. ) ;
#46757=CARTESIAN_POINT ( 'NONE',  ( 200.2454457599218927, 15.96501597606886769, 10.07064028581559256 ) ) ;
#46771=CARTESIAN_POINT ( 'NONE',  ( 195.9944643786954259, 40.77738931532193334, 13.32058305467766957 ) ) ;
#46779=CYLINDRICAL_SURFACE ( 'NONE', #36822, 2.000000000000000000 ) ;
#46783=DIRECTION ( 'NONE',  ( -0.000000000000000000, -1.000000000000000000, -0.000000000000000000 ) ) ;
#46785=DIRECTION ( 'NONE',  ( 0.000000000000000000, 0.000000000000000000, 1.000000000000000000 ) ) ;
#46792=CARTESIAN_POINT ( 'NONE',  ( 201.2104617360081704, 41.21457449016152452, 10.49999999999999822 ) ) ;
#46795=FACE_OUTER_BOUND ( 'NONE', #7246, .T. ) ;
#46802=VECTOR ( 'NONE', #35071, 1000.000000000000000 ) ;
#46806=DIRECTION ( 'NONE',  ( 0.6056179655966479336, -0.7957555401921982963, 0.000000000000000000 ) ) ;
#46817=ORIENTED_EDGE ( 'NONE', *, *, #18018, .T. ) ;
#46821=CARTESIAN_POINT ( 'NONE',  ( 196.3886764727502054, 69.83403101108301314, -15.08154681515735085 ) ) ;
#46824=EDGE_CURVE ( 'NONE', #27803, #12480, #66318, .T. ) ;
#46829=CARTESIAN_POINT ( 'NONE',  ( 189.4188515237862589, 293.9636489450775798, 9.103929867429222611 ) ) ;
#46837=VERTEX_POINT ( 'NONE', #12097 ) ;
#46843=ADVANCED_FACE ( 'NONE', ( #55202 ), #76920, .F. ) ;
#46849=ORIENTED_EDGE ( 'NONE', *, *, #52243, .T. ) ;
#46855=CARTESIAN_POINT ( 'NONE',  ( 196.1963538710216994, 282.2246705312485915, -40.00000000000000711 ) ) ;
#46867=LINE ( 'NONE', #76709, #20134 ) ;
#46872=CIRCLE ( 'NONE', #69609, 2.999999999999997780 ) ;
#46876=CARTESIAN_POINT ( 'NONE',  ( 207.6662022560303171, 36.29800326561214519, 14.90057469441918947 ) ) ;
#46888=DIRECTION ( 'NONE',  ( -0.000000000000000000, -1.000000000000000000, -0.000000000000000000 ) ) ;
#46890=CARTESIAN_POINT ( 'NONE',  ( 209.5769276792742346, 0.02860196560701893168, 7.415405905516098350 ) ) ;
#46899=DIRECTION ( 'NONE',  ( 0.000000000000000000, 0.000000000000000000, 1.000000000000000000 ) ) ;
#46901=CARTESIAN_POINT ( 'NONE',  ( 198.6462973140338875, 41.50354292539933709, 11.14960445194718019 ) ) ;
#46902=CARTESIAN_POINT ( 'NONE',  ( 151.4851178187871312, 21.00000000000000000, 3.492110388858642889 ) ) ;
#46913=ORIENTED_EDGE ( 'NONE', *, *, #68145, .F. ) ;
#46914=CYLINDRICAL_SURFACE ( 'NONE', #9028, 4.999999999999990230 ) ;
#46917=CARTESIAN_POINT ( 'NONE',  ( 208.4306832106271088, 20.44233620800389772, 0.000000000000000000 ) ) ;
#46944=ORIENTED_EDGE ( 'NONE', *, *, #11778, .F. ) ;
#46946=ORIENTED_EDGE ( 'NONE', *, *, #71569, .T. ) ;
#46957=ORIENTED_EDGE ( 'NONE', *, *, #11727, .F. ) ;
#46964=DIRECTION ( 'NONE',  ( 0.000000000000000000, 0.000000000000000000, 1.000000000000000000 ) ) ;
#46974=EDGE_CURVE ( 'NONE', #60602, #2535, #54766, .T. ) ;
#46981=EDGE_CURVE ( 'NONE', #34296, #4490, #4525, .T. ) ;
#46989=CARTESIAN_POINT ( 'NONE',  ( 165.2494399300530290, 8.542400036368780647, 25.74970488511327815 ) ) ;
#47005=CARTESIAN_POINT ( 'NONE',  ( 175.2296996224750103, 275.0000000000000568, 0.000000000000000000 ) ) ;
#47008=CIRCLE ( 'NONE', #75753, 2.842139515347646750 ) ;
#47010=CARTESIAN_POINT ( 'NONE',  ( 139.1539576904058606, 249.5000000000000568, -10.49999999999999822 ) ) ;
#47012=CARTESIAN_POINT ( 'NONE',  ( 156.3938767642171115, 16.40718364543664620, -10.09124105457608245 ) ) ;
#47014=DIRECTION ( 'NONE',  ( 0.000000000000000000, 1.000000000000000000, 0.000000000000000000 ) ) ;
#47035=CARTESIAN_POINT ( 'NONE',  ( 175.2296996224750103, 276.0000000000000568, 0.000000000000000000 ) ) ;
#47050=PLANE ( 'NONE',  #7621 ) ;
#47063=ORIENTED_EDGE ( 'NONE', *, *, #33369, .T. ) ;
#47083=ORIENTED_EDGE ( 'NONE', *, *, #909, .F. ) ;
#47097=CARTESIAN_POINT ( 'NONE',  ( 151.9826577741344522, 20.03748314401282471, -9.225496140113904175 ) ) ;
#47102=CARTESIAN_POINT ( 'NONE',  ( 201.2104617360081704, 60.19600395700749829, -9.000000000000000000 ) ) ;
#47110=CARTESIAN_POINT ( 'NONE',  ( 154.4002551233161000, 19.39818217137391443, -12.47984618067382634 ) ) ;
#47115=CARTESIAN_POINT ( 'NONE',  ( 199.4392256788250961, 65.82574266882504332, 7.741079165001063522 ) ) ;
#47120=CARTESIAN_POINT ( 'NONE',  ( 208.6208076322478746, 32.98517505407394168, 13.99999999999999822 ) ) ;
#47124=CARTESIAN_POINT ( 'NONE',  ( 197.5007179652673415, 41.86699982721680868, 12.19591313108007036 ) ) ;
#47129=CARTESIAN_POINT ( 'NONE',  ( 153.5035891336125360, 20.65792664182377791, -10.22121553831927088 ) ) ;
#47133=AXIS2_PLACEMENT_3D ( 'NONE', #8342, #73683, #794 ) ;
#47143=ADVANCED_FACE ( 'NONE', ( #79326 ), #78380, .F. ) ;
#47145=EDGE_CURVE ( 'NONE', #71226, #15778, #80231, .T. ) ;
#47159=VERTEX_POINT ( 'NONE', #36674 ) ;
#47162=DIRECTION ( 'NONE',  ( 0.000000000000000000, 0.000000000000000000, -1.000000000000000000 ) ) ;
#47183=LINE ( 'NONE', #48125, #68613 ) ;
#47204=CARTESIAN_POINT ( 'NONE',  ( 222.8344101925596306, 0.000000000000000000, -7.000000000000000888 ) ) ;
#47205=B_SPLINE_CURVE_WITH_KNOTS ( 'NONE', 3,
 ( #19878, #39754, #48749, #77653, #41646, #5688, #13727, #85211 ),
 .UNSPECIFIED., .F., .F.,
 ( 4, 2, 2, 4 ),
 ( 0.000000000000000000, 0.0008360664702759048076, 0.001672132940551809615, 0.003344265881103569357 ),
 .UNSPECIFIED. ) ;
#47215=CIRCLE ( 'NONE', #35147, 0.4999999999999938938 ) ;
#47217=FACE_OUTER_BOUND ( 'NONE', #27154, .T. ) ;
#47221=CARTESIAN_POINT ( 'NONE',  ( 199.4949018615358511, 17.05867184936851899, 10.28330198088169212 ) ) ;
#47234=LINE ( 'NONE', #25937, #30773 ) ;
#47235=CARTESIAN_POINT ( 'NONE',  ( 195.4781563537916043, 39.36132622696000283, 14.00000000000000000 ) ) ;
#47247=EDGE_CURVE ( 'NONE', #27568, #26249, #43653, .T. ) ;
#47255=EDGE_CURVE ( 'NONE', #34296, #64853, #78416, .T. ) ;
#47256=FACE_OUTER_BOUND ( 'NONE', #42742, .T. ) ;
#47267=EDGE_LOOP ( 'NONE', ( #1895, #27823, #78812, #49798 ) ) ;
#47268=CARTESIAN_POINT ( 'NONE',  ( 200.9103445561496244, 65.54396272403067769, -5.212391550061756362 ) ) ;
#47271=DIRECTION ( 'NONE',  ( 0.000000000000000000, -0.7353190267777791611, -0.6777211291221335587 ) ) ;
#47284=FACE_OUTER_BOUND ( 'NONE', #47457, .T. ) ;
#47289=CARTESIAN_POINT ( 'NONE',  ( 169.2744399300530347, 8.542400036368780647, 25.74970488511327815 ) ) ;
#47290=CARTESIAN_POINT ( 'NONE',  ( 195.2949575809873011, 26.08759934769877376, 14.91285779741154016 ) ) ;
#47293=EDGE_CURVE ( 'NONE', #61775, #70030, #40584, .T. ) ;
#47299=VECTOR ( 'NONE', #92948, 1000.000000000000000 ) ;
#47300=ORIENTED_EDGE ( 'NONE', *, *, #26635, .T. ) ;
#47311=FACE_OUTER_BOUND ( 'NONE', #57052, .T. ) ;
#47316=CARTESIAN_POINT ( 'NONE',  ( 200.0272528223206052, 26.57456426123552617, 9.050802287977962379 ) ) ;
#47322=EDGE_CURVE ( 'NONE', #45887, #21613, #86387, .T. ) ;
#47327=VERTEX_POINT ( 'NONE', #50421 ) ;
#47328=FACE_OUTER_BOUND ( 'NONE', #47512, .T. ) ;
#47336=CIRCLE ( 'NONE', #24653, 24.00000000000001066 ) ;
#47351=AXIS2_PLACEMENT_3D ( 'NONE', #55074, #47949, #69745 ) ;
#47353=CARTESIAN_POINT ( 'NONE',  ( 200.2296996224750103, 66.43830042153604154, 2.389358538587006198 ) ) ;
#47358=VECTOR ( 'NONE', #74173, 1000.000000000000000 ) ;
#47367=CARTESIAN_POINT ( 'NONE',  ( 140.6539576904058606, 275.5000000000000568, 10.50000000000000000 ) ) ;
#47369=LINE ( 'NONE', #83838, #9441 ) ;
#47370=DIRECTION ( 'NONE',  ( 0.000000000000000000, 1.000000000000000000, 0.000000000000000000 ) ) ;
#47379=EDGE_CURVE ( 'NONE', #33695, #89141, #7332, .T. ) ;
#47386=CIRCLE ( 'NONE', #68577, 1.499999999999999556 ) ;
#47387=ADVANCED_FACE ( 'NONE', ( #44229 ), #64672, .F. ) ;
#47388=DIRECTION ( 'NONE',  ( 0.000000000000000000, 0.000000000000000000, 1.000000000000000000 ) ) ;
#47398=VECTOR ( 'NONE', #6883, 1000.000000000000000 ) ;
#47401=DIRECTION ( 'NONE',  ( 0.000000000000000000, -0.000000000000000000, 1.000000000000000000 ) ) ;
#47404=VECTOR ( 'NONE', #11265, 1000.000000000000000 ) ;
#47424=CARTESIAN_POINT ( 'NONE',  ( 199.0872936271226479, 69.92583464099142532, -8.677435037599659395 ) ) ;
#47432=CIRCLE ( 'NONE', #21725, 0.5000000000000004441 ) ;
#47443=EDGE_LOOP ( 'NONE', ( #32780, #6459, #57515, #56997, #51538, #28941 ) ) ;
#47452=DIRECTION ( 'NONE',  ( 0.000000000000000000, 1.000000000000000000, 0.000000000000000000 ) ) ;
#47457=EDGE_LOOP ( 'NONE', ( #13709, #4031, #2634, #32390 ) ) ;
#47475=CARTESIAN_POINT ( 'NONE',  ( 208.2002831509629175, 1.063508326896295486, -7.500000000000015099 ) ) ;
#47478=ADVANCED_FACE ( 'NONE', ( #85925 ), #48168, .T. ) ;
#47481=CARTESIAN_POINT ( 'NONE',  ( 209.1374487190023501, 30.94653725228601715, 12.09245862095555601 ) ) ;
#47482=CARTESIAN_POINT ( 'NONE',  ( 196.8803347170859865, 20.19615242270662847, 12.49999999999999289 ) ) ;
#47484=AXIS2_PLACEMENT_3D ( 'NONE', #19187, #48047, #76952 ) ;
#47488=ORIENTED_EDGE ( 'NONE', *, *, #80317, .T. ) ;
#47489=AXIS2_PLACEMENT_3D ( 'NONE', #52968, #66275, #44928 ) ;
#47490=CARTESIAN_POINT ( 'NONE',  ( 159.4851178187871312, 15.00000000000000178, -10.00000000000000178 ) ) ;
#47492=PLANE ( 'NONE',  #52767 ) ;
#47502=CIRCLE ( 'NONE', #91365, 4.999999999999990230 ) ;
#47510=FACE_OUTER_BOUND ( 'NONE', #46755, .T. ) ;
#47512=EDGE_LOOP ( 'NONE', ( #71018, #40777, #26829, #78095 ) ) ;
#47514=CARTESIAN_POINT ( 'NONE',  ( 139.1539576904058606, 276.0000000000000568, -10.49999999999999822 ) ) ;
#47528=ADVANCED_FACE ( 'NONE', ( #66957 ), #24802, .T. ) ;
#47531=FACE_OUTER_BOUND ( 'NONE', #82604, .T. ) ;
#47547=EDGE_LOOP ( 'NONE', ( #34323, #84351, #85168, #17192 ) ) ;
#47569=VERTEX_POINT ( 'NONE', #39439 ) ;
#47584=FACE_OUTER_BOUND ( 'NONE', #48964, .T. ) ;
#47594=B_SPLINE_CURVE_WITH_KNOTS ( 'NONE', 3,
 ( #68239, #62069, #89993, #68712, #69638, #18988, #47840, #18045 ),
 .UNSPECIFIED., .F., .F.,
 ( 4, 2, 2, 4 ),
 ( -8.944277078438763205E-06, 0.001321608365870415719, 0.001986884687344899272, 0.002652161008819382826 ),
 .UNSPECIFIED. ) ;
#47598=CARTESIAN_POINT ( 'NONE',  ( 196.9307570179617244, 70.66253453039786336, 10.51418682698406748 ) ) ;
#47606=CARTESIAN_POINT ( 'NONE',  ( 196.4610981682406532, 41.67863480118781183, 13.65708146052827843 ) ) ;
#47607=CARTESIAN_POINT ( 'NONE',  ( 197.4836817735085219, 42.27872732282707346, 11.66666666666667673 ) ) ;
#47655=ORIENTED_EDGE ( 'NONE', *, *, #34577, .T. ) ;
#47656=CARTESIAN_POINT ( 'NONE',  ( 150.8012326218627948, 131.0000000000000568, -11.50000000000000000 ) ) ;
#47666=DIRECTION ( 'NONE',  ( 0.000000000000000000, 0.000000000000000000, 1.000000000000000000 ) ) ;
#47684=CARTESIAN_POINT ( 'NONE',  ( 175.2296996224750103, 21.00000000000000000, 0.000000000000000000 ) ) ;
#47686=CARTESIAN_POINT ( 'NONE',  ( 219.8344101925596021, 3.000000000000000000, -10.00000000000000000 ) ) ;
#47694=EDGE_CURVE ( 'NONE', #69489, #65034, #93593, .T. ) ;
#47697=EDGE_CURVE ( 'NONE', #67402, #31059, #90525, .T. ) ;
#47698=CARTESIAN_POINT ( 'NONE',  ( 195.8123035524153295, 42.33305793707737053, 12.34482224977402609 ) ) ;
#47700=ORIENTED_EDGE ( 'NONE', *, *, #14640, .T. ) ;
#47702=CARTESIAN_POINT ( 'NONE',  ( 200.7741138073381819, 15.52361751442932025, 10.00000000000000178 ) ) ;
#47716=DIRECTION ( 'NONE',  ( 0.000000000000000000, 1.000000000000000000, 0.000000000000000000 ) ) ;
#47717=CARTESIAN_POINT ( 'NONE',  ( 196.1627136253405581, 40.86402454320599986, 13.15072824800578388 ) ) ;
#47729=DIRECTION ( 'NONE',  ( 0.000000000000000000, 0.000000000000000000, -1.000000000000000000 ) ) ;
#47740=CARTESIAN_POINT ( 'NONE',  ( 195.4997886693276712, 41.25212764115887865, 14.63349899658207498 ) ) ;
#47748=EDGE_LOOP ( 'NONE', ( #33662, #88661, #75770, #91704 ) ) ;
#47749=DIRECTION ( 'NONE',  ( 0.7957555401921946325, 0.6056179655966527076, 0.000000000000000000 ) ) ;
#47771=DIRECTION ( 'NONE',  ( 0.000000000000000000, 1.000000000000000000, 0.000000000000000000 ) ) ;
#47790=EDGE_LOOP ( 'NONE', ( #45199, #72420, #42535, #87736, #79193, #26271 ) ) ;
#47791=DIRECTION ( 'NONE',  ( 0.000000000000000000, 1.000000000000000000, 0.000000000000000000 ) ) ;
#47796=CARTESIAN_POINT ( 'NONE',  ( 197.9084906637196468, 26.03761768678752730, 11.52973355077852524 ) ) ;
#47800=EDGE_CURVE ( 'NONE', #63636, #9221, #19526, .T. ) ;
#47807=VERTEX_POINT ( 'NONE', #87778 ) ;
#47816=CARTESIAN_POINT ( 'NONE',  ( 197.2116943569230045, 249.5000000000000568, -12.92446933126075592 ) ) ;
#47830=CARTESIAN_POINT ( 'NONE',  ( 199.5308170082005290, 67.35660163418374680, 10.35296668938518216 ) ) ;
#47832=CARTESIAN_POINT ( 'NONE',  ( 169.8384340989974532, 249.5000000000000568, -24.41176470588233727 ) ) ;
#47840=CARTESIAN_POINT ( 'NONE',  ( 152.6524812969444724, 129.6175404775655409, -12.50000000000000000 ) ) ;
#47842=CARTESIAN_POINT ( 'NONE',  ( 201.2029632875019729, 287.9274539447415577, -5.251267118318729388 ) ) ;
#47844=CARTESIAN_POINT ( 'NONE',  ( 196.0143093133015384, 42.36571313990103249, 11.99999999999998757 ) ) ;
#47845=CARTESIAN_POINT ( 'NONE',  ( 30.28173832083462358, 95.44497268212424501, 10.00000000000000000 ) ) ;
#47855=ORIENTED_EDGE ( 'NONE', *, *, #63702, .T. ) ;
#47856=CARTESIAN_POINT ( 'NONE',  ( 202.9738562182569694, 293.9636489450776367, -44.00000000000000000 ) ) ;
#47870=ADVANCED_FACE ( 'NONE', ( #16760 ), #88252, .T. ) ;
#47872=CARTESIAN_POINT ( 'NONE',  ( 156.4947056272797852, 20.00000000000000000, -15.00000000000000000 ) ) ;
#47873=CARTESIAN_POINT ( 'NONE',  ( 169.2744399300530347, 8.542400036368780647, -9.000000000000001776 ) ) ;
#47887=ORIENTED_EDGE ( 'NONE', *, *, #21988, .F. ) ;
#47890=AXIS2_PLACEMENT_3D ( 'NONE', #33112, #62000, #5187 ) ;
#47895=EDGE_CURVE ( 'NONE', #86001, #41734, #3483, .T. ) ;
#47896=CARTESIAN_POINT ( 'NONE',  ( 196.4287260171921332, 19.73406386204618457, -13.26569520083611842 ) ) ;
#47901=ORIENTED_EDGE ( 'NONE', *, *, #15031, .T. ) ;
#47908=CARTESIAN_POINT ( 'NONE',  ( 189.9243309297870610, 249.5000000000000568, 20.22542485937349355 ) ) ;
#47913=ORIENTED_EDGE ( 'NONE', *, *, #64946, .F. ) ;
#47920=ORIENTED_EDGE ( 'NONE', *, *, #92, .F. ) ;
#47924=EDGE_CURVE ( 'NONE', #10890, #4223, #53199, .T. ) ;
#47932=DIRECTION ( 'NONE',  ( -0.000000000000000000, -1.000000000000000000, 0.000000000000000000 ) ) ;
#47942=EDGE_CURVE ( 'NONE', #74899, #52690, #57342, .T. ) ;
#47948=DIRECTION ( 'NONE',  ( 0.9693563597868444237, 0.2456588035076248677, -0.000000000000000000 ) ) ;
#47949=DIRECTION ( 'NONE',  ( -0.9531768234071980039, 0.3024135303179465994, 0.000000000000000000 ) ) ;
#47955=ORIENTED_EDGE ( 'NONE', *, *, #73884, .T. ) ;
#47956=CARTESIAN_POINT ( 'NONE',  ( 200.2349812190172713, 66.43136063442170780, 7.741079165001062634 ) ) ;
#47958=CARTESIAN_POINT ( 'NONE',  ( 206.5090647127522629, 29.77167987842737773, 13.94198228246500548 ) ) ;
#47970=ORIENTED_EDGE ( 'NONE', *, *, #66104, .T. ) ;
#47973=CARTESIAN_POINT ( 'NONE',  ( 197.2116943569230330, 276.0000000000000568, -12.92446933126074882 ) ) ;
#47977=DIRECTION ( 'NONE',  ( 0.000000000000000000, 0.000000000000000000, 1.000000000000000000 ) ) ;
#48009=ORIENTED_EDGE ( 'NONE', *, *, #1783, .T. ) ;
#48014=EDGE_CURVE ( 'NONE', #86239, #29030, #4386, .T. ) ;
#48026=VERTEX_POINT ( 'NONE', #38048 ) ;
#48042=CARTESIAN_POINT ( 'NONE',  ( 6.111556883886342995, -24.11587310938936568, 10.00000000000000000 ) ) ;
#48047=DIRECTION ( 'NONE',  ( 0.000000000000000000, 1.000000000000000000, 0.000000000000000000 ) ) ;
#48054=CARTESIAN_POINT ( 'NONE',  ( 153.1901962297478974, 19.73438857712020678, -11.80184082122059230 ) ) ;
#48055=B_SPLINE_CURVE_WITH_KNOTS ( 'NONE', 3,
 ( #7914, #50552, #80351, #29718, #42984, #80820, #37265, #23052, #79895, #87441 ),
 .UNSPECIFIED., .F., .F.,
 ( 4, 2, 2, 2, 4 ),
 ( 0.000000000000000000, 0.0005225403654565069023, 0.001045080730913013805, 0.001567621096369520815, 0.002090161461826027609 ),
 .UNSPECIFIED. ) ;
#48064=CARTESIAN_POINT ( 'NONE',  ( 199.2296996224750387, 68.12454877777268791, 4.237361107270380067 ) ) ;
#48067=CARTESIAN_POINT ( 'NONE',  ( 195.5098045679252721, 40.07219932029098430, 14.92550485056066911 ) ) ;
#48068=DIRECTION ( 'NONE',  ( -0.000000000000000000, -0.000000000000000000, 1.000000000000000000 ) ) ;
#48073=FACE_OUTER_BOUND ( 'NONE', #52174, .T. ) ;
#48082=DIRECTION ( 'NONE',  ( -0.000000000000000000, -0.000000000000000000, -1.000000000000000000 ) ) ;
#48105=CARTESIAN_POINT ( 'NONE',  ( 208.4306832106271656, 1.063508326895939327, -7.500000000000014211 ) ) ;
#48115=VERTEX_POINT ( 'NONE', #3016 ) ;
#48125=CARTESIAN_POINT ( 'NONE',  ( 209.9972545312790544, 27.55378999303204068, 9.000000000000001776 ) ) ;
#48126=CARTESIAN_POINT ( 'NONE',  ( 152.7546676148616029, 130.4533703983872783, -11.50000000000000178 ) ) ;
#48130=EDGE_LOOP ( 'NONE', ( #24468, #44443, #13034, #52818 ) ) ;
#48145=DIRECTION ( 'NONE',  ( 0.000000000000000000, -1.000000000000000000, 0.000000000000000000 ) ) ;
#48156=DIRECTION ( 'NONE',  ( -0.6023974895724014678, -0.000000000000000000, 0.7981962569173501887 ) ) ;
#48163=EDGE_CURVE ( 'NONE', #48925, #78455, #40646, .T. ) ;
#48168=TOROIDAL_SURFACE ( 'NONE', #22501, 24.00000000000000355, 1.000000000000000000 ) ;
#48176=CARTESIAN_POINT ( 'NONE',  ( 193.1193385863660978, 276.0000000000001137, 16.90038786543260940 ) ) ;
#48177=DIRECTION ( 'NONE',  ( -0.000000000000000000, -1.000000000000000000, -0.000000000000000000 ) ) ;
#48189=DIRECTION ( 'NONE',  ( -1.000000000000000000, 0.000000000000000000, 0.000000000000000000 ) ) ;
#48209=ORIENTED_EDGE ( 'NONE', *, *, #26879, .F. ) ;
#48210=DIRECTION ( 'NONE',  ( 0.6056179655966483777, -0.7957555401921979632, 0.000000000000000000 ) ) ;
#48224=VERTEX_POINT ( 'NONE', #83470 ) ;
#48242=ORIENTED_EDGE ( 'NONE', *, *, #82962, .T. ) ;
#48260=CARTESIAN_POINT ( 'NONE',  ( 156.4947056272798136, 20.99999999999998934, -15.00000000000000711 ) ) ;
#48276=CARTESIAN_POINT ( 'NONE',  ( 207.1626556784407001, 29.88353989719039916, 14.95883904121434860 ) ) ;
#48291=EDGE_CURVE ( 'NONE', #34891, #60602, #53602, .T. ) ;
#48298=DIRECTION ( 'NONE',  ( 0.000000000000000000, 0.000000000000000000, -1.000000000000000000 ) ) ;
#48305=AXIS2_PLACEMENT_3D ( 'NONE', #81607, #37140, #24318 ) ;
#48312=CARTESIAN_POINT ( 'NONE',  ( 197.4027394742815602, 40.84896208771628068, 12.00000000000000000 ) ) ;
#48324=VERTEX_POINT ( 'NONE', #54140 ) ;
#48325=DIRECTION ( 'NONE',  ( 1.000000000000000000, 0.000000000000000000, 0.000000000000000000 ) ) ;
#48341=DIRECTION ( 'NONE',  ( 0.000000000000000000, 1.000000000000000000, 0.000000000000000000 ) ) ;
#48355=ORIENTED_EDGE ( 'NONE', *, *, #77442, .T. ) ;
#48367=EDGE_LOOP ( 'NONE', ( #33227, #45407, #14886, #45118 ) ) ;
#48375=FACE_OUTER_BOUND ( 'NONE', #527, .T. ) ;
#48386=VERTEX_POINT ( 'NONE', #56021 ) ;
#48387=DIRECTION ( 'NONE',  ( 0.000000000000000000, 0.000000000000000000, 1.000000000000000000 ) ) ;
#48391=ORIENTED_EDGE ( 'NONE', *, *, #17135, .T. ) ;
#48398=DIRECTION ( 'NONE',  ( -1.000000000000000000, 0.000000000000000000, 0.000000000000000000 ) ) ;
#48414=CARTESIAN_POINT ( 'NONE',  ( 199.0061125298537377, 275.0000000000000568, -7.725424859374024678 ) ) ;
#48419=CYLINDRICAL_SURFACE ( 'NONE', #4517, 24.00000000000001066 ) ;
#48422=CARTESIAN_POINT ( 'NONE',  ( 207.8645969454241538, 36.34083695896440958, 14.87498546835719360 ) ) ;
#48436=ADVANCED_FACE ( 'NONE', ( #12956 ), #47492, .T. ) ;
#48438=CIRCLE ( 'NONE', #45383, 2.046895004029262832 ) ;
#48444=ORIENTED_EDGE ( 'NONE', *, *, #43976, .F. ) ;
#48446=EDGE_CURVE ( 'NONE', #9431, #12419, #70246, .T. ) ;
#48469=DIRECTION ( 'NONE',  ( 0.000000000000000000, 0.000000000000000000, -1.000000000000000000 ) ) ;
#48476=EDGE_CURVE ( 'NONE', #57275, #12480, #24239, .T. ) ;
#48481=ORIENTED_EDGE ( 'NONE', *, *, #34233, .F. ) ;
#48504=ORIENTED_EDGE ( 'NONE', *, *, #29582, .F. ) ;
#48512=DIRECTION ( 'NONE',  ( -4.095251346825558428E-15, 1.000000000000000000, 0.000000000000000000 ) ) ;
#48515=EDGE_CURVE ( 'NONE', #88799, #34891, #66379, .T. ) ;
#48525=CYLINDRICAL_SURFACE ( 'NONE', #45712, 2.999999999999999556 ) ;
#48530=CARTESIAN_POINT ( 'NONE',  ( 198.6884013828325521, 64.61450673763174279, 9.555809373750797420 ) ) ;
#48534=CARTESIAN_POINT ( 'NONE',  ( 200.3359402460285139, 61.72811464988816965, -8.999999999999998224 ) ) ;
#48538=CARTESIAN_POINT ( 'NONE',  ( 175.2296996224750103, 140.2072866198470251, 21.95310499597075804 ) ) ;
#48544=EDGE_CURVE ( 'NONE', #69489, #86306, #31632, .T. ) ;
#48551=DIRECTION ( 'NONE',  ( 0.000000000000000000, 1.000000000000000000, 0.000000000000000000 ) ) ;
#48568=ADVANCED_FACE ( 'NONE', ( #20027 ), #61725, .T. ) ;
#48574=LINE ( 'NONE', #85030, #61143 ) ;
#48576=EDGE_CURVE ( 'NONE', #12173, #30016, #49082, .T. ) ;
#48585=ORIENTED_EDGE ( 'NONE', *, *, #61465, .F. ) ;
#48596=FACE_OUTER_BOUND ( 'NONE', #36358, .T. ) ;
#48597=CARTESIAN_POINT ( 'NONE',  ( 219.8344101925596021, 0.000000000000000000, -7.000000000000000888 ) ) ;
#48601=ORIENTED_EDGE ( 'NONE', *, *, #46545, .F. ) ;
#48610=VERTEX_POINT ( 'NONE', #69287 ) ;
#48614=EDGE_LOOP ( 'NONE', ( #71440, #8111, #75262 ) ) ;
#48617=CARTESIAN_POINT ( 'NONE',  ( 219.8344101925596021, 35.72494958537217968, 7.000000000000000000 ) ) ;
#48618=CARTESIAN_POINT ( 'NONE',  ( 157.2528655986780564, 19.19772955881679621, 10.67418916507565640 ) ) ;
#48624=CARTESIAN_POINT ( 'NONE',  ( 175.2296996224750103, 214.5000000000000568, -25.00000000000000355 ) ) ;
#48626=DIRECTION ( 'NONE',  ( -0.7981962569173501887, 0.000000000000000000, -0.6023974895724014678 ) ) ;
#48627=B_SPLINE_CURVE_WITH_KNOTS ( 'NONE', 3,
 ( #73894, #1009, #66344, #80068 ),
 .UNSPECIFIED., .F., .F.,
 ( 4, 4 ),
 ( 0.000000000000000000, 1.000000000000000000 ),
 .UNSPECIFIED. ) ;
#48631=CARTESIAN_POINT ( 'NONE',  ( 199.1517898866434848, 16.71555987447338509, 10.28330198088196568 ) ) ;
#48633=EDGE_CURVE ( 'NONE', #557, #46575, #79958, .T. ) ;
#48641=CIRCLE ( 'NONE', #77388, 2.000000000000001776 ) ;
#48651=TOROIDAL_SURFACE ( 'NONE', #29002, 24.00000000000002132, 2.046895004029262388 ) ;
#48662=CYLINDRICAL_SURFACE ( 'NONE', #82312, 4.999999999999990230 ) ;
#48674=CARTESIAN_POINT ( 'NONE',  ( 195.1454508245391537, 40.17711433623591688, 15.11173962605491461 ) ) ;
#48695=VERTEX_POINT ( 'NONE', #6775 ) ;
#48696=LINE ( 'NONE', #27409, #68257 ) ;
#48699=CARTESIAN_POINT ( 'NONE',  ( 195.9765076956177268, 73.46773880466290052, -12.06523745212588139 ) ) ;
#48700=ADVANCED_FACE ( 'NONE', ( #14807 ), #92043, .T. ) ;
#48707=AXIS2_PLACEMENT_3D ( 'NONE', #19182, #48512, #11134 ) ;
#48709=CARTESIAN_POINT ( 'NONE',  ( 199.4392256788250961, 65.82574266882505754, -7.741079165001063522 ) ) ;
#48710=AXIS2_PLACEMENT_3D ( 'NONE', #68021, #67564, #31575 ) ;
#48711=LINE ( 'NONE', #42070, #11371 ) ;
#48721=AXIS2_PLACEMENT_3D ( 'NONE', #76042, #55211, #54254 ) ;
#48732=ORIENTED_EDGE ( 'NONE', *, *, #2955, .F. ) ;
#48749=CARTESIAN_POINT ( 'NONE',  ( 194.3470905245161191, 19.98788413800966168, -14.59400273035306483 ) ) ;
#48757=CARTESIAN_POINT ( 'NONE',  ( 156.8041522122653930, 250.5000000000000568, 16.89672165344857646 ) ) ;
#48772=DIRECTION ( 'NONE',  ( 0.000000000000000000, 0.000000000000000000, 1.000000000000000000 ) ) ;
#48773=CIRCLE ( 'NONE', #26129, 3.000000000000000000 ) ;
#48776=CIRCLE ( 'NONE', #29193, 9.103929867429224387 ) ;
#48785=DIRECTION ( 'NONE',  ( -5.551115123125789802E-15, 0.000000000000000000, 1.000000000000000000 ) ) ;
#48795=DIRECTION ( 'NONE',  ( -0.000000000000000000, -1.000000000000000000, -0.000000000000000000 ) ) ;
#48797=CARTESIAN_POINT ( 'NONE',  ( 175.2296996224750103, 20.00000000000000000, 0.000000000000000000 ) ) ;
#48800=VECTOR ( 'NONE', #70044, 1000.000000000000000 ) ;
#48802=( BOUNDED_CURVE ( )  B_SPLINE_CURVE ( 3, ( #9209, #67474, #10615, #17278 ),
 .UNSPECIFIED., .F., .F. ) 
 B_SPLINE_CURVE_WITH_KNOTS ( ( 4, 4 ),
 ( 1.570796326794896558, 2.411864997362828333 ),
 .UNSPECIFIED. ) 
 CURVE ( )  GEOMETRIC_REPRESENTATION_ITEM ( )  RATIONAL_B_SPLINE_CURVE ( ( 1.000000000000000000, 0.9419139527835176384, 0.9419139527835176384, 1.000000000000000000 ) ) 
 REPRESENTATION_ITEM ( '' )  );
#48810=( BOUNDED_SURFACE ( )  B_SPLINE_SURFACE ( 3, 2, ( 
 ( #359, #43442, #51462 ),
 ( #59052, #29246, #35883 ),
 ( #21676, #22140, #72338 ),
 ( #28782, #1287, #7457 ) ),
 .UNSPECIFIED., .F., .F., .F. ) 
 B_SPLINE_SURFACE_WITH_KNOTS ( ( 4, 4 ),
 ( 3, 3 ),
 ( 0.000000000000000000, 0.0009300155619514785879 ),
 ( 0.000000000000000000, 1.000000000000000000 ),
 .UNSPECIFIED. ) 
 GEOMETRIC_REPRESENTATION_ITEM ( )  RATIONAL_B_SPLINE_SURFACE ( (
 ( 1.000000000000000000, 0.8255171224912171146, 1.000000000000000000),
 ( 1.000000000000000000, 0.8158797882023639536, 1.000000000000000000),
 ( 1.000000000000000000, 0.8010468905540685247, 1.000000000000000000),
 ( 1.000000000000000000, 0.7827533893364954087, 1.000000000000000000) ) ) 
 REPRESENTATION_ITEM ( '' )  SURFACE ( )  );
#48812=DIRECTION ( 'NONE',  ( 0.6632250457539263788, -0.000000000000000000, 0.7484200282493129741 ) ) ;
#48814=DIRECTION ( 'NONE',  ( -1.000000000000000000, 0.000000000000000000, 0.000000000000000000 ) ) ;
#48827=ORIENTED_EDGE ( 'NONE', *, *, #90014, .T. ) ;
#48829=ORIENTED_EDGE ( 'NONE', *, *, #11258, .T. ) ;
#48839=AXIS2_PLACEMENT_3D ( 'NONE', #47481, #89624, #11514 ) ;
#48842=AXIS2_PLACEMENT_3D ( 'NONE', #54450, #41152, #91361 ) ;
#48847=CARTESIAN_POINT ( 'NONE',  ( 188.3531807883583440, 45.29379214021909661, 9.000000000000001776 ) ) ;
#48854=ORIENTED_EDGE ( 'NONE', *, *, #6237, .T. ) ;
#48863=CARTESIAN_POINT ( 'NONE',  ( 175.2296996224750103, 20.00000000000000000, 0.000000000000000000 ) ) ;
#48868=ORIENTED_EDGE ( 'NONE', *, *, #53950, .T. ) ;
#48877=AXIS2_PLACEMENT_3D ( 'NONE', #79069, #57307, #50655 ) ;
#48884=EDGE_CURVE ( 'NONE', #65856, #49322, #79208, .T. ) ;
#48886=EDGE_CURVE ( 'NONE', #46489, #78077, #51217, .T. ) ;
#48895=DIRECTION ( 'NONE',  ( 0.000000000000000000, 1.000000000000000000, 0.000000000000000000 ) ) ;
#48900=CARTESIAN_POINT ( 'NONE',  ( 186.6539576904058890, 276.0000000000000568, -11.60392986742922439 ) ) ;
#48902=CARTESIAN_POINT ( 'NONE',  ( 158.6539576904058606, 293.9636489450775230, 11.60392986742922439 ) ) ;
#48907=CARTESIAN_POINT ( 'NONE',  ( 157.4642333713238429, 15.57755555264425240, -7.027845929950948367 ) ) ;
#48918=( GEOMETRIC_REPRESENTATION_CONTEXT ( 3 ) GLOBAL_UNCERTAINTY_ASSIGNED_CONTEXT ( ( #86909 ) ) GLOBAL_UNIT_ASSIGNED_CONTEXT ( ( #60100, #52041, #68118 ) ) REPRESENTATION_CONTEXT ( 'NONE', 'WORKASPACE' ) );
#48919=ORIENTED_EDGE ( 'NONE', *, *, #8888, .T. ) ;
#48923=CARTESIAN_POINT ( 'NONE',  ( 209.8744251295252354, 28.03846817292548366, 12.00000000000000000 ) ) ;
#48925=VERTEX_POINT ( 'NONE', #80116 ) ;
#48938=VECTOR ( 'NONE', #34123, 1000.000000000000000 ) ;
#48944=CIRCLE ( 'NONE', #85244, 4.500000000000003553 ) ;
#48958=VECTOR ( 'NONE', #18896, 1000.000000000000000 ) ;
#48962=ORIENTED_EDGE ( 'NONE', *, *, #70919, .F. ) ;
#48964=EDGE_LOOP ( 'NONE', ( #19956, #91595, #64152, #84029, #5399, #63171, #61692, #78667, #78545, #38812, #46043, #54674, #45052, #85068, #62755, #78586, #56784, #57147, #69490 ) ) ;
#48974=CIRCLE ( 'NONE', #12696, 0.4999999999999979461 ) ;
#48988=ORIENTED_EDGE ( 'NONE', *, *, #3347, .F. ) ;
#48990=ORIENTED_EDGE ( 'NONE', *, *, #5970, .T. ) ;
#48992=EDGE_CURVE ( 'NONE', #11198, #13924, #73928, .T. ) ;
#48993=CIRCLE ( 'NONE', #73201, 7.500000000000012434 ) ;
#48999=CARTESIAN_POINT ( 'NONE',  ( 186.6539576904058890, 293.9636489450775230, 11.60392986742922439 ) ) ;
#49001=EDGE_CURVE ( 'NONE', #59807, #75996, #46671, .T. ) ;
#49003=VECTOR ( 'NONE', #71520, 1000.000000000000000 ) ;
#49006=DIRECTION ( 'NONE',  ( 0.000000000000000000, 1.000000000000000000, 0.000000000000000000 ) ) ;
#49009=CIRCLE ( 'NONE', #20296, 25.00000000000000355 ) ;
#49015=CARTESIAN_POINT ( 'NONE',  ( 197.2116943569230330, 275.5000000000000568, -12.42446933126074882 ) ) ;
#49024=AXIS2_PLACEMENT_3D ( 'NONE', #11437, #85277, #76774 ) ;
#49025=DIRECTION ( 'NONE',  ( 1.110223024625152438E-14, 0.000000000000000000, 1.000000000000000000 ) ) ;
#49028=CARTESIAN_POINT ( 'NONE',  ( 195.4695817506115532, 39.54252710742871812, 15.00000000000000355 ) ) ;
#49029=DIRECTION ( 'NONE',  ( -0.000000000000000000, 1.000000000000000000, -0.000000000000000000 ) ) ;
#49061=CARTESIAN_POINT ( 'NONE',  ( 202.9738562182569694, 293.9636489450776367, -44.00000000000000000 ) ) ;
#49075=CIRCLE ( 'NONE', #33941, 25.00000000000000355 ) ;
#49082=B_SPLINE_CURVE_WITH_KNOTS ( 'NONE', 3,
 ( #11987, #68833, #3961, #54599, #40370, #40836 ),
 .UNSPECIFIED., .F., .F.,
 ( 4, 2, 4 ),
 ( 0.000000000000000000, 0.001526582415388715898, 0.003053164830777431796 ),
 .UNSPECIFIED. ) ;
#49084=DIRECTION ( 'NONE',  ( 0.000000000000000000, 0.000000000000000000, 1.000000000000000000 ) ) ;
#49088=ORIENTED_EDGE ( 'NONE', *, *, #50431, .T. ) ;
#49098=VERTEX_POINT ( 'NONE', #50303 ) ;
#49102=EDGE_LOOP ( 'NONE', ( #72637, #48962, #56713, #87066 ) ) ;
#49104=CARTESIAN_POINT ( 'NONE',  ( 196.8803347170859865, 42.36571313990103249, 12.49999999999999289 ) ) ;
#49105=EDGE_CURVE ( 'NONE', #23354, #28813, #93392, .T. ) ;
#49106=CARTESIAN_POINT ( 'NONE',  ( 154.7156223832783724, 20.48904911123736028, 12.57712157663156560 ) ) ;
#49112=CARTESIAN_POINT ( 'NONE',  ( 192.9182251362765328, 275.0000000000000568, 16.22085278731029945 ) ) ;
#49113=CYLINDRICAL_SURFACE ( 'NONE', #51673, 5.000000000000000888 ) ;
#49117=CARTESIAN_POINT ( 'NONE',  ( 175.2296996224750103, 134.0000000000000284, 24.00000000000001066 ) ) ;
#49120=EDGE_CURVE ( 'NONE', #27913, #20475, #75428, .T. ) ;
#49132=DIRECTION ( 'NONE',  ( -0.000000000000000000, -1.000000000000000000, -0.000000000000000000 ) ) ;
#49133=CARTESIAN_POINT ( 'NONE',  ( 170.4537599243631405, 275.0000000000000568, -23.52000000000000313 ) ) ;
#49145=VECTOR ( 'NONE', #31231, 1000.000000000000000 ) ;
#49147=CARTESIAN_POINT ( 'NONE',  ( 175.2296996224750103, 20.99999999999998934, 25.00000000000000355 ) ) ;
#49159=DIRECTION ( 'NONE',  ( 0.000000000000000000, 1.000000000000000000, -0.000000000000000000 ) ) ;
#49161=TOROIDAL_SURFACE ( 'NONE', #23477, 2.103083949679977582, 2.000000000000000000 ) ;
#49163=LINE ( 'NONE', #34025, #76384 ) ;
#49172=CARTESIAN_POINT ( 'NONE',  ( 152.6002739434462399, 20.65727164547140760, 10.65122728701363464 ) ) ;
#49184=CARTESIAN_POINT ( 'NONE',  ( 195.5501422583016904, 40.28162780827879885, 13.79047839948404786 ) ) ;
#49195=CARTESIAN_POINT ( 'NONE',  ( 198.0307558930329037, 68.10103061380198142, -9.048247235950418244 ) ) ;
#49196=FACE_OUTER_BOUND ( 'NONE', #1670, .T. ) ;
#49216=VERTEX_POINT ( 'NONE', #29479 ) ;
#49217=CARTESIAN_POINT ( 'NONE',  ( 175.2296996224750103, 150.9142415853029036, -22.83127060016886034 ) ) ;
#49233=ORIENTED_EDGE ( 'NONE', *, *, #11598, .T. ) ;
#49238=EDGE_CURVE ( 'NONE', #42443, #70, #35514, .T. ) ;
#49250=CARTESIAN_POINT ( 'NONE',  ( 175.2296996224750103, 275.5000000000000568, 0.000000000000000000 ) ) ;
#49257=EDGE_CURVE ( 'NONE', #92829, #41691, #42170, .T. ) ;
#49269=CYLINDRICAL_SURFACE ( 'NONE', #71112, 5.000000000000000888 ) ;
#49271=DIRECTION ( 'NONE',  ( 1.000000000000000000, 0.000000000000000000, 0.000000000000000000 ) ) ;
#49281=DIRECTION ( 'NONE',  ( 0.000000000000000000, 0.000000000000000000, 1.000000000000000000 ) ) ;
#49288=AXIS2_PLACEMENT_3D ( 'NONE', #4587, #70419, #33950 ) ;
#49296=CARTESIAN_POINT ( 'NONE',  ( 180.7287904564219332, 249.5000000000000568, -24.90000000000002345 ) ) ;
#49297=EDGE_CURVE ( 'NONE', #2535, #39182, #17973, .T. ) ;
#49298=DIRECTION ( 'NONE',  ( 0.000000000000000000, 0.000000000000000000, -1.000000000000000000 ) ) ;
#49311=ORIENTED_EDGE ( 'NONE', *, *, #82549, .F. ) ;
#49322=VERTEX_POINT ( 'NONE', #78731 ) ;
#49335=ORIENTED_EDGE ( 'NONE', *, *, #82962, .F. ) ;
#49343=CARTESIAN_POINT ( 'NONE',  ( 195.5941493172114747, 26.57455637838030071, 13.78431146525796791 ) ) ;
#49353=CARTESIAN_POINT ( 'NONE',  ( 175.2296996224750103, 246.0000000000001137, -9.550761578869391144 ) ) ;
#49369=ADVANCED_FACE ( 'NONE', ( #7679 ), #58523, .F. ) ;
#49372=CARTESIAN_POINT ( 'NONE',  ( 212.7238915819278589, 32.98517505407394168, 10.50000000000000000 ) ) ;
#49379=CARTESIAN_POINT ( 'NONE',  ( 193.6552470326849686, 250.4202232226204785, 16.89672165344822830 ) ) ;
#49381=CARTESIAN_POINT ( 'NONE',  ( 209.8602183316602066, 37.94571256237730239, 12.08763307006258536 ) ) ;
#49384=CARTESIAN_POINT ( 'NONE',  ( 154.7659666677267865, 20.47222690886501439, -12.53936336329526391 ) ) ;
#49387=CARTESIAN_POINT ( 'NONE',  ( 154.1407330040854333, 275.5000000000000568, -13.42592592592594158 ) ) ;
#49394=( BOUNDED_SURFACE ( )  B_SPLINE_SURFACE ( 3, 2, ( 
 ( #33297, #76404, #12465 ),
 ( #4889, #61280, #83957 ),
 ( #25266, #90560, #41312 ),
 ( #69290, #62686, #75920 ),
 ( #91519, #55565, #11045 ),
 ( #34249, #39915, #63155 ),
 ( #68836, #18629, #3964 ),
 ( #91986, #82558, #53691 ),
 ( #93396, #14811, #65483 ),
 ( #34711, #35656, #64094 ),
 ( #20030, #86749, #64571 ),
 ( #20519, #28095, #48907 ),
 ( #14355, #42731, #56982 ),
 ( #36107, #77809, #63625 ) ),
 .UNSPECIFIED., .F., .F., .F. ) 
 B_SPLINE_SURFACE_WITH_KNOTS ( ( 4, 2, 2, 2, 2, 2, 4 ),
 ( 3, 3 ),
 ( 1.986477369973489893, 2.275256190877565921, 2.564035011781641504, 2.708424422233679074, 2.852813832685717088, 2.997203243137755102, 3.141592653589793116 ),
 ( 0.000000000000000000, 1.000000000000000000 ),
 .UNSPECIFIED. ) 
 GEOMETRIC_REPRESENTATION_ITEM ( )  RATIONAL_B_SPLINE_SURFACE ( (
 ( 1.000000000000000000, 0.9583671019092235843, 1.000000000000000000),
 ( 1.000000000000000000, 0.9398658125636398797, 1.000000000000000000),
 ( 1.000000000000000000, 0.9157002655845836170, 1.000000000000000000),
 ( 1.000000000000000000, 0.8622678315320960740, 1.000000000000000000),
 ( 1.000000000000000000, 0.8329613673158866582, 1.000000000000000000),
 ( 1.000000000000000000, 0.7919708659745643420, 1.000000000000000000),
 ( 1.000000000000000000, 0.7788285231914600093, 1.000000000000000000),
 ( 1.000000000000000000, 0.7549177526734387467, 1.000000000000000000),
 ( 1.000000000000000000, 0.7441566529437995126, 1.000000000000000000),
 ( 1.000000000000000000, 0.7262859251462967514, 1.000000000000000000),
 ( 1.000000000000000000, 0.7191857644035031250, 1.000000000000000000),
 ( 1.000000000000000000, 0.7095926089625215205, 1.000000000000000000),
 ( 1.000000000000000000, 0.7070960980132218188, 1.000000000000000000),
 ( 1.000000000000000000, 0.7071067811865473507, 1.000000000000000000) ) ) 
 REPRESENTATION_ITEM ( '' )  SURFACE ( )  );
#49398=ORIENTED_EDGE ( 'NONE', *, *, #55295, .F. ) ;
#49402=ADVANCED_FACE ( 'NONE', ( #29934 ), #18037, .T. ) ;
#49404=ORIENTED_EDGE ( 'NONE', *, *, #29058, .F. ) ;
#49426=ADVANCED_FACE ( 'NONE', ( #53566 ), #17116, .T. ) ;
#49428=FACE_OUTER_BOUND ( 'NONE', #50156, .T. ) ;
#49429=EDGE_CURVE ( 'NONE', #19500, #41151, #31785, .T. ) ;
#49456=ORIENTED_EDGE ( 'NONE', *, *, #51225, .T. ) ;
#49464=EDGE_LOOP ( 'NONE', ( #62519, #29883, #93128 ) ) ;
#49471=DIRECTION ( 'NONE',  ( 0.000000000000000000, 1.000000000000000000, 0.000000000000000000 ) ) ;
#49487=DIRECTION ( 'NONE',  ( -0.000000000000000000, -1.000000000000000000, -0.000000000000000000 ) ) ;
#49490=EDGE_CURVE ( 'NONE', #6854, #1135, #9053, .T. ) ;
#49495=LINE ( 'NONE', #77925, #32295 ) ;
#49510=DIRECTION ( 'NONE',  ( 0.000000000000000000, 0.000000000000000000, -1.000000000000000000 ) ) ;
#49529=EDGE_CURVE ( 'NONE', #35152, #13924, #42222, .T. ) ;
#49536=ORIENTED_EDGE ( 'NONE', *, *, #28070, .T. ) ;
#49537=VERTEX_POINT ( 'NONE', #45981 ) ;
#49547=CARTESIAN_POINT ( 'NONE',  ( 175.2296996224750103, 161.0000000000000853, 0.000000000000000000 ) ) ;
#49548=DIRECTION ( 'NONE',  ( -0.000000000000000000, -1.000000000000000000, -0.000000000000000000 ) ) ;
#49551=EDGE_LOOP ( 'NONE', ( #33450, #83967, #62867, #85210 ) ) ;
#49565=CYLINDRICAL_SURFACE ( 'NONE', #11429, 4.999999999999986677 ) ;
#49567=CARTESIAN_POINT ( 'NONE',  ( 202.9738562182569694, 293.9636489450776367, -44.00000000000000000 ) ) ;
#49574=CARTESIAN_POINT ( 'NONE',  ( 210.1640492649794396, 37.84931640281016030, 15.00000000000000000 ) ) ;
#49576=ORIENTED_EDGE ( 'NONE', *, *, #21333, .F. ) ;
#49577=VERTEX_POINT ( 'NONE', #44586 ) ;
#49578=CARTESIAN_POINT ( 'NONE',  ( 175.2296996224750103, 20.99999999999998934, 0.000000000000000000 ) ) ;
#49592=CARTESIAN_POINT ( 'NONE',  ( 195.4781563537916043, 27.48493576247232895, 13.99999999999999822 ) ) ;
#49608=LINE ( 'NONE', #64792, #14290 ) ;
#49609=CIRCLE ( 'NONE', #63234, 25.00000000000000355 ) ;
#49632=ORIENTED_EDGE ( 'NONE', *, *, #79909, .F. ) ;
#49633=CARTESIAN_POINT ( 'NONE',  ( 151.7498149058253887, 20.88232504567505288, 8.615841630451626543 ) ) ;
#49635=CARTESIAN_POINT ( 'NONE',  ( 209.2890703971520452, 28.92173720827219086, 12.90116063919741407 ) ) ;
#49645=CARTESIAN_POINT ( 'NONE',  ( 195.0629117428269126, 293.9636489450776367, -54.00000000000000000 ) ) ;
#49649=EDGE_CURVE ( 'NONE', #69300, #85724, #89055, .T. ) ;
#49659=CARTESIAN_POINT ( 'NONE',  ( 139.4823848151520735, 130.0000000000000568, 12.50000000000000000 ) ) ;
#49691=EDGE_LOOP ( 'NONE', ( #28744, #2059, #28949, #17902 ) ) ;
#49692=ORIENTED_EDGE ( 'NONE', *, *, #42029, .T. ) ;
#49693=CARTESIAN_POINT ( 'NONE',  ( 208.3936076804783966, 28.69480487596609919, 12.02381566707519944 ) ) ;
#49707=DIRECTION ( 'NONE',  ( 0.000000000000000000, 1.000000000000000000, 0.000000000000000000 ) ) ;
#49717=CARTESIAN_POINT ( 'NONE',  ( 196.0143093133015384, 24.42324672360809856, 11.99999999999998934 ) ) ;
#49719=DIRECTION ( 'NONE',  ( 2.312964634635742267E-15, 0.000000000000000000, 1.000000000000000000 ) ) ;
#49730=CARTESIAN_POINT ( 'NONE',  ( 197.3748232817348764, 214.9910457053126720, -12.45182892472558756 ) ) ;
#49740=AXIS2_PLACEMENT_3D ( 'NONE', #24322, #67438, #1620 ) ;
#49742=VERTEX_POINT ( 'NONE', #88128 ) ;
#49745=DIRECTION ( 'NONE',  ( 0.000000000000000000, 0.000000000000000000, 1.000000000000000000 ) ) ;
#49758=ADVANCED_FACE ( 'NONE', ( #30866, #67775, #9527 ), #8147, .F. ) ;
#49772=ORIENTED_EDGE ( 'NONE', *, *, #68258, .T. ) ;
#49780=ORIENTED_EDGE ( 'NONE', *, *, #66104, .F. ) ;
#49786=CARTESIAN_POINT ( 'NONE',  ( 200.4644824113734387, 249.5000000000000568, -2.942835885954282471 ) ) ;
#49791=VERTEX_POINT ( 'NONE', #24204 ) ;
#49798=ORIENTED_EDGE ( 'NONE', *, *, #82272, .F. ) ;
#49799=CARTESIAN_POINT ( 'NONE',  ( 195.6201958373143270, 24.53660424933035955, 12.66340435719105351 ) ) ;
#49804=CIRCLE ( 'NONE', #66445, 4.999999999999986677 ) ;
#49813=CARTESIAN_POINT ( 'NONE',  ( 189.9243309297870610, 249.5000000000000568, 24.72542485937348644 ) ) ;
#49818=ORIENTED_EDGE ( 'NONE', *, *, #8683, .F. ) ;
#49823=EDGE_CURVE ( 'NONE', #27414, #1443, #34328, .T. ) ;
#49826=CARTESIAN_POINT ( 'NONE',  ( 153.9143451375467748, 19.64542168185916537, 13.06799429260036050 ) ) ;
#49831=CARTESIAN_POINT ( 'NONE',  ( 192.9623460957494956, 250.0000000000000568, 16.90571646082667812 ) ) ;
#49832=FACE_BOUND ( 'NONE', #18428, .T. ) ;
#49834=DIRECTION ( 'NONE',  ( 0.000000000000000000, 0.000000000000000000, 1.000000000000000000 ) ) ;
#49837=CARTESIAN_POINT ( 'NONE',  ( 208.3332195429246383, 35.82735008953291356, 14.32883950752262514 ) ) ;
#49848=ORIENTED_EDGE ( 'NONE', *, *, #6789, .T. ) ;
#49851=DIRECTION ( 'NONE',  ( -0.000000000000000000, -1.000000000000000000, -0.000000000000000000 ) ) ;
#49867=VECTOR ( 'NONE', #2816, 1000.000000000000000 ) ;
#49872=VECTOR ( 'NONE', #49487, 1000.000000000000000 ) ;
#49892=EDGE_CURVE ( 'NONE', #15778, #36174, #83044, .T. ) ;
#49908=EDGE_LOOP ( 'NONE', ( #20779, #51629, #34908, #83150 ) ) ;
#49914=ORIENTED_EDGE ( 'NONE', *, *, #29336, .T. ) ;
#49916=EDGE_LOOP ( 'NONE', ( #31567, #59491, #21241, #42805, #64829 ) ) ;
#49924=LINE ( 'NONE', #22000, #57798 ) ;
#49933=AXIS2_PLACEMENT_3D ( 'NONE', #3522, #59911, #9690 ) ;
#49937=CARTESIAN_POINT ( 'NONE',  ( 0.000000000000000000, 0.000000000000000000, -10.00000000000000000 ) ) ;
#49939=AXIS2_PLACEMENT_3D ( 'NONE', #48900, #5832, #85362 ) ;
#49942=EDGE_CURVE ( 'NONE', #16833, #85072, #5025, .T. ) ;
#49943=LINE ( 'NONE', #78836, #49872 ) ;
#49950=CARTESIAN_POINT ( 'NONE',  ( 184.7149167944524493, 8.542400036368780647, 10.00000000000000000 ) ) ;
#49962=PLANE ( 'NONE',  #89251 ) ;
#49991=ORIENTED_EDGE ( 'NONE', *, *, #52504, .F. ) ;
#49999=AXIS2_PLACEMENT_3D ( 'NONE', #69790, #12989, #63657 ) ;
#50002=DIRECTION ( 'NONE',  ( 0.000000000000000000, 0.000000000000000000, 1.000000000000000000 ) ) ;
#50003=DIRECTION ( 'NONE',  ( 0.000000000000000000, 0.000000000000000000, 1.000000000000000000 ) ) ;
#50005=CIRCLE ( 'NONE', #68131, 0.5000000000000004441 ) ;
#50008=ORIENTED_EDGE ( 'NONE', *, *, #8199, .T. ) ;
#50016=ORIENTED_EDGE ( 'NONE', *, *, #91848, .F. ) ;
#50020=VERTEX_POINT ( 'NONE', #69416 ) ;
#50021=FACE_OUTER_BOUND ( 'NONE', #27323, .T. ) ;
#50023=CARTESIAN_POINT ( 'NONE',  ( 154.4364498827612806, 20.25578850495988092, 11.06489058133685788 ) ) ;
#50029=CARTESIAN_POINT ( 'NONE',  ( 175.2296996224750103, 20.00000000000000000, 0.000000000000000000 ) ) ;
#50030=CARTESIAN_POINT ( 'NONE',  ( 207.2842799582832356, 30.47689859374760957, 12.00000000000000000 ) ) ;
#50032=CARTESIAN_POINT ( 'NONE',  ( 197.8563597697584839, 24.47698789593438917, 12.00000000000000178 ) ) ;
#50048=CARTESIAN_POINT ( 'NONE',  ( 197.5992351617976226, 290.6681976320160743, -7.304042938976587074 ) ) ;
#50049=EDGE_CURVE ( 'NONE', #13111, #55526, #80086, .T. ) ;
#50050=EDGE_CURVE ( 'NONE', #75749, #4469, #21086, .T. ) ;
#50064=FACE_OUTER_BOUND ( 'NONE', #9576, .T. ) ;
#50066=CARTESIAN_POINT ( 'NONE',  ( 196.5738969053448102, 20.46081150943064841, 13.02005007215800880 ) ) ;
#50080=CARTESIAN_POINT ( 'NONE',  ( 183.0442525570908288, 264.6571197653884155, -7.500000000000000000 ) ) ;
#50089=EDGE_CURVE ( 'NONE', #27188, #60755, #73996, .T. ) ;
#50091=EDGE_LOOP ( 'NONE', ( #41627, #18893, #26637, #31497 ) ) ;
#50092=DIRECTION ( 'NONE',  ( -1.000000000000000000, 0.000000000000000000, 0.000000000000000000 ) ) ;
#50103=ORIENTED_EDGE ( 'NONE', *, *, #39485, .F. ) ;
#50104=CARTESIAN_POINT ( 'NONE',  ( 195.4404140996584829, 39.85136009038485838, 13.95084252573039763 ) ) ;
#50110=ORIENTED_EDGE ( 'NONE', *, *, #20685, .T. ) ;
#50116=CARTESIAN_POINT ( 'NONE',  ( 196.6009088602460508, 70.32516635541138328, -11.14992109073990534 ) ) ;
#50138=ORIENTED_EDGE ( 'NONE', *, *, #76026, .T. ) ;
#50139=DIRECTION ( 'NONE',  ( 0.000000000000000000, 0.000000000000000000, 1.000000000000000000 ) ) ;
#50151=CIRCLE ( 'NONE', #60776, 25.00000000000000355 ) ;
#50156=EDGE_LOOP ( 'NONE', ( #5918, #64596, #9579, #31866 ) ) ;
#50172=CARTESIAN_POINT ( 'NONE',  ( 200.2296996224750103, 68.12454877784578855, -2.194831983251746443 ) ) ;
#50173=EDGE_CURVE ( 'NONE', #6854, #10377, #26802, .T. ) ;
#50183=CARTESIAN_POINT ( 'NONE',  ( 175.2296996224750103, 154.6894116713782807, 0.000000000000000000 ) ) ;
#50185=CARTESIAN_POINT ( 'NONE',  ( 208.6208076322478746, 32.98517505407394168, 14.26380412667038655 ) ) ;
#50194=DIRECTION ( 'NONE',  ( -0.000000000000000000, -1.000000000000000000, -0.000000000000000000 ) ) ;
#50195=CARTESIAN_POINT ( 'NONE',  ( 207.6175730408113509, 30.32598770090650575, 14.41714557868298741 ) ) ;
#50205=AXIS2_PLACEMENT_3D ( 'NONE', #34444, #85556, #93581 ) ;
#50206=DIRECTION ( 'NONE',  ( 0.000000000000000000, 0.000000000000000000, 1.000000000000000000 ) ) ;
#50209=DIRECTION ( 'NONE',  ( -1.000000000000000000, -0.000000000000000000, 0.000000000000000000 ) ) ;
#50213=CIRCLE ( 'NONE', #89517, 1.500000000000001332 ) ;
#50222=CARTESIAN_POINT ( 'NONE',  ( 202.8019728163925777, 61.40723988820082724, -9.000000000000000000 ) ) ;
#50223=DIRECTION ( 'NONE',  ( 0.000000000000000000, 0.000000000000000000, -1.000000000000000000 ) ) ;
#50231=EDGE_CURVE ( 'NONE', #20997, #30715, #85011, .T. ) ;
#50235=ORIENTED_EDGE ( 'NONE', *, *, #59139, .T. ) ;
#50242=ORIENTED_EDGE ( 'NONE', *, *, #82641, .F. ) ;
#50243=ORIENTED_EDGE ( 'NONE', *, *, #53950, .F. ) ;
#50249=LINE ( 'NONE', #48847, #27876 ) ;
#50260=VERTEX_POINT ( 'NONE', #69886 ) ;
#50261=CARTESIAN_POINT ( 'NONE',  ( 186.6539576904058890, 293.9636489450775230, 9.103929867429224387 ) ) ;
#50270=AXIS2_PLACEMENT_3D ( 'NONE', #79753, #57067, #22445 ) ;
#50273=CARTESIAN_POINT ( 'NONE',  ( 221.5917695054402543, 1.242640687119284992, 9.999999999999998224 ) ) ;
#50274=CIRCLE ( 'NONE', #35141, 1.499999999999998002 ) ;
#50281=VECTOR ( 'NONE', #56137, 1000.000000000000000 ) ;
#50286=VERTEX_POINT ( 'NONE', #40964 ) ;
#50291=EDGE_CURVE ( 'NONE', #37664, #48386, #26331, .T. ) ;
#50294=CARTESIAN_POINT ( 'NONE',  ( 208.6208076322478746, 32.98517505407394168, 14.49999999999999822 ) ) ;
#50303=CARTESIAN_POINT ( 'NONE',  ( 183.0442525570908288, 296.7472757692770529, 7.499999999999996447 ) ) ;
#50306=CARTESIAN_POINT ( 'NONE',  ( 164.2231345125756263, 293.9636489450775230, 0.000000000000000000 ) ) ;
#50307=CARTESIAN_POINT ( 'NONE',  ( 204.7786681169002350, 32.98517505407394168, 13.99999999999999822 ) ) ;
#50317=VERTEX_POINT ( 'NONE', #5964 ) ;
#50320=CARTESIAN_POINT ( 'NONE',  ( 197.4836817735085219, 24.47698789593438917, 11.66666666666666963 ) ) ;
#50322=EDGE_LOOP ( 'NONE', ( #9615, #26843, #11694, #5670 ) ) ;
#50331=ORIENTED_EDGE ( 'NONE', *, *, #22726, .F. ) ;
#50334=CIRCLE ( 'NONE', #9491, 3.000000000000000000 ) ;
#50338=DIRECTION ( 'NONE',  ( 0.000000000000000000, 1.000000000000000000, 0.000000000000000000 ) ) ;
#50341=AXIS2_PLACEMENT_3D ( 'NONE', #26152, #39873, #11486 ) ;
#50347=VECTOR ( 'NONE', #66392, 1000.000000000000000 ) ;
#50351=AXIS2_PLACEMENT_3D ( 'NONE', #29704, #73260, #88368 ) ;
#50356=ORIENTED_EDGE ( 'NONE', *, *, #49297, .T. ) ;
#50378=ORIENTED_EDGE ( 'NONE', *, *, #43406, .F. ) ;
#50382=AXIS2_PLACEMENT_3D ( 'NONE', #34613, #27037, #10943 ) ;
#50389=EDGE_CURVE ( 'NONE', #57506, #84890, #49804, .T. ) ;
#50398=PLANE ( 'NONE',  #19994 ) ;
#50404=AXIS2_PLACEMENT_3D ( 'NONE', #21180, #57643, #70921 ) ;
#50411=DIRECTION ( 'NONE',  ( 0.000000000000000000, 1.000000000000000000, 0.000000000000000000 ) ) ;
#50412=AXIS2_PLACEMENT_3D ( 'NONE', #26182, #47948, #19548 ) ;
#50419=CIRCLE ( 'NONE', #33794, 1.500000000000003997 ) ;
#50421=CARTESIAN_POINT ( 'NONE',  ( 169.8384340989974817, 250.5000000000000568, -24.41176470588234437 ) ) ;
#50425=CARTESIAN_POINT ( 'NONE',  ( 156.9431851590352665, 250.0000000000000568, 17.51463615629799975 ) ) ;
#50431=EDGE_CURVE ( 'NONE', #51603, #43740, #71301, .T. ) ;
#50435=AXIS2_PLACEMENT_3D ( 'NONE', #93601, #14562, #20256 ) ;
#50473=EDGE_CURVE ( 'NONE', #75506, #49742, #51852, .T. ) ;
#50480=AXIS2_PLACEMENT_3D ( 'NONE', #37678, #73689, #15934 ) ;
#50488=AXIS2_PLACEMENT_3D ( 'NONE', #64905, #50666, #27481 ) ;
#50498=DIRECTION ( 'NONE',  ( -1.000000000000000000, 0.000000000000000000, 0.000000000000000000 ) ) ;
#50499=TOROIDAL_SURFACE ( 'NONE', #9658, 1.500000000000000000, 0.5000000000000000000 ) ;
#50502=CIRCLE ( 'NONE', #85308, 24.99999999999999645 ) ;
#50508=FACE_OUTER_BOUND ( 'NONE', #10011, .T. ) ;
#50509=CARTESIAN_POINT ( 'NONE',  ( 169.7306087885279453, 275.5000000000000568, -24.89999999999999147 ) ) ;
#50511=AXIS2_PLACEMENT_3D ( 'NONE', #53831, #89791, #69904 ) ;
#50512=CARTESIAN_POINT ( 'NONE',  ( 193.9402003287077605, 250.0000000000000568, 16.58062614384823874 ) ) ;
#50529=CARTESIAN_POINT ( 'NONE',  ( 195.7521072783280545, 26.33975396946494385, 13.62141033231749887 ) ) ;
#50530=DIRECTION ( 'NONE',  ( 0.000000000000000000, 0.000000000000000000, -1.000000000000000000 ) ) ;
#50544=DIRECTION ( 'NONE',  ( 0.5831039236546639026, -0.7661730729848326149, -0.2701270746362063879 ) ) ;
#50552=CARTESIAN_POINT ( 'NONE',  ( 209.3315607876652109, 29.46185999635553898, 14.69807322781335301 ) ) ;
#50560=PLANE ( 'NONE',  #1955 ) ;
#50567=AXIS2_PLACEMENT_3D ( 'NONE', #72969, #9011, #65897 ) ;
#50573=AXIS2_PLACEMENT_3D ( 'NONE', #90297, #55284, #84138 ) ;
#50586=EDGE_LOOP ( 'NONE', ( #76468, #56283 ) ) ;
#50587=CARTESIAN_POINT ( 'NONE',  ( 175.2296996224750103, 247.0000000000001137, 0.000000000000000000 ) ) ;
#50593=ORIENTED_EDGE ( 'NONE', *, *, #34052, .T. ) ;
#50597=B_SPLINE_CURVE_WITH_KNOTS ( 'NONE', 3,
 ( #8011, #6171, #21301, #36904, #22681, #64896 ),
 .UNSPECIFIED., .F., .F.,
 ( 4, 2, 4 ),
 ( 1.734723475976807094E-18, 0.0006612700175534703311, 0.001322540035106938927 ),
 .UNSPECIFIED. ) ;
#50601=PLANE ( 'NONE',  #40199 ) ;
#50605=ORIENTED_EDGE ( 'NONE', *, *, #52172, .F. ) ;
#50606=EDGE_CURVE ( 'NONE', #20929, #1176, #75489, .T. ) ;
#50614=VERTEX_POINT ( 'NONE', #52629 ) ;
#50623=ORIENTED_EDGE ( 'NONE', *, *, #44755, .T. ) ;
#50624=FACE_OUTER_BOUND ( 'NONE', #6109, .T. ) ;
#50639=CARTESIAN_POINT ( 'NONE',  ( 156.6297654408069491, 214.9642006536927852, 17.09991073265227968 ) ) ;
#50642=AXIS2_PLACEMENT_3D ( 'NONE', #30819, #15675, #45454 ) ;
#50647=EDGE_CURVE ( 'NONE', #36421, #71850, #19789, .T. ) ;
#50655=DIRECTION ( 'NONE',  ( 0.8435586647355846068, 0.000000000000000000, -0.5370370370370349811 ) ) ;
#50666=DIRECTION ( 'NONE',  ( 0.000000000000000000, 1.000000000000000000, 0.000000000000000000 ) ) ;
#50668=DIRECTION ( 'NONE',  ( -0.3024135303179465439, -0.9531768234071978929, 0.000000000000000000 ) ) ;
#50676=DIRECTION ( 'NONE',  ( -1.000000000000000000, 0.000000000000000000, 0.000000000000000000 ) ) ;
#50679=CARTESIAN_POINT ( 'NONE',  ( 197.5223219362740963, 69.56630120087481828, -11.61486628297207524 ) ) ;
#50680=LINE ( 'NONE', #30759, #82383 ) ;
#50690=DIRECTION ( 'NONE',  ( 0.4995866236608238475, 0.04065491159389757192, -0.8653094149623422604 ) ) ;
#50705=DIRECTION ( 'NONE',  ( 0.000000000000000000, 0.000000000000000000, 1.000000000000000000 ) ) ;
#50718=AXIS2_PLACEMENT_3D ( 'NONE', #5189, #70985, #92265 ) ;
#50719=VERTEX_POINT ( 'NONE', #52175 ) ;
#50724=SHAPE_REPRESENTATION_RELATIONSHIP ( 'NONE' , 'NONE' ,  #80896, #57659 ) ;
#50728=VERTEX_POINT ( 'NONE', #81973 ) ;
#50734=DIRECTION ( 'NONE',  ( 0.000000000000000000, 0.000000000000000000, 1.000000000000000000 ) ) ;
#50747=VERTEX_POINT ( 'NONE', #73952 ) ;
#50757=FACE_OUTER_BOUND ( 'NONE', #81817, .T. ) ;
#50765=ORIENTED_EDGE ( 'NONE', *, *, #24713, .T. ) ;
#50772=CARTESIAN_POINT ( 'NONE',  ( 188.3531807883583440, 45.29379214021909661, 10.50000000000000000 ) ) ;
#50778=DIRECTION ( 'NONE',  ( -6.167905692361989633E-15, 0.000000000000000000, 1.000000000000000000 ) ) ;
#50784=DIRECTION ( 'NONE',  ( 0.000000000000000000, 0.000000000000000000, 1.000000000000000000 ) ) ;
#50794=ORIENTED_EDGE ( 'NONE', *, *, #4124, .T. ) ;
#50797=CARTESIAN_POINT ( 'NONE',  ( 197.4375396935993763, 24.88665474053331650, 11.71825508031673024 ) ) ;
#50799=ORIENTED_EDGE ( 'NONE', *, *, #470, .F. ) ;
#50811=DIRECTION ( 'NONE',  ( 0.000000000000000000, 0.000000000000000000, 1.000000000000000000 ) ) ;
#50812=ADVANCED_FACE ( 'NONE', ( #37493 ), #31344, .T. ) ;
#50815=DIRECTION ( 'NONE',  ( 0.000000000000000000, -0.000000000000000000, 1.000000000000000000 ) ) ;
#50830=ORIENTED_EDGE ( 'NONE', *, *, #75705, .T. ) ;
#50836=EDGE_CURVE ( 'NONE', #43740, #67960, #10447, .T. ) ;
#50853=AXIS2_PLACEMENT_3D ( 'NONE', #7958, #45317, #36853 ) ;
#50859=VERTEX_POINT ( 'NONE', #80586 ) ;
#50862=VERTEX_POINT ( 'NONE', #88616 ) ;
#50871=LINE ( 'NONE', #79303, #6420 ) ;
#50882=CARTESIAN_POINT ( 'NONE',  ( 155.0589890788434388, 20.95955078618711553, 14.77888609071400872 ) ) ;
#50889=CARTESIAN_POINT ( 'NONE',  ( 156.4851178187871312, 0.000000000000000000, 7.000000000000000000 ) ) ;
#50893=DIRECTION ( 'NONE',  ( -0.000000000000000000, -1.000000000000000000, -0.000000000000000000 ) ) ;
#50903=CARTESIAN_POINT ( 'NONE',  ( 170.1758599444071081, 214.8829713991971744, -24.64732457002846644 ) ) ;
#50960=FACE_OUTER_BOUND ( 'NONE', #28161, .T. ) ;
#50961=CARTESIAN_POINT ( 'NONE',  ( 196.5168303497916895, 24.84897060197241814, 13.11473570156704405 ) ) ;
#50968=LINE ( 'NONE', #79852, #35069 ) ;
#50970=CARTESIAN_POINT ( 'NONE',  ( 164.8310050610337498, 214.8829733828359565, 22.91067844396894060 ) ) ;
#50973=EDGE_LOOP ( 'NONE', ( #80144, #85090 ) ) ;
#50974=CYLINDRICAL_SURFACE ( 'NONE', #88245, 0.5000000000000004441 ) ;
#50986=DIRECTION ( 'NONE',  ( 0.000000000000000000, 0.000000000000000000, 1.000000000000000000 ) ) ;
#51002=CARTESIAN_POINT ( 'NONE',  ( 195.1553079136006943, 21.00000000000003553, 15.11292322100999819 ) ) ;
#51024=EDGE_LOOP ( 'NONE', ( #73318, #89134, #19978, #35223 ) ) ;
#51027=DIRECTION ( 'NONE',  ( 8.299690114939509805E-17, -0.7353190267777791611, 0.6777211291221335587 ) ) ;
#51037=ORIENTED_EDGE ( 'NONE', *, *, #51565, .T. ) ;
#51038=CARTESIAN_POINT ( 'NONE',  ( 0.000000000000000000, 3.000000000000000000, 9.000000000000001776 ) ) ;
#51048=CARTESIAN_POINT ( 'NONE',  ( 196.2275967971934847, 72.70402042033215650, -11.63057524128066866 ) ) ;
#51049=CARTESIAN_POINT ( 'NONE',  ( 156.4851178187871312, 1.000000000000000000, -7.000000000000000888 ) ) ;
#51053=ORIENTED_EDGE ( 'NONE', *, *, #34764, .T. ) ;
#51069=EDGE_CURVE ( 'NONE', #26346, #2466, #57404, .T. ) ;
#51071=LINE ( 'NONE', #66686, #41273 ) ;
#51072=DIRECTION ( 'NONE',  ( -0.000000000000000000, -0.000000000000000000, 1.000000000000000000 ) ) ;
#51085=ORIENTED_EDGE ( 'NONE', *, *, #72094, .F. ) ;
#51094=TOROIDAL_SURFACE ( 'NONE', #43590, 2.103083949679977582, 3.000000000000000000 ) ;
#51102=CARTESIAN_POINT ( 'NONE',  ( 196.2452211277167748, 71.67373103464963435, -13.59235650557799779 ) ) ;
#51104=DIRECTION ( 'NONE',  ( -1.110223024625156540E-15, 0.000000000000000000, 1.000000000000000000 ) ) ;
#51115=CARTESIAN_POINT ( 'NONE',  ( 186.6539576904058890, 293.9636489450775230, -9.103929867429224387 ) ) ;
#51117=CARTESIAN_POINT ( 'NONE',  ( 201.6445761222582007, 62.92800856396192444, 6.999999999998341771 ) ) ;
#51125=EDGE_CURVE ( 'NONE', #40555, #38261, #93665, .T. ) ;
#51132=CARTESIAN_POINT ( 'NONE',  ( 175.2296996224750103, 160.0000000000000568, 0.000000000000000000 ) ) ;
#51142=ORIENTED_EDGE ( 'NONE', *, *, #85122, .T. ) ;
#51156=CYLINDRICAL_SURFACE ( 'NONE', #36031, 2.000000000000001776 ) ;
#51167=EDGE_LOOP ( 'NONE', ( #42680, #68799, #3681, #63335 ) ) ;
#51175=ORIENTED_EDGE ( 'NONE', *, *, #50389, .F. ) ;
#51193=EDGE_LOOP ( 'NONE', ( #64260, #27095, #50331, #48732 ) ) ;
#51194=CARTESIAN_POINT ( 'NONE',  ( 196.0068564634292159, 26.11245708493671103, 13.37100780525461374 ) ) ;
#51217=CIRCLE ( 'NONE', #21027, 4.003189038634634045 ) ;
#51218=CARTESIAN_POINT ( 'NONE',  ( 153.4656128104947470, 19.61038002238656475, 12.30465931838429228 ) ) ;
#51223=ADVANCED_FACE ( 'NONE', ( #73506 ), #46914, .T. ) ;
#51225=EDGE_CURVE ( 'NONE', #37664, #14615, #33234, .T. ) ;
#51226=DIRECTION ( 'NONE',  ( -0.000000000000000000, -1.000000000000000000, -0.000000000000000000 ) ) ;
#51228=DIRECTION ( 'NONE',  ( 0.000000000000000000, 0.000000000000000000, 1.000000000000000000 ) ) ;
#51231=FACE_OUTER_BOUND ( 'NONE', #29676, .T. ) ;
#51245=DIRECTION ( 'NONE',  ( -0.000000000000000000, -1.000000000000000000, -0.000000000000000000 ) ) ;
#51258=CARTESIAN_POINT ( 'NONE',  ( 154.6019620322140327, 19.02489598988758601, 11.88315578648355597 ) ) ;
#51261=PLANE ( 'NONE',  #69673 ) ;
#51275=ORIENTED_EDGE ( 'NONE', *, *, #66162, .T. ) ;
#51285=AXIS2_PLACEMENT_3D ( 'NONE', #12600, #34376, #76528 ) ;
#51306=EDGE_CURVE ( 'NONE', #13595, #35945, #10514, .T. ) ;
#51318=DIRECTION ( 'NONE',  ( -0.000000000000000000, -0.000000000000000000, -1.000000000000000000 ) ) ;
#51323=DIRECTION ( 'NONE',  ( 0.000000000000000000, 1.000000000000000000, 0.000000000000000000 ) ) ;
#51325=EDGE_CURVE ( 'NONE', #89945, #14641, #91415, .T. ) ;
#51330=DIRECTION ( 'NONE',  ( 1.000000000000000000, 0.000000000000000000, 0.000000000000000000 ) ) ;
#51333=ADVANCED_FACE ( 'NONE', ( #11886 ), #6023, .T. ) ;
#51334=LINE ( 'NONE', #23405, #52833 ) ;
#51337=CARTESIAN_POINT ( 'NONE',  ( 160.5350683151633291, 250.0000000000000568, 20.22542485937379908 ) ) ;
#51341=LINE ( 'NONE', #1624, #64117 ) ;
#51393=B_SPLINE_CURVE_WITH_KNOTS ( 'NONE', 3,
 ( #41137, #55394, #84246, #62987, #10874, #34084 ),
 .UNSPECIFIED., .F., .F.,
 ( 4, 2, 4 ),
 ( 0.000000000000000000, 0.001526582415388715898, 0.003053164830777431796 ),
 .UNSPECIFIED. ) ;
#51411=DIRECTION ( 'NONE',  ( 1.000000000000000000, 0.000000000000000000, 0.000000000000000000 ) ) ;
#51416=AXIS2_PLACEMENT_3D ( 'NONE', #58208, #7073, #35490 ) ;
#51420=PLANE ( 'NONE',  #66828 ) ;
#51424=VERTEX_POINT ( 'NONE', #90008 ) ;
#51425=CARTESIAN_POINT ( 'NONE',  ( 200.7568414405312751, 39.78480925505072463, 10.49999999999999822 ) ) ;
#51438=CARTESIAN_POINT ( 'NONE',  ( 194.7453183674696504, 19.99999999999992895, 15.62500000000045475 ) ) ;
#51439=CARTESIAN_POINT ( 'NONE',  ( 208.4306832106271088, -74.55766379199613425, 0.000000000000000000 ) ) ;
#51451=EDGE_CURVE ( 'NONE', #27414, #79261, #77227, .T. ) ;
#51455=DIRECTION ( 'NONE',  ( -0.000000000000000000, 1.000000000000000000, 0.000000000000000000 ) ) ;
#51459=EDGE_CURVE ( 'NONE', #69103, #68845, #22625, .T. ) ;
#51462=CARTESIAN_POINT ( 'NONE',  ( 196.8702642586142986, 40.96915988761478644, 12.42857142857142350 ) ) ;
#51475=AXIS2_PLACEMENT_3D ( 'NONE', #81649, #3996, #75491 ) ;
#51478=ORIENTED_EDGE ( 'NONE', *, *, #63587, .T. ) ;
#51479=CARTESIAN_POINT ( 'NONE',  ( 198.6670339576480160, 69.03724764704809047, 9.597602971383192738 ) ) ;
#51490=ORIENTED_EDGE ( 'NONE', *, *, #14384, .T. ) ;
#51501=DIRECTION ( 'NONE',  ( -0.000000000000000000, -1.000000000000000000, -0.000000000000000000 ) ) ;
#51502=FACE_OUTER_BOUND ( 'NONE', #19115, .T. ) ;
#51506=ORIENTED_EDGE ( 'NONE', *, *, #34702, .F. ) ;
#51533=CARTESIAN_POINT ( 'NONE',  ( 196.8803347170859865, 20.19615242270661426, 12.49999999999999289 ) ) ;
#51537=ORIENTED_EDGE ( 'NONE', *, *, #77868, .F. ) ;
#51538=ORIENTED_EDGE ( 'NONE', *, *, #73794, .T. ) ;
#51539=CARTESIAN_POINT ( 'NONE',  ( 198.3325868694534222, 18.45344983985875231, -10.88803913700318127 ) ) ;
#51553=DIRECTION ( 'NONE',  ( 0.000000000000000000, -1.000000000000000000, -0.000000000000000000 ) ) ;
#51554=PLANE ( 'NONE',  #45780 ) ;
#51562=DIRECTION ( 'NONE',  ( -0.000000000000000000, 1.000000000000000000, 0.000000000000000000 ) ) ;
#51565=EDGE_CURVE ( 'NONE', #7087, #70758, #43572, .T. ) ;
#51567=CARTESIAN_POINT ( 'NONE',  ( 194.3144103428324172, 250.0000000000000568, 16.91223866672520515 ) ) ;
#51569=CARTESIAN_POINT ( 'NONE',  ( 151.3711209067282368, 130.9666726753620196, 11.50000000000000178 ) ) ;
#51587=EDGE_CURVE ( 'NONE', #78927, #20997, #34147, .T. ) ;
#51590=ORIENTED_EDGE ( 'NONE', *, *, #50231, .F. ) ;
#51594=DIRECTION ( 'NONE',  ( -0.000000000000000000, -1.000000000000000000, -0.000000000000000000 ) ) ;
#51603=VERTEX_POINT ( 'NONE', #41692 ) ;
#51606=CARTESIAN_POINT ( 'NONE',  ( 198.6884013828325521, 64.61450673763175701, -9.555809373750795643 ) ) ;
#51607=DIRECTION ( 'NONE',  ( -0.000000000000000000, -1.000000000000000000, -0.000000000000000000 ) ) ;
#51610=DIRECTION ( 'NONE',  ( 0.000000000000000000, -0.000000000000000000, 1.000000000000000000 ) ) ;
#51611=CIRCLE ( 'NONE', #63767, 0.4999999999999941158 ) ;
#51617=B_SPLINE_CURVE_WITH_KNOTS ( 'NONE', 3,
 ( #21163, #28742, #50970, #71371, #52711, #79854 ),
 .UNSPECIFIED., .F., .F.,
 ( 4, 2, 4 ),
 ( 0.000000000000000000, 0.0004262108901887123489, 0.0008524217803774246979 ),
 .UNSPECIFIED. ) ;
#51621=ORIENTED_EDGE ( 'NONE', *, *, #56217, .F. ) ;
#51629=ORIENTED_EDGE ( 'NONE', *, *, #73478, .T. ) ;
#51649=DIRECTION ( 'NONE',  ( -0.6056179655966479336, 0.7957555401921982963, 0.000000000000000000 ) ) ;
#51658=CARTESIAN_POINT ( 'NONE',  ( 140.6539576904058606, 0.000000000000000000, 12.50000000000000000 ) ) ;
#51673=AXIS2_PLACEMENT_3D ( 'NONE', #28740, #85086, #92649 ) ;
#51680=CARTESIAN_POINT ( 'NONE',  ( 175.2296996224750103, 134.0000000000000284, 24.00000000000001066 ) ) ;
#51683=CARTESIAN_POINT ( 'NONE',  ( 198.5293976730290524, 24.71549707027390141, 10.72178272431895962 ) ) ;
#51687=DIRECTION ( 'NONE',  ( 0.000000000000000000, 0.000000000000000000, -1.000000000000000000 ) ) ;
#51698=DIRECTION ( 'NONE',  ( 0.7957555401921962979, 0.6056179655966504871, -8.673617379884085762E-16 ) ) ;
#51701=CARTESIAN_POINT ( 'NONE',  ( 188.2019740231993410, 44.81720372851549428, 12.00000000000000000 ) ) ;
#51713=CARTESIAN_POINT ( 'NONE',  ( 197.8598376457711367, 297.6481317602094236, -7.112773483223372217 ) ) ;
#51729=ORIENTED_EDGE ( 'NONE', *, *, #11367, .T. ) ;
#51742=ORIENTED_EDGE ( 'NONE', *, *, #18555, .F. ) ;
#51743=AXIS2_PLACEMENT_3D ( 'NONE', #62772, #6866, #64187 ) ;
#51747=AXIS2_PLACEMENT_3D ( 'NONE', #7917, #23536, #36342 ) ;
#51752=CIRCLE ( 'NONE', #10920, 1.499999999999999556 ) ;
#51758=ORIENTED_EDGE ( 'NONE', *, *, #77632, .F. ) ;
#51766=CARTESIAN_POINT ( 'NONE',  ( 154.1407330040854333, 250.0000000000000568, -13.42592592592592915 ) ) ;
#51773=B_SPLINE_CURVE_WITH_KNOTS ( 'NONE', 3,
 ( #82430, #75332, #10448, #46890, #39314, #18038, #75791, #55434 ),
 .UNSPECIFIED., .F., .F.,
 ( 4, 2, 2, 4 ),
 ( 2.845565583954360595E-21, 0.001369958260980388021, 0.002054937391470581815, 0.002739916521960775609 ),
 .UNSPECIFIED. ) ;
#51780=LINE ( 'NONE', #73584, #4856 ) ;
#51791=DIRECTION ( 'NONE',  ( 0.000000000000000000, 0.000000000000000000, -1.000000000000000000 ) ) ;
#51794=CARTESIAN_POINT ( 'NONE',  ( 195.4781563537916043, 27.42197070042634621, 15.00000000000000000 ) ) ;
#51796=CARTESIAN_POINT ( 'NONE',  ( 175.2296996224750103, 20.99999999999998934, 0.000000000000000000 ) ) ;
#51802=CARTESIAN_POINT ( 'NONE',  ( 164.2231345125756263, 293.9636489450775230, 0.000000000000000000 ) ) ;
#51810=AXIS2_PLACEMENT_3D ( 'NONE', #21531, #13055, #63252 ) ;
#51812=VECTOR ( 'NONE', #55046, 1000.000000000000000 ) ;
#51819=CIRCLE ( 'NONE', #60895, 25.00000000000000355 ) ;
#51847=( BOUNDED_SURFACE ( )  B_SPLINE_SURFACE ( 3, 2, ( 
 ( #85146, #56284, #77113 ),
 ( #93188, #78065, #6090 ),
 ( #63410, #78528, #20761 ),
 ( #91772, #20300, #49633 ),
 ( #28340, #13666, #70958 ),
 ( #41089, #55811, #49172 ),
 ( #92712, #26924, #13208 ),
 ( #42518, #35442, #86072 ) ),
 .UNSPECIFIED., .F., .F., .F. ) 
 B_SPLINE_SURFACE_WITH_KNOTS ( ( 4, 2, 2, 4 ),
 ( 3, 3 ),
 ( 0.000000000000000000, 0.004223792520792201549, 0.006335688781188302324, 0.008447585041584403098 ),
 ( 0.000000000000000000, 1.000000000000000000 ),
 .UNSPECIFIED. ) 
 GEOMETRIC_REPRESENTATION_ITEM ( )  RATIONAL_B_SPLINE_SURFACE ( (
 ( 1.000000000000000000, 0.7071067811865475727, 1.000000000000000000),
 ( 1.000000000000000000, 0.7191403781184984023, 1.000000000000000000),
 ( 1.000000000000000000, 0.7377564866452918091, 1.000000000000000000),
 ( 1.000000000000000000, 0.7710512730019563055, 1.000000000000000000),
 ( 1.000000000000000000, 0.7830816923593915124, 1.000000000000000000),
 ( 1.000000000000000000, 0.8079768302257757107, 1.000000000000000000),
 ( 1.000000000000000000, 0.8207366415442810537, 1.000000000000000000),
 ( 1.000000000000000000, 0.8333723006565931790, 1.000000000000000000) ) ) 
 REPRESENTATION_ITEM ( '' )  SURFACE ( )  );
#51849=VECTOR ( 'NONE', #83854, 1000.000000000000000 ) ;
#51852=( BOUNDED_CURVE ( )  B_SPLINE_CURVE ( 3, ( #77939, #63749, #13083, #41921 ),
 .UNSPECIFIED., .F., .F. ) 
 B_SPLINE_CURVE_WITH_KNOTS ( ( 4, 4 ),
 ( 4.278565243615663150, 4.712388980384691450 ),
 .UNSPECIFIED. ) 
 CURVE ( )  GEOMETRIC_REPRESENTATION_ITEM ( )  RATIONAL_B_SPLINE_CURVE ( ( 1.000000000000000000, 0.9843778111405747655, 0.9843778111405747655, 1.000000000000000000 ) ) 
 REPRESENTATION_ITEM ( '' )  );
#51875=EDGE_LOOP ( 'NONE', ( #78527, #2418, #92945 ) ) ;
#51876=CARTESIAN_POINT ( 'NONE',  ( 175.2296996224750103, 275.5000000000000568, 0.000000000000000000 ) ) ;
#51877=AXIS2_PLACEMENT_3D ( 'NONE', #35860, #86490, #65702 ) ;
#51879=CIRCLE ( 'NONE', #89645, 0.5000000000000004441 ) ;
#51880=VECTOR ( 'NONE', #84152, 1000.000000000000000 ) ;
#51884=CARTESIAN_POINT ( 'NONE',  ( 210.3152560301384142, 38.32590481451375553, 10.00000000000000000 ) ) ;
#51885=CARTESIAN_POINT ( 'NONE',  ( 154.1779308144228651, 20.65864417925001817, 13.49368544356955901 ) ) ;
#51892=CARTESIAN_POINT ( 'NONE',  ( 199.5287591261953253, 41.61473866538664623, 9.179409580634077415 ) ) ;
#51903=CIRCLE ( 'NONE', #48877, 0.4999999999999892308 ) ;
#51906=CARTESIAN_POINT ( 'NONE',  ( 197.8941236165608473, 24.69666864892464986, 9.707778735729039710 ) ) ;
#51908=AXIS2_PLACEMENT_3D ( 'NONE', #1883, #16102, #45411 ) ;
#51916=CARTESIAN_POINT ( 'NONE',  ( 196.0143093133018510, 20.19615242270630517, -11.99999999999943867 ) ) ;
#51921=CARTESIAN_POINT ( 'NONE',  ( 139.6539576904058606, 132.0000000000000568, 10.50000000000000000 ) ) ;
#51930=DIRECTION ( 'NONE',  ( 0.000000000000000000, 0.000000000000000000, -1.000000000000000000 ) ) ;
#51933=DIRECTION ( 'NONE',  ( 0.000000000000000000, 1.000000000000000000, 0.000000000000000000 ) ) ;
#51947=CARTESIAN_POINT ( 'NONE',  ( 153.8109486292483439, 20.54314272855871337, 10.84972530314838579 ) ) ;
#51948=CIRCLE ( 'NONE', #53515, 0.5000000000000004441 ) ;
#51956=AXIS2_PLACEMENT_3D ( 'NONE', #49813, #573, #29457 ) ;
#51961=CARTESIAN_POINT ( 'NONE',  ( 196.4772017995496469, 40.96554989718337225, 12.83327475779042359 ) ) ;
#51965=AXIS2_PLACEMENT_3D ( 'NONE', #55726, #93099, #84578 ) ;
#51973=CARTESIAN_POINT ( 'NONE',  ( 164.6329196456214277, 214.9910457053126720, 23.09031830825856346 ) ) ;
#51974=AXIS2_PLACEMENT_3D ( 'NONE', #93624, #58141, #86987 ) ;
#51979=VERTEX_POINT ( 'NONE', #71072 ) ;
#51997=EDGE_CURVE ( 'NONE', #70265, #70200, #92235, .T. ) ;
#52014=EDGE_CURVE ( 'NONE', #37280, #610, #77705, .T. ) ;
#52015=DIRECTION ( 'NONE',  ( 0.000000000000000000, 1.000000000000000000, 0.000000000000000000 ) ) ;
#52031=DIRECTION ( 'NONE',  ( 0.9693563597868444237, 0.2456588035076248677, 0.000000000000000000 ) ) ;
#52033=CIRCLE ( 'NONE', #23309, 0.5000000000000004441 ) ;
#52041=( NAMED_UNIT ( * ) PLANE_ANGLE_UNIT ( ) SI_UNIT ( $, .RADIAN. ) );
#52042=CIRCLE ( 'NONE', #59568, 24.00000000000001066 ) ;
#52044=AXIS2_PLACEMENT_3D ( 'NONE', #92878, #34656, #64036 ) ;
#52046=DIRECTION ( 'NONE',  ( -0.01818181818181330636, 0.000000000000000000, 0.9998346970812744816 ) ) ;
#52048=DIRECTION ( 'NONE',  ( 0.000000000000000000, 0.000000000000000000, 1.000000000000000000 ) ) ;
#52051=AXIS2_PLACEMENT_3D ( 'NONE', #40810, #77779, #34681 ) ;
#52061=DIRECTION ( 'NONE',  ( -0.5831039236546632365, 0.7661730729848328370, -0.2701270746362063324 ) ) ;
#52072=CARTESIAN_POINT ( 'NONE',  ( 138.6539576904058606, 130.0000000000000568, -10.49999999999999822 ) ) ;
#52087=DIRECTION ( 'NONE',  ( 0.000000000000000000, 1.000000000000000000, 0.000000000000000000 ) ) ;
#52089=ADVANCED_FACE ( 'NONE', ( #63522 ), #20413, .F. ) ;
#52092=LINE ( 'NONE', #81889, #88880 ) ;
#52100=VERTEX_POINT ( 'NONE', #14259 ) ;
#52105=ADVANCED_FACE ( 'NONE', ( #72023 ), #43117, .T. ) ;
#52116=CYLINDRICAL_SURFACE ( 'NONE', #32521, 2.000000000000001776 ) ;
#52124=TOROIDAL_SURFACE ( 'NONE', #41502, 4.499999999999990230, 0.5000000000000000000 ) ;
#52129=CARTESIAN_POINT ( 'NONE',  ( 207.7761861081325776, 35.69891260691534285, 14.41714557868295010 ) ) ;
#52132=ADVANCED_FACE ( 'NONE', ( #86649 ), #92830, .T. ) ;
#52139=CARTESIAN_POINT ( 'NONE',  ( 197.7335303680046650, 24.96166607582781083, 12.00000000000000000 ) ) ;
#52150=CARTESIAN_POINT ( 'NONE',  ( 185.2169494693457921, 249.5000000000000568, 22.91843887563416615 ) ) ;
#52157=CARTESIAN_POINT ( 'NONE',  ( 180.7149167944524493, 8.542400036368780647, 10.00000000000000000 ) ) ;
#52159=DIRECTION ( 'NONE',  ( -0.000000000000000000, 1.000000000000000000, -0.000000000000000000 ) ) ;
#52162=CARTESIAN_POINT ( 'NONE',  ( 201.2104617360081704, 41.21457449016152452, 9.999999999999998224 ) ) ;
#52163=FACE_BOUND ( 'NONE', #27793, .T. ) ;
#52169=AXIS2_PLACEMENT_3D ( 'NONE', #27385, #54843, #85134 ) ;
#52172=EDGE_CURVE ( 'NONE', #59332, #5855, #63559, .T. ) ;
#52174=EDGE_LOOP ( 'NONE', ( #42660, #14404, #70718 ) ) ;
#52175=CARTESIAN_POINT ( 'NONE',  ( 175.2296996224750103, 20.00000000000000000, 24.00000000000000355 ) ) ;
#52178=CARTESIAN_POINT ( 'NONE',  ( 189.9243309297870610, 275.0000000000000568, 20.22542485937349355 ) ) ;
#52183=TOROIDAL_SURFACE ( 'NONE', #62842, 24.50000000000000355, 0.5000000000000000000 ) ;
#52194=DIRECTION ( 'NONE',  ( -0.000000000000000000, -1.000000000000000000, -0.000000000000000000 ) ) ;
#52211=ORIENTED_EDGE ( 'NONE', *, *, #87897, .T. ) ;
#52231=VERTEX_POINT ( 'NONE', #20871 ) ;
#52236=EDGE_CURVE ( 'NONE', #25460, #52628, #85725, .T. ) ;
#52239=ORIENTED_EDGE ( 'NONE', *, *, #90876, .T. ) ;
#52240=CARTESIAN_POINT ( 'NONE',  ( 206.1919228894574303, 35.96217941443950394, 14.00000000000000000 ) ) ;
#52243=EDGE_CURVE ( 'NONE', #90976, #34178, #66752, .T. ) ;
#52244=ORIENTED_EDGE ( 'NONE', *, *, #80432, .F. ) ;
#52255=CARTESIAN_POINT ( 'NONE',  ( 152.4536156746142410, 275.0000000000000568, -14.50000000000000000 ) ) ;
#52261=DIRECTION ( 'NONE',  ( 0.000000000000000000, 1.000000000000000000, 0.000000000000000000 ) ) ;
#52268=CARTESIAN_POINT ( 'NONE',  ( 159.4851178187871312, 15.00000000000000000, 10.00000000000000000 ) ) ;
#52270=ADVANCED_FACE ( 'NONE', ( #58727, #60129 ), #965, .T. ) ;
#52274=CARTESIAN_POINT ( 'NONE',  ( 153.9445672679333939, 19.37982107813205701, -11.06488088134649139 ) ) ;
#52276=CARTESIAN_POINT ( 'NONE',  ( 165.4421947725420523, 250.5000000000000568, 22.46007009812166544 ) ) ;
#52288=ORIENTED_EDGE ( 'NONE', *, *, #43641, .T. ) ;
#52292=DIRECTION ( 'NONE',  ( -0.000000000000000000, -0.000000000000000000, -1.000000000000000000 ) ) ;
#52296=EDGE_CURVE ( 'NONE', #74338, #52100, #23190, .T. ) ;
#52297=CARTESIAN_POINT ( 'NONE',  ( 201.2104617360081704, 0.000000000000000000, 10.00000000000000000 ) ) ;
#52323=VECTOR ( 'NONE', #75624, 1000.000000000000000 ) ;
#52326=VERTEX_POINT ( 'NONE', #8512 ) ;
#52350=CYLINDRICAL_SURFACE ( 'NONE', #65883, 4.999999999999986677 ) ;
#52356=CARTESIAN_POINT ( 'NONE',  ( 196.5880405626493257, 70.38190996880992145, -11.16570917829870702 ) ) ;
#52363=ORIENTED_EDGE ( 'NONE', *, *, #72959, .F. ) ;
#52364=CARTESIAN_POINT ( 'NONE',  ( 200.3691939011709735, 41.41475569181790206, 9.000000000000000000 ) ) ;
#52377=CARTESIAN_POINT ( 'NONE',  ( 151.6545379164648750, 20.00000000000000000, 4.874475407329899923 ) ) ;
#52404=ADVANCED_FACE ( 'NONE', ( #88033 ), #81622, .F. ) ;
#52408=( BOUNDED_CURVE ( )  B_SPLINE_CURVE ( 3, ( #17801, #46654, #75558, #4520 ),
 .UNSPECIFIED., .F., .F. ) 
 B_SPLINE_CURVE_WITH_KNOTS ( ( 4, 4 ),
 ( 4.712388980384689674, 5.553457650952619673 ),
 .UNSPECIFIED. ) 
 CURVE ( )  GEOMETRIC_REPRESENTATION_ITEM ( )  RATIONAL_B_SPLINE_CURVE ( ( 1.000000000000000000, 0.9419139527835179715, 0.9419139527835179715, 1.000000000000000000 ) ) 
 REPRESENTATION_ITEM ( '' )  );
#52420=ORIENTED_EDGE ( 'NONE', *, *, #6914, .F. ) ;
#52421=CARTESIAN_POINT ( 'NONE',  ( 151.6916247871641303, 20.99999999999999645, 4.896253172919318608 ) ) ;
#52442=LINE ( 'NONE', #22628, #26737 ) ;
#52447=EDGE_LOOP ( 'NONE', ( #2040, #34560, #21500, #38478 ) ) ;
#52461=CARTESIAN_POINT ( 'NONE',  ( 169.2744399300530347, 8.542400036368780647, 10.00000000000000000 ) ) ;
#52473=DIRECTION ( 'NONE',  ( 0.000000000000000000, 0.000000000000000000, -1.000000000000000000 ) ) ;
#52477=ORIENTED_EDGE ( 'NONE', *, *, #73694, .T. ) ;
#52478=EDGE_LOOP ( 'NONE', ( #20361, #10630, #79282, #20760 ) ) ;
#52479=FACE_OUTER_BOUND ( 'NONE', #3311, .T. ) ;
#52500=CARTESIAN_POINT ( 'NONE',  ( 152.4536156746142410, 250.0000000000000568, -14.50000000000000000 ) ) ;
#52504=EDGE_CURVE ( 'NONE', #4883, #35594, #59188, .T. ) ;
#52505=DIRECTION ( 'NONE',  ( -0.000000000000000000, -0.000000000000000000, 1.000000000000000000 ) ) ;
#52514=LINE ( 'NONE', #81390, #1815 ) ;
#52517=DIRECTION ( 'NONE',  ( -0.000000000000000000, -0.000000000000000000, -1.000000000000000000 ) ) ;
#52528=VERTEX_POINT ( 'NONE', #52529 ) ;
#52529=CARTESIAN_POINT ( 'NONE',  ( 151.4851178187871312, 21.00000000000000000, -3.492110388858666870 ) ) ;
#52532=DIRECTION ( 'NONE',  ( -0.000000000000000000, -1.000000000000000000, -0.000000000000000000 ) ) ;
#52556=ORIENTED_EDGE ( 'NONE', *, *, #56386, .T. ) ;
#52563=VERTEX_POINT ( 'NONE', #88968 ) ;
#52570=CARTESIAN_POINT ( 'NONE',  ( 219.8344101925596021, 35.72494958537217968, 10.00000000000000000 ) ) ;
#52582=CARTESIAN_POINT ( 'NONE',  ( 207.0561972617101674, 35.35788477359429294, 14.49999999999999822 ) ) ;
#52600=EDGE_CURVE ( 'NONE', #90042, #92711, #77109, .T. ) ;
#52604=CARTESIAN_POINT ( 'NONE',  ( 196.5998995412811041, 25.70598842973115694, 11.15476524095018007 ) ) ;
#52610=CARTESIAN_POINT ( 'NONE',  ( 208.6208076322478746, 32.98517505407394168, 10.50000000000000000 ) ) ;
#52612=DIRECTION ( 'NONE',  ( 0.000000000000000000, -0.000000000000000000, 1.000000000000000000 ) ) ;
#52616=CARTESIAN_POINT ( 'NONE',  ( 175.2296996224750103, 275.0000000000000568, 0.000000000000000000 ) ) ;
#52625=ADVANCED_FACE ( 'NONE', ( #81404 ), #13598, .T. ) ;
#52627=CIRCLE ( 'NONE', #42021, 0.5000000000000004441 ) ;
#52628=VERTEX_POINT ( 'NONE', #80955 ) ;
#52629=CARTESIAN_POINT ( 'NONE',  ( 158.6539576904058606, 293.9636489450775230, -9.103929867429224387 ) ) ;
#52631=CARTESIAN_POINT ( 'NONE',  ( 196.1072012964043267, 25.48927062411483391, 14.15988601298065674 ) ) ;
#52643=CARTESIAN_POINT ( 'NONE',  ( 180.2288731078812702, 275.5000000000000568, -24.90909090909093848 ) ) ;
#52646=DIRECTION ( 'NONE',  ( 8.659560562354828088E-17, 0.7071067811865561215, -0.7071067811865389130 ) ) ;
#52660=ORIENTED_EDGE ( 'NONE', *, *, #6101, .T. ) ;
#52663=EDGE_LOOP ( 'NONE', ( #63354, #69032, #90855, #24336 ) ) ;
#52683=EDGE_LOOP ( 'NONE', ( #74210, #27455, #83059, #15999, #15572 ) ) ;
#52690=VERTEX_POINT ( 'NONE', #37846 ) ;
#52691=CARTESIAN_POINT ( 'NONE',  ( 159.3464669004306984, 16.14910309755062556, 9.103988188768894929 ) ) ;
#52694=ADVANCED_FACE ( 'NONE', ( #1879 ), #72343, .T. ) ;
#52698=VECTOR ( 'NONE', #7789, 1000.000000000000000 ) ;
#52711=CARTESIAN_POINT ( 'NONE',  ( 165.1508121697700346, 214.6009552038360084, 22.87850562931658871 ) ) ;
#52724=CARTESIAN_POINT ( 'NONE',  ( 195.8698257649199377, 19.45052997590691390, 12.70854403887906514 ) ) ;
#52726=CARTESIAN_POINT ( 'NONE',  ( 156.9594811538141244, 18.65395765032456765, -11.57852291560661762 ) ) ;
#52728=CARTESIAN_POINT ( 'NONE',  ( 208.6208076322478746, 32.98517505407394168, 9.000000000000001776 ) ) ;
#52732=CARTESIAN_POINT ( 'NONE',  ( 208.9495066643430903, 38.23465321184740873, 12.02381566707520477 ) ) ;
#52740=B_SPLINE_CURVE_WITH_KNOTS ( 'NONE', 3,
 ( #7105, #43990, #28877, #65353 ),
 .UNSPECIFIED., .F., .F.,
 ( 4, 4 ),
 ( 0.000000000000000000, 9.632970524406137035E-05 ),
 .UNSPECIFIED. ) ;
#52746=DIRECTION ( 'NONE',  ( 0.000000000000000000, 1.000000000000000000, 0.000000000000000000 ) ) ;
#52749=LINE ( 'NONE', #74540, #21631 ) ;
#52756=ADVANCED_FACE ( 'NONE', ( #7586 ), #66512, .T. ) ;
#52765=EDGE_CURVE ( 'NONE', #14152, #70640, #78614, .T. ) ;
#52767=AXIS2_PLACEMENT_3D ( 'NONE', #90557, #62683, #77329 ) ;
#52770=DIRECTION ( 'NONE',  ( 1.000000000000000000, 0.000000000000000000, 0.000000000000000000 ) ) ;
#52783=EDGE_LOOP ( 'NONE', ( #35722, #52288, #80026, #31954 ) ) ;
#52785=VERTEX_POINT ( 'NONE', #89426 ) ;
#52800=VERTEX_POINT ( 'NONE', #31698 ) ;
#52813=CARTESIAN_POINT ( 'NONE',  ( 152.4536156746142410, 130.6065089285656313, -11.50000000000000000 ) ) ;
#52818=ORIENTED_EDGE ( 'NONE', *, *, #21848, .F. ) ;
#52819=CARTESIAN_POINT ( 'NONE',  ( 198.3438837837159383, 40.55036610199213953, 11.14960445194775041 ) ) ;
#52823=EDGE_CURVE ( 'NONE', #13665, #73985, #82759, .T. ) ;
#52826=AXIS2_PLACEMENT_3D ( 'NONE', #1069, #87678, #22829 ) ;
#52833=VECTOR ( 'NONE', #73598, 1000.000000000000000 ) ;
#52846=DIRECTION ( 'NONE',  ( 0.000000000000000000, 1.000000000000000000, 0.000000000000000000 ) ) ;
#52854=DIRECTION ( 'NONE',  ( -0.8660254037844368202, -0.5000000000000032196, 0.000000000000000000 ) ) ;
#52877=ORIENTED_EDGE ( 'NONE', *, *, #68122, .T. ) ;
#52878=CARTESIAN_POINT ( 'NONE',  ( 197.8058612754009289, 70.97294607549092404, 10.93316417084198910 ) ) ;
#52880=CARTESIAN_POINT ( 'NONE',  ( 209.4907211740960804, 29.55254324029474233, 13.48241519114203690 ) ) ;
#52890=ORIENTED_EDGE ( 'NONE', *, *, #38393, .F. ) ;
#52891=CARTESIAN_POINT ( 'NONE',  ( 175.2296996224750103, 275.5000000000000568, 0.000000000000000000 ) ) ;
#52898=AXIS2_PLACEMENT_3D ( 'NONE', #23663, #8051, #74307 ) ;
#52901=CARTESIAN_POINT ( 'NONE',  ( 140.6539576904058606, 275.5000000000000568, 12.00000000000000178 ) ) ;
#52904=TOROIDAL_SURFACE ( 'NONE', #28735, 24.16304133878946558, 4.003189038634632269 ) ;
#52907=ORIENTED_EDGE ( 'NONE', *, *, #72224, .T. ) ;
#52924=CARTESIAN_POINT ( 'NONE',  ( 197.2116943569230330, 250.5000000000000568, -12.92446933126074882 ) ) ;
#52925=CARTESIAN_POINT ( 'NONE',  ( 222.8344101925596306, 0.000000000000000000, 7.000000000000000000 ) ) ;
#52934=EDGE_CURVE ( 'NONE', #24951, #135, #39693, .T. ) ;
#52935=CARTESIAN_POINT ( 'NONE',  ( 184.5358909326088792, 2.965303559109565779, -9.000000000000001776 ) ) ;
#52955=CARTESIAN_POINT ( 'NONE',  ( 155.3770881450957688, 21.00000000067973005, -15.20409621215713969 ) ) ;
#52957=( BOUNDED_CURVE ( )  B_SPLINE_CURVE ( 3, ( #61492, #91260, #90779, #25938 ),
 .UNSPECIFIED., .F., .F. ) 
 B_SPLINE_CURVE_WITH_KNOTS ( ( 4, 4 ),
 ( 2.029441677703989644, 3.141592653589793116 ),
 .UNSPECIFIED. ) 
 CURVE ( )  GEOMETRIC_REPRESENTATION_ITEM ( )  RATIONAL_B_SPLINE_CURVE ( ( 1.000000000000000000, 0.8995554851227762772, 0.8995554851227762772, 1.000000000000000000 ) ) 
 REPRESENTATION_ITEM ( '' )  );
#52964=DIRECTION ( 'NONE',  ( -0.000000000000000000, -1.000000000000000000, -0.000000000000000000 ) ) ;
#52968=CARTESIAN_POINT ( 'NONE',  ( 160.5350683151633291, 250.5000000000000568, 20.22542485937379908 ) ) ;
#52970=TOROIDAL_SURFACE ( 'NONE', #51475, 2.500000000000000000, 0.5000000000000000000 ) ;
#52971=DIRECTION ( 'NONE',  ( -0.000000000000000000, -1.000000000000000000, -0.000000000000000000 ) ) ;
#52972=EDGE_CURVE ( 'NONE', #39851, #73473, #56020, .T. ) ;
#52981=B_SPLINE_CURVE_WITH_KNOTS ( 'NONE', 3,
 ( #1168, #73142, #44705, #73606 ),
 .UNSPECIFIED., .F., .F.,
 ( 4, 4 ),
 ( 0.000000000000000000, 9.632970524405802288E-05 ),
 .UNSPECIFIED. ) ;
#52994=VERTEX_POINT ( 'NONE', #32161 ) ;
#52995=DIRECTION ( 'NONE',  ( 0.000000000000000000, 0.000000000000000000, 1.000000000000000000 ) ) ;
#53008=CARTESIAN_POINT ( 'NONE',  ( 196.7806748523260012, 275.5000000000000568, -12.67104836398113399 ) ) ;
#53013=CARTESIAN_POINT ( 'NONE',  ( 164.2231345125756263, 264.6571197653884155, 7.500000000000000000 ) ) ;
#53031=EDGE_CURVE ( 'NONE', #3893, #81225, #71106, .T. ) ;
#53033=VECTOR ( 'NONE', #67809, 1000.000000000000000 ) ;
#53038=CARTESIAN_POINT ( 'NONE',  ( 200.4946632162240405, 214.9970011440365454, -2.952039013598904749 ) ) ;
#53042=EDGE_CURVE ( 'NONE', #55081, #54755, #60567, .T. ) ;
#53050=EDGE_LOOP ( 'NONE', ( #11233, #53864, #62871, #70407 ) ) ;
#53060=CARTESIAN_POINT ( 'NONE',  ( 175.2296996224750103, 250.0000000000000568, 0.000000000000000000 ) ) ;
#53079=CARTESIAN_POINT ( 'NONE',  ( 197.1656530321902494, 41.90019538913895758, 12.64285714285713169 ) ) ;
#53081=CARTESIAN_POINT ( 'NONE',  ( 194.3594942055387094, 21.00000000000000000, -14.50689422379897842 ) ) ;
#53084=DIRECTION ( 'NONE',  ( 0.000000000000000000, 0.000000000000000000, 1.000000000000000000 ) ) ;
#53098=CARTESIAN_POINT ( 'NONE',  ( 195.8534385314006556, 25.84060167483426085, 14.48761588863094119 ) ) ;
#53102=EDGE_CURVE ( 'NONE', #70513, #47159, #18173, .T. ) ;
#53111=CARTESIAN_POINT ( 'NONE',  ( 157.9772837799791319, 17.93151222991711791, 10.94239627425259442 ) ) ;
#53128=ORIENTED_EDGE ( 'NONE', *, *, #3249, .F. ) ;
#53136=EDGE_CURVE ( 'NONE', #20475, #27913, #83175, .T. ) ;
#53160=ORIENTED_EDGE ( 'NONE', *, *, #15556, .F. ) ;
#53161=CARTESIAN_POINT ( 'NONE',  ( 158.5846220834750397, 17.78059845260490590, 9.675371801486511103 ) ) ;
#53164=ADVANCED_FACE ( 'NONE', ( #61062 ), #17954, .T. ) ;
#53166=ORIENTED_EDGE ( 'NONE', *, *, #51325, .F. ) ;
#53172=AXIS2_PLACEMENT_3D ( 'NONE', #12189, #77060, #32583 ) ;
#53179=DIRECTION ( 'NONE',  ( 0.000000000000000000, 0.000000000000000000, -1.000000000000000000 ) ) ;
#53182=VECTOR ( 'NONE', #37707, 1000.000000000000000 ) ;
#53185=ADVANCED_FACE ( 'NONE', ( #3753 ), #54391, .F. ) ;
#53186=CARTESIAN_POINT ( 'NONE',  ( 219.8344101925596021, 35.72494958537217968, -7.000000000000000888 ) ) ;
#53191=CARTESIAN_POINT ( 'NONE',  ( 160.5350683151633291, 275.0000000000000568, 20.22542485937379908 ) ) ;
#53192=FACE_OUTER_BOUND ( 'NONE', #47547, .T. ) ;
#53197=CARTESIAN_POINT ( 'NONE',  ( 156.0603832538683093, 17.29324094227624187, -10.42473456490740169 ) ) ;
#53199=LINE ( 'NONE', #46097, #11956 ) ;
#53218=FACE_OUTER_BOUND ( 'NONE', #70755, .T. ) ;
#53238=VECTOR ( 'NONE', #83557, 1000.000000000000000 ) ;
#53254=ORIENTED_EDGE ( 'NONE', *, *, #1367, .T. ) ;
#53277=EDGE_CURVE ( 'NONE', #91480, #3443, #78673, .T. ) ;
#53279=B_SPLINE_CURVE_WITH_KNOTS ( 'NONE', 3,
 ( #49104, #64290, #92637, #27330 ),
 .UNSPECIFIED., .F., .F.,
 ( 4, 4 ),
 ( 3.469446951953614189E-18, 0.001032491475659819006 ),
 .UNSPECIFIED. ) ;
#53283=CYLINDRICAL_SURFACE ( 'NONE', #33639, 5.568361562975243650 ) ;
#53290=ADVANCED_FACE ( 'NONE', ( #40625 ), #6086, .T. ) ;
#53298=CIRCLE ( 'NONE', #76018, 24.00000000000001066 ) ;
#53306=CIRCLE ( 'NONE', #1889, 24.00000000000001066 ) ;
#53330=CARTESIAN_POINT ( 'NONE',  ( 165.0427047786672290, 250.0000000000000568, 23.37680765314704701 ) ) ;
#53336=CIRCLE ( 'NONE', #35248, 4.999999999999990230 ) ;
#53345=EDGE_CURVE ( 'NONE', #11375, #23299, #48438, .T. ) ;
#53351=CARTESIAN_POINT ( 'NONE',  ( 175.2296996224750103, 161.0000000000000853, 0.000000000000000000 ) ) ;
#53360=ORIENTED_EDGE ( 'NONE', *, *, #52014, .T. ) ;
#53361=DIRECTION ( 'NONE',  ( -0.8195702660915945570, 1.110223024625169667E-13, 0.5729786897769871823 ) ) ;
#53372=DIRECTION ( 'NONE',  ( -0.9693563597868444237, -0.2456588035076248677, 0.000000000000000000 ) ) ;
#53373=DIRECTION ( 'NONE',  ( 1.000000000000000000, 0.000000000000000000, 0.000000000000000000 ) ) ;
#53377=ORIENTED_EDGE ( 'NONE', *, *, #47942, .F. ) ;
#53378=AXIS2_PLACEMENT_3D ( 'NONE', #59130, #16961, #30240 ) ;
#53385=AXIS2_PLACEMENT_3D ( 'NONE', #38999, #26213, #76420 ) ;
#53388=ORIENTED_EDGE ( 'NONE', *, *, #65647, .T. ) ;
#53396=CARTESIAN_POINT ( 'NONE',  ( 152.5990036449067588, 20.65770287760360802, 10.64853154254647016 ) ) ;
#53397=CARTESIAN_POINT ( 'NONE',  ( 195.9765076956177268, 73.46773880466290052, 12.06523745212588494 ) ) ;
#53406=DIRECTION ( 'NONE',  ( -0.000000000000000000, -0.000000000000000000, 1.000000000000000000 ) ) ;
#53408=CIRCLE ( 'NONE', #82132, 4.499999999999993783 ) ;
#53410=ORIENTED_EDGE ( 'NONE', *, *, #16496, .T. ) ;
#53411=VERTEX_POINT ( 'NONE', #34963 ) ;
#53412=CARTESIAN_POINT ( 'NONE',  ( 200.3378311594553622, 16.04715669186298044, -10.05743975622762143 ) ) ;
#53415=ADVANCED_FACE ( 'NONE', ( #27394 ), #51847, .T. ) ;
#53427=DIRECTION ( 'NONE',  ( 1.000000000000000000, 4.095251346825557639E-15, 0.000000000000000000 ) ) ;
#53428=CYLINDRICAL_SURFACE ( 'NONE', #27708, 6.000000000000000000 ) ;
#53440=AXIS2_PLACEMENT_3D ( 'NONE', #68934, #25361, #18262 ) ;
#53444=CARTESIAN_POINT ( 'NONE',  ( 194.7272697301369533, 20.94006893973816119, 14.00764870559285136 ) ) ;
#53445=AXIS2_PLACEMENT_3D ( 'NONE', #37817, #45377, #9403 ) ;
#53454=AXIS2_PLACEMENT_3D ( 'NONE', #91144, #84523, #18749 ) ;
#53457=CARTESIAN_POINT ( 'NONE',  ( 207.4428545773736801, 30.38304882718446009, 15.03172026577670550 ) ) ;
#53463=AXIS2_PLACEMENT_3D ( 'NONE', #56010, #48895, #70695 ) ;
#53468=ORIENTED_EDGE ( 'NONE', *, *, #4411, .T. ) ;
#53469=DIRECTION ( 'NONE',  ( 0.000000000000000000, 0.000000000000000000, 1.000000000000000000 ) ) ;
#53476=EDGE_CURVE ( 'NONE', #73850, #60939, #46872, .T. ) ;
#53477=EDGE_CURVE ( 'NONE', #16833, #75053, #33306, .T. ) ;
#53484=EDGE_LOOP ( 'NONE', ( #78562, #81321, #41270, #84370 ) ) ;
#53488=CARTESIAN_POINT ( 'NONE',  ( 185.4166944662902665, 214.7015631973135044, 22.87680765314684095 ) ) ;
#53490=DIRECTION ( 'NONE',  ( 0.8660254037844405950, -0.4999999999999966693, 0.000000000000000000 ) ) ;
#53494=DIRECTION ( 'NONE',  ( 0.000000000000000000, 1.000000000000000000, 0.000000000000000000 ) ) ;
#53495=DIRECTION ( 'NONE',  ( 0.000000000000000000, 1.000000000000000000, 0.000000000000000000 ) ) ;
#53503=ORIENTED_EDGE ( 'NONE', *, *, #56386, .F. ) ;
#53514=EDGE_CURVE ( 'NONE', #70776, #87978, #63875, .T. ) ;
#53515=AXIS2_PLACEMENT_3D ( 'NONE', #92187, #12683, #34909 ) ;
#53520=CARTESIAN_POINT ( 'NONE',  ( 150.7108941768076704, 21.00000000000001066, -5.100416763304296275 ) ) ;
#53526=AXIS2_PLACEMENT_3D ( 'NONE', #43092, #20846, #7116 ) ;
#53532=ORIENTED_EDGE ( 'NONE', *, *, #20809, .T. ) ;
#53533=DIRECTION ( 'NONE',  ( 0.000000000000000000, 0.000000000000000000, 1.000000000000000000 ) ) ;
#53535=CIRCLE ( 'NONE', #24811, 11.60392986742922439 ) ;
#53558=CARTESIAN_POINT ( 'NONE',  ( 157.4851178187871312, 69.18068689461284748, 10.00000000000000000 ) ) ;
#53566=FACE_OUTER_BOUND ( 'NONE', #67944, .T. ) ;
#53569=CARTESIAN_POINT ( 'NONE',  ( 185.4166944662832179, 215.0000000000000568, 23.37680765314684095 ) ) ;
#53570=DIRECTION ( 'NONE',  ( 0.000000000000000000, 1.000000000000000000, 0.000000000000000000 ) ) ;
#53580=CIRCLE ( 'NONE', #32369, 0.4999999999999998890 ) ;
#53581=DIRECTION ( 'NONE',  ( -1.000000000000000000, 0.000000000000000000, 0.000000000000000000 ) ) ;
#53584=CYLINDRICAL_SURFACE ( 'NONE', #20103, 2.000000000000000000 ) ;
#53598=CARTESIAN_POINT ( 'NONE',  ( 156.3938767642113703, 16.40718364543451813, 10.09124105457537368 ) ) ;
#53602=B_SPLINE_CURVE_WITH_KNOTS ( 'NONE', 3,
 ( #26672, #90111, #32835, #91983 ),
 .UNSPECIFIED., .F., .F.,
 ( 4, 4 ),
 ( 0.000000000000000000, 0.0008009674008372812039 ),
 .UNSPECIFIED. ) ;
#53618=ORIENTED_EDGE ( 'NONE', *, *, #93562, .F. ) ;
#53620=EDGE_LOOP ( 'NONE', ( #58766, #11807, #38881, #2051 ) ) ;
#53642=ORIENTED_EDGE ( 'NONE', *, *, #32523, .T. ) ;
#53650=DIRECTION ( 'NONE',  ( 1.000000000000000000, 0.000000000000000000, -0.000000000000000000 ) ) ;
#53655=EDGE_LOOP ( 'NONE', ( #78783, #74471, #52890, #48585 ) ) ;
#53666=DIRECTION ( 'NONE',  ( -0.7806247497998081153, 0.000000000000000000, 0.6249999999999895639 ) ) ;
#53670=CARTESIAN_POINT ( 'NONE',  ( 175.2296996224750103, 154.6894116713782807, 0.000000000000000000 ) ) ;
#53671=EDGE_CURVE ( 'NONE', #64817, #23459, #42358, .T. ) ;
#53677=CARTESIAN_POINT ( 'NONE',  ( 210.6908326509675362, 1.000000000000000000, 7.166337341072457789 ) ) ;
#53678=DIRECTION ( 'NONE',  ( -0.000000000000000000, -1.000000000000000000, -0.000000000000000000 ) ) ;
#53682=CARTESIAN_POINT ( 'NONE',  ( 189.4188515237862589, 293.9636489450775798, 9.103929867429222611 ) ) ;
#53684=ORIENTED_EDGE ( 'NONE', *, *, #62476, .T. ) ;
#53685=LINE ( 'NONE', #76398, #9294 ) ;
#53691=CARTESIAN_POINT ( 'NONE',  ( 157.0521749816625743, 17.25638377770970777, -7.577257116167048778 ) ) ;
#53698=EDGE_CURVE ( 'NONE', #24267, #45543, #12736, .T. ) ;
#53703=DIRECTION ( 'NONE',  ( 0.000000000000000000, 0.000000000000000000, 1.000000000000000000 ) ) ;
#53705=ORIENTED_EDGE ( 'NONE', *, *, #24919, .F. ) ;
#53707=CARTESIAN_POINT ( 'NONE',  ( 197.8478357033531267, 68.18663436155952695, 11.29153850601979592 ) ) ;
#53725=CARTESIAN_POINT ( 'NONE',  ( 205.2786681169002350, 32.98517505407394168, 14.49999999999999822 ) ) ;
#53738=VERTEX_POINT ( 'NONE', #70501 ) ;
#53766=DIRECTION ( 'NONE',  ( -1.000000000000000000, 0.000000000000000000, 0.000000000000000000 ) ) ;
#53791=CARTESIAN_POINT ( 'NONE',  ( 221.8344101925596306, 1.000000000000000222, 7.000000000000000000 ) ) ;
#53797=CARTESIAN_POINT ( 'NONE',  ( 152.9410204041312795, 20.82809642979767872, -8.928152258827880772 ) ) ;
#53799=EDGE_CURVE ( 'NONE', #23700, #68064, #90722, .T. ) ;
#53810=FACE_OUTER_BOUND ( 'NONE', #29440, .T. ) ;
#53824=ADVANCED_FACE ( 'NONE', ( #35900 ), #26983, .T. ) ;
#53825=EDGE_CURVE ( 'NONE', #14772, #1176, #80367, .T. ) ;
#53828=ORIENTED_EDGE ( 'NONE', *, *, #56142, .F. ) ;
#53829=CARTESIAN_POINT ( 'NONE',  ( 198.8657840505796628, 68.63430910526400908, 9.310452007619588244 ) ) ;
#53831=CARTESIAN_POINT ( 'NONE',  ( 154.5625123364532101, 275.5000000000000568, -13.15740740740742787 ) ) ;
#53851=FACE_OUTER_BOUND ( 'NONE', #10517, .T. ) ;
#53852=CARTESIAN_POINT ( 'NONE',  ( 222.8344101925596306, 0.000000000000000000, 10.00000000000000000 ) ) ;
#53864=ORIENTED_EDGE ( 'NONE', *, *, #76674, .T. ) ;
#53869=DIRECTION ( 'NONE',  ( 0.000000000000000000, 1.000000000000000000, 0.000000000000000000 ) ) ;
#53872=DIRECTION ( 'NONE',  ( 0.000000000000000000, -1.000000000000000000, 0.000000000000000000 ) ) ;
#53873=CARTESIAN_POINT ( 'NONE',  ( 200.1063562619108609, 64.94916223746493245, 5.267193185414368095 ) ) ;
#53881=CARTESIAN_POINT ( 'NONE',  ( 194.2984252800551417, 39.76179767010464161, 14.57344116787098720 ) ) ;
#53883=ORIENTED_EDGE ( 'NONE', *, *, #15423, .T. ) ;
#53884=LINE ( 'NONE', #86015, #79223 ) ;
#53899=FACE_OUTER_BOUND ( 'NONE', #12750, .T. ) ;
#53900=CARTESIAN_POINT ( 'NONE',  ( 156.4851178187871312, 15.00000000000000000, 7.000000000000000000 ) ) ;
#53908=CARTESIAN_POINT ( 'NONE',  ( 154.7659666677267580, 19.56018909072085066, 12.94946946941272437 ) ) ;
#53912=DIRECTION ( 'NONE',  ( 0.5068419345592570791, -1.196319445165339194E-14, 0.8620390091940327570 ) ) ;
#53914=CARTESIAN_POINT ( 'NONE',  ( 152.4536156746142410, 276.0000000000000568, -11.99999999999999112 ) ) ;
#53921=CARTESIAN_POINT ( 'NONE',  ( 175.2296996224750103, 249.5000000000000568, 0.000000000000000000 ) ) ;
#53924=CARTESIAN_POINT ( 'NONE',  ( 207.3682846056400990, 30.42003702808571930, 14.46447120960799992 ) ) ;
#53933=ORIENTED_EDGE ( 'NONE', *, *, #41260, .F. ) ;
#53934=CARTESIAN_POINT ( 'NONE',  ( 152.4536156746142410, 249.5000000000000568, 12.00000000000000000 ) ) ;
#53936=LINE ( 'NONE', #82805, #39868 ) ;
#53943=EDGE_CURVE ( 'NONE', #80622, #53974, #18336, .T. ) ;
#53949=DIRECTION ( 'NONE',  ( 0.000000000000000000, 0.000000000000000000, 1.000000000000000000 ) ) ;
#53950=EDGE_CURVE ( 'NONE', #11243, #4576, #9316, .T. ) ;
#53956=DIRECTION ( 'NONE',  ( 1.000000000000000000, 0.000000000000000000, 0.000000000000000000 ) ) ;
#53974=VERTEX_POINT ( 'NONE', #66640 ) ;
#54001=CARTESIAN_POINT ( 'NONE',  ( 208.3342852401368930, 35.82745088358564800, 14.32871520589203485 ) ) ;
#54006=EDGE_CURVE ( 'NONE', #25330, #1451, #30651, .T. ) ;
#54013=CARTESIAN_POINT ( 'NONE',  ( 199.8839601302323388, 66.89258700486192311, 4.790067391029672272 ) ) ;
#54015=DIRECTION ( 'NONE',  ( 0.8526555397811738102, 0.000000000000000000, -0.5224734734706395489 ) ) ;
#54022=DIRECTION ( 'NONE',  ( -1.000000000000000000, 0.000000000000000000, 0.000000000000000000 ) ) ;
#54026=CARTESIAN_POINT ( 'NONE',  ( 199.7979780134897396, 41.13815025368441525, 10.63455718547532314 ) ) ;
#54037=DIRECTION ( 'NONE',  ( 0.000000000000000000, 0.000000000000000000, 1.000000000000000000 ) ) ;
#54040=CARTESIAN_POINT ( 'NONE',  ( 175.2296996224750103, 133.0000000000000000, 0.000000000000000000 ) ) ;
#54051=CARTESIAN_POINT ( 'NONE',  ( 159.4572718888341285, 15.48129629386906281, 10.01740370621924292 ) ) ;
#54065=EDGE_CURVE ( 'NONE', #85072, #57747, #31131, .T. ) ;
#54068=ORIENTED_EDGE ( 'NONE', *, *, #71679, .T. ) ;
#54087=DIRECTION ( 'NONE',  ( 1.000000000000000000, -0.000000000000000000, -0.000000000000000000 ) ) ;
#54100=CARTESIAN_POINT ( 'NONE',  ( 157.4851178187871312, 15.19241473665912778, 8.999999999997330136 ) ) ;
#54105=EDGE_LOOP ( 'NONE', ( #76295, #76555, #10779, #18577 ) ) ;
#54117=CARTESIAN_POINT ( 'NONE',  ( 207.7039919494849869, 30.29338434242846390, 15.02863188060213773 ) ) ;
#54121=EDGE_CURVE ( 'NONE', #73562, #75506, #60113, .T. ) ;
#54124=CARTESIAN_POINT ( 'NONE',  ( 206.1705337702867382, 1.000000000000000222, -7.166337341072456901 ) ) ;
#54129=CARTESIAN_POINT ( 'NONE',  ( 208.4306832106270519, 1.063508326895939771, 7.500000000000014211 ) ) ;
#54130=AXIS2_PLACEMENT_3D ( 'NONE', #63746, #48082, #54724 ) ;
#54131=DIRECTION ( 'NONE',  ( 0.000000000000000000, 0.000000000000000000, 1.000000000000000000 ) ) ;
#54134=APPLICATION_CONTEXT ( 'automotive_design' ) ;
#54135=LINE ( 'NONE', #39907, #64999 ) ;
#54138=CARTESIAN_POINT ( 'NONE',  ( 156.5008572375018332, 15.54442400203453190, -9.984260581291959369 ) ) ;
#54140=CARTESIAN_POINT ( 'NONE',  ( 209.7064572754725873, 36.40703279031890816, 14.69807322781363546 ) ) ;
#54153=ORIENTED_EDGE ( 'NONE', *, *, #56330, .F. ) ;
#54176=CARTESIAN_POINT ( 'NONE',  ( 164.2231345125756263, 293.9636489450775230, 0.000000000000000000 ) ) ;
#54189=ORIENTED_EDGE ( 'NONE', *, *, #31528, .T. ) ;
#54191=EDGE_CURVE ( 'NONE', #49322, #86359, #63635, .T. ) ;
#54214=VERTEX_POINT ( 'NONE', #82695 ) ;
#54221=CARTESIAN_POINT ( 'NONE',  ( 151.0356227160792173, 20.07892719424426531, -6.469110745567457244 ) ) ;
#54222=EDGE_CURVE ( 'NONE', #70758, #44168, #44270, .T. ) ;
#54227=CARTESIAN_POINT ( 'NONE',  ( 197.3748232817348764, 214.9910457053126720, -12.45182892472558756 ) ) ;
#54235=CARTESIAN_POINT ( 'NONE',  ( 153.9124347780988558, 19.64445381522117273, -13.06493381020000477 ) ) ;
#54241=CARTESIAN_POINT ( 'NONE',  ( 199.2180164324846885, 65.99917555505274436, 9.231954786409863445 ) ) ;
#54248=CARTESIAN_POINT ( 'NONE',  ( 180.0056393205866812, 275.0000000000000568, -23.52000000000002800 ) ) ;
#54254=DIRECTION ( 'NONE',  ( 0.000000000000000000, 0.000000000000000000, 1.000000000000000000 ) ) ;
#54281=CARTESIAN_POINT ( 'NONE',  ( 197.3296566515638517, 72.17749256844233230, 11.72628858667597740 ) ) ;
#54283=DIRECTION ( 'NONE',  ( 0.000000000000000000, 1.000000000000000000, 0.000000000000000000 ) ) ;
#54295=DIRECTION ( 'NONE',  ( -1.000000000000000000, 0.000000000000000000, 0.000000000000000000 ) ) ;
#54304=DIRECTION ( 'NONE',  ( 1.000000000000000000, 0.000000000000000000, 0.000000000000000000 ) ) ;
#54305=CARTESIAN_POINT ( 'NONE',  ( 157.4851178187871312, 1.000000000000000000, 10.00000000000000000 ) ) ;
#54309=ORIENTED_EDGE ( 'NONE', *, *, #24971, .T. ) ;
#54326=EDGE_CURVE ( 'NONE', #75749, #47327, #66088, .T. ) ;
#54328=VECTOR ( 'NONE', #27747, 1000.000000000000000 ) ;
#54337=DIRECTION ( 'NONE',  ( 1.000000000000000000, 0.000000000000000000, -2.940294503956655304E-16 ) ) ;
#54340=ORIENTED_EDGE ( 'NONE', *, *, #89067, .F. ) ;
#54344=EDGE_CURVE ( 'NONE', #78327, #93327, #48802, .T. ) ;
#54354=ADVANCED_FACE ( 'NONE', ( #45187 ), #47050, .F. ) ;
#54357=DIRECTION ( 'NONE',  ( -0.000000000000000000, 1.000000000000000000, -0.000000000000000000 ) ) ;
#54371=CARTESIAN_POINT ( 'NONE',  ( 158.6539576904058606, 293.9636489450775230, 0.000000000000000000 ) ) ;
#54377=DIRECTION ( 'NONE',  ( 0.000000000000000000, 0.000000000000000000, -1.000000000000000000 ) ) ;
#54390=ORIENTED_EDGE ( 'NONE', *, *, #91848, .T. ) ;
#54391=CYLINDRICAL_SURFACE ( 'NONE', #34806, 0.5000000000000004441 ) ;
#54393=CARTESIAN_POINT ( 'NONE',  ( 189.9243309297870610, 275.0000000000000568, 20.22542485937349355 ) ) ;
#54394=AXIS2_PLACEMENT_3D ( 'NONE', #39435, #67889, #3012 ) ;
#54407=CARTESIAN_POINT ( 'NONE',  ( 197.8536156918379447, 70.38469146215045669, -8.282373351500920577 ) ) ;
#54408=EDGE_CURVE ( 'NONE', #60602, #12757, #22753, .T. ) ;
#54411=ORIENTED_EDGE ( 'NONE', *, *, #81790, .F. ) ;
#54416=CARTESIAN_POINT ( 'NONE',  ( 195.8632375102449146, 25.05079320569620904, 14.11692515535455783 ) ) ;
#54433=ORIENTED_EDGE ( 'NONE', *, *, #34294, .T. ) ;
#54439=CARTESIAN_POINT ( 'NONE',  ( 200.8419735307467420, 26.78103457774644269, 10.49999999999999822 ) ) ;
#54450=CARTESIAN_POINT ( 'NONE',  ( 159.4851178187871312, 15.00000000000000000, -7.000000000000000888 ) ) ;
#54454=ADVANCED_FACE ( 'NONE', ( #47531 ), #9085, .T. ) ;
#54456=VECTOR ( 'NONE', #30538, 1000.000000000000000 ) ;
#54460=CARTESIAN_POINT ( 'NONE',  ( 195.4781563537916043, 250.0000000000000568, 15.50000000000000000 ) ) ;
#54462=VECTOR ( 'NONE', #12840, 1000.000000000000000 ) ;
#54472=EDGE_CURVE ( 'NONE', #2308, #13829, #83505, .T. ) ;
#54473=DIRECTION ( 'NONE',  ( 0.000000000000000000, 0.000000000000000000, -1.000000000000000000 ) ) ;
#54483=CYLINDRICAL_SURFACE ( 'NONE', #33572, 0.5000000000000000000 ) ;
#54485=CARTESIAN_POINT ( 'NONE',  ( 201.4395141301528724, 287.8627056969148725, -5.175264492474406453 ) ) ;
#54487=DIRECTION ( 'NONE',  ( 0.000000000000000000, 1.000000000000000000, 0.000000000000000000 ) ) ;
#54499=DIRECTION ( 'NONE',  ( -0.5000000000000046629, 0.8660254037844359321, 0.000000000000000000 ) ) ;
#54542=ORIENTED_EDGE ( 'NONE', *, *, #21877, .T. ) ;
#54561=ORIENTED_EDGE ( 'NONE', *, *, #34825, .F. ) ;
#54584=CARTESIAN_POINT ( 'NONE',  ( 207.2843595876404095, 1.043152431597805130, -7.415392722555414373 ) ) ;
#54587=EDGE_CURVE ( 'NONE', #30213, #63820, #40849, .T. ) ;
#54590=CARTESIAN_POINT ( 'NONE',  ( 153.3663770037547636, 20.33084388956512001, 12.12609372516293327 ) ) ;
#54592=AXIS2_PLACEMENT_3D ( 'NONE', #60711, #17620, #46471 ) ;
#54594=CARTESIAN_POINT ( 'NONE',  ( 156.5440870305766055, 214.9910457053126720, 17.21343741151179429 ) ) ;
#54597=CARTESIAN_POINT ( 'NONE',  ( 200.5815643859949944, 65.97596549932491428, 9.780880230328994784 ) ) ;
#54599=CARTESIAN_POINT ( 'NONE',  ( 155.2898987420118431, 20.78850644404472092, 13.36622507082863187 ) ) ;
#54611=ORIENTED_EDGE ( 'NONE', *, *, #14110, .F. ) ;
#54614=DIRECTION ( 'NONE',  ( 0.000000000000000000, 0.000000000000000000, 1.000000000000000000 ) ) ;
#54616=EDGE_LOOP ( 'NONE', ( #29304, #11520, #92861, #36943, #71109, #11485, #43709, #35197, #37390, #58866, #25012 ) ) ;
#54633=CARTESIAN_POINT ( 'NONE',  ( 175.2296996224749250, 250.5000000000000568, -29.99999999999998224 ) ) ;
#54651=EDGE_LOOP ( 'NONE', ( #8915, #47920, #91180, #89127 ) ) ;
#54661=VECTOR ( 'NONE', #1618, 1000.000000000000000 ) ;
#54669=AXIS2_PLACEMENT_3D ( 'NONE', #68948, #11638, #10225 ) ;
#54674=ORIENTED_EDGE ( 'NONE', *, *, #9906, .F. ) ;
#54676=ORIENTED_EDGE ( 'NONE', *, *, #60013, .F. ) ;
#54683=CARTESIAN_POINT ( 'NONE',  ( 175.2296996224750103, 133.0000000000000000, 0.000000000000000000 ) ) ;
#54687=CARTESIAN_POINT ( 'NONE',  ( 195.7226947101956682, 20.87406718349393486, -14.32264105795935372 ) ) ;
#54695=CARTESIAN_POINT ( 'NONE',  ( 196.7383257810085979, 24.47698789593438917, 11.00000000000000000 ) ) ;
#54700=CARTESIAN_POINT ( 'NONE',  ( 196.2775035532951335, 71.85522536017060702, 11.57408223790024060 ) ) ;
#54705=CARTESIAN_POINT ( 'NONE',  ( 175.2296996224750103, 249.5000000000000568, -12.00000000000000000 ) ) ;
#54713=DIRECTION ( 'NONE',  ( 0.000000000000000000, 0.000000000000000000, -1.000000000000000000 ) ) ;
#54717=VECTOR ( 'NONE', #15928, 1000.000000000000000 ) ;
#54724=DIRECTION ( 'NONE',  ( -1.000000000000000000, 0.000000000000000000, 0.000000000000000000 ) ) ;
#54727=CARTESIAN_POINT ( 'NONE',  ( 169.9462594094670180, 250.0000000000000568, -23.92352941176469727 ) ) ;
#54741=EDGE_LOOP ( 'NONE', ( #78676, #45446, #63676, #22895 ) ) ;
#54742=CARTESIAN_POINT ( 'NONE',  ( 165.2494399300530290, 8.542400036368780647, -9.000000000000001776 ) ) ;
#54744=CARTESIAN_POINT ( 'NONE',  ( 207.8987101828041375, 29.19759012196911740, 13.45150321557463791 ) ) ;
#54748=ADVANCED_FACE ( 'NONE', ( #60371 ), #52970, .T. ) ;
#54755=VERTEX_POINT ( 'NONE', #18198 ) ;
#54756=ORIENTED_EDGE ( 'NONE', *, *, #53943, .T. ) ;
#54757=CARTESIAN_POINT ( 'NONE',  ( 139.6539576904058606, 275.0000000000000568, 10.50000000000000000 ) ) ;
#54766=B_SPLINE_CURVE_WITH_KNOTS ( 'NONE', 3,
 ( #12579, #92555, #77921, #91628, #5945, #34356, #32940, #26781 ),
 .UNSPECIFIED., .F., .F.,
 ( 4, 2, 2, 4 ),
 ( 0.000000000000000000, 0.0004363303908676402477, 0.0008726607817352804953, 0.001745321563470476857 ),
 .UNSPECIFIED. ) ;
#54767=CARTESIAN_POINT ( 'NONE',  ( 202.9738562182569694, 293.9636489450776367, -54.00000000000000000 ) ) ;
#54772=ORIENTED_EDGE ( 'NONE', *, *, #29167, .F. ) ;
#54781=ORIENTED_EDGE ( 'NONE', *, *, #57468, .F. ) ;
#54800=AXIS2_PLACEMENT_3D ( 'NONE', #59576, #29757, #67602 ) ;
#54801=CARTESIAN_POINT ( 'NONE',  ( 196.9906426852887193, 73.09784627861046147, -12.30894099459319513 ) ) ;
#54805=DIRECTION ( 'NONE',  ( 0.000000000000000000, 0.000000000000000000, -1.000000000000000000 ) ) ;
#54819=DIRECTION ( 'NONE',  ( -0.000000000000000000, -0.000000000000000000, -1.000000000000000000 ) ) ;
#54832=DIRECTION ( 'NONE',  ( 0.000000000000000000, 0.000000000000000000, -1.000000000000000000 ) ) ;
#54834=DIRECTION ( 'NONE',  ( 0.000000000000000000, 1.000000000000000000, 0.000000000000000000 ) ) ;
#54843=DIRECTION ( 'NONE',  ( 0.000000000000000000, 0.000000000000000000, 1.000000000000000000 ) ) ;
#54849=EDGE_CURVE ( 'NONE', #52994, #24040, #75686, .T. ) ;
#54851=CIRCLE ( 'NONE', #14063, 25.50000000000000355 ) ;
#54855=AXIS2_PLACEMENT_3D ( 'NONE', #49567, #27812, #85550 ) ;
#54857=CARTESIAN_POINT ( 'NONE',  ( 206.6110726073805210, 0.01288801604375346306, -7.290233312756247308 ) ) ;
#54861=CIRCLE ( 'NONE', #6498, 21.95310499597075804 ) ;
#54864=AXIS2_PLACEMENT_3D ( 'NONE', #32398, #83029, #55582 ) ;
#54869=EDGE_LOOP ( 'NONE', ( #13888, #76823, #93003, #92775 ) ) ;
#54877=VERTEX_POINT ( 'NONE', #39950 ) ;
#54881=CARTESIAN_POINT ( 'NONE',  ( 197.1159755554518256, 25.84677204156019314, 12.26097734572891795 ) ) ;
#54882=CARTESIAN_POINT ( 'NONE',  ( 195.3593974516954006, 25.91226055734827582, 14.82602457198997747 ) ) ;
#54891=CIRCLE ( 'NONE', #83608, 0.5000000000000004441 ) ;
#54892=ORIENTED_EDGE ( 'NONE', *, *, #42128, .F. ) ;
#54893=ADVANCED_FACE ( 'NONE', ( #45651 ), #13734, .T. ) ;
#54902=ORIENTED_EDGE ( 'NONE', *, *, #43587, .F. ) ;
#54903=CARTESIAN_POINT ( 'NONE',  ( 165.2424497756046549, 250.0000000000000568, 22.91843887563435445 ) ) ;
#54908=CARTESIAN_POINT ( 'NONE',  ( 200.2110226547167429, 26.62113606806761013, 10.50000000000112799 ) ) ;
#54919=CARTESIAN_POINT ( 'NONE',  ( 208.6208076322478746, 32.98517505407394168, 9.000000000000001776 ) ) ;
#54921=VECTOR ( 'NONE', #93602, 1000.000000000000000 ) ;
#54930=CIRCLE ( 'NONE', #62531, 5.000000000000000888 ) ;
#54936=VECTOR ( 'NONE', #49029, 1000.000000000000000 ) ;
#54944=AXIS2_PLACEMENT_3D ( 'NONE', #8593, #87654, #72549 ) ;
#54945=DIRECTION ( 'NONE',  ( 1.000000000000000000, -0.000000000000000000, 0.000000000000000000 ) ) ;
#54948=B_SPLINE_CURVE_WITH_KNOTS ( 'NONE', 3,
 ( #16517, #30259, #30730, #59151, #38748, #73363 ),
 .UNSPECIFIED., .F., .F.,
 ( 4, 2, 4 ),
 ( -4.472146915482244616E-06, 0.0003332253989338073027, 0.0006709229447830969287 ),
 .UNSPECIFIED. ) ;
#54951=CIRCLE ( 'NONE', #14092, 0.4999999999999999445 ) ;
#54959=AXIS2_PLACEMENT_3D ( 'NONE', #82352, #37849, #2367 ) ;
#54960=CARTESIAN_POINT ( 'NONE',  ( 0.000000000000000000, 0.000000000000000000, -9.000000000000001776 ) ) ;
#54962=CARTESIAN_POINT ( 'NONE',  ( 139.1539576904058606, 250.5000000000000568, 10.50000000000000000 ) ) ;
#54963=DIRECTION ( 'NONE',  ( 0.000000000000000000, 1.000000000000000000, -0.000000000000000000 ) ) ;
#54974=ORIENTED_EDGE ( 'NONE', *, *, #17688, .F. ) ;
#54991=DIRECTION ( 'NONE',  ( 0.000000000000000000, 0.000000000000000000, -1.000000000000000000 ) ) ;
#54992=EDGE_CURVE ( 'NONE', #24992, #33695, #34873, .T. ) ;
#54994=CARTESIAN_POINT ( 'NONE',  ( 189.4188515237862589, 293.9636489450775798, -40.00000000000000711 ) ) ;
#55004=CIRCLE ( 'NONE', #58077, 0.5000000000000004441 ) ;
#55010=VERTEX_POINT ( 'NONE', #54633 ) ;
#55012=ORIENTED_EDGE ( 'NONE', *, *, #73993, .F. ) ;
#55014=TOROIDAL_SURFACE ( 'NONE', #23317, 1.500000000000001776, 0.5000000000000000000 ) ;
#55017=CIRCLE ( 'NONE', #76180, 24.00000000000000355 ) ;
#55019=CARTESIAN_POINT ( 'NONE',  ( 195.5463244018911269, 20.93879963055986693, -14.58213394506753602 ) ) ;
#55027=CIRCLE ( 'NONE', #79247, 2.000000000000000000 ) ;
#55041=AXIS2_PLACEMENT_3D ( 'NONE', #66642, #74200, #1769 ) ;
#55046=DIRECTION ( 'NONE',  ( 0.000000000000000000, 0.000000000000000000, 1.000000000000000000 ) ) ;
#55050=EDGE_LOOP ( 'NONE', ( #90574, #62159, #62699 ) ) ;
#55062=CARTESIAN_POINT ( 'NONE',  ( 208.1093360985927347, 29.46709201141245060, 14.78642201437206261 ) ) ;
#55070=EDGE_CURVE ( 'NONE', #31130, #17753, #40872, .T. ) ;
#55073=FACE_OUTER_BOUND ( 'NONE', #31835, .T. ) ;
#55074=CARTESIAN_POINT ( 'NONE',  ( 209.2568086740256206, 34.98978593258856051, 12.00000000000000000 ) ) ;
#55079=CARTESIAN_POINT ( 'NONE',  ( 164.5772123382336360, 215.0000000000000568, 23.16839473634451352 ) ) ;
#55081=VERTEX_POINT ( 'NONE', #11556 ) ;
#55083=CARTESIAN_POINT ( 'NONE',  ( 201.2104617360081704, 60.19600395700751250, 9.999999999999998224 ) ) ;
#55095=TOROIDAL_SURFACE ( 'NONE', #50567, 1.000000000000000000, 0.5000000000000000000 ) ;
#55099=EDGE_LOOP ( 'NONE', ( #45437, #78128, #1450, #21046 ) ) ;
#55103=CARTESIAN_POINT ( 'NONE',  ( 207.8064396648212551, 36.74001737686529623, 13.57731244650625690 ) ) ;
#55105=ORIENTED_EDGE ( 'NONE', *, *, #25741, .F. ) ;
#55107=VERTEX_POINT ( 'NONE', #85401 ) ;
#55112=CIRCLE ( 'NONE', #14311, 2.000000000000000000 ) ;
#55122=B_SPLINE_CURVE_WITH_KNOTS ( 'NONE', 3,
 ( #31073, #67051, #73237, #66136 ),
 .UNSPECIFIED., .F., .F.,
 ( 4, 4 ),
 ( 0.000000000000000000, 0.001235754004288067880 ),
 .UNSPECIFIED. ) ;
#55124=DIRECTION ( 'NONE',  ( 0.000000000000000000, 1.000000000000000000, 0.000000000000000000 ) ) ;
#55131=CYLINDRICAL_SURFACE ( 'NONE', #87707, 24.00000000000001066 ) ;
#55137=EDGE_CURVE ( 'NONE', #60346, #68064, #1609, .T. ) ;
#55142=EDGE_LOOP ( 'NONE', ( #79487, #321, #2261, #81784 ) ) ;
#55145=ADVANCED_FACE ( 'NONE', ( #27645 ), #27171, .F. ) ;
#55165=ORIENTED_EDGE ( 'NONE', *, *, #28287, .F. ) ;
#55177=DIRECTION ( 'NONE',  ( 0.9167375550253600291, 0.000000000000000000, -0.3994899938748465162 ) ) ;
#55180=CIRCLE ( 'NONE', #38534, 0.5000000000000004441 ) ;
#55183=CARTESIAN_POINT ( 'NONE',  ( 196.8803347170859865, 24.42324672360809856, 12.49999999999999289 ) ) ;
#55196=EDGE_CURVE ( 'NONE', #20929, #24375, #69322, .T. ) ;
#55198=CARTESIAN_POINT ( 'NONE',  ( 196.7837483607274294, 69.56983351252434034, 10.93883090039470396 ) ) ;
#55202=FACE_OUTER_BOUND ( 'NONE', #84663, .T. ) ;
#55206=DIRECTION ( 'NONE',  ( 0.000000000000000000, 1.000000000000000000, 0.000000000000000000 ) ) ;
#55211=DIRECTION ( 'NONE',  ( -1.000000000000000000, 0.000000000000000000, 0.000000000000000000 ) ) ;
#55224=CARTESIAN_POINT ( 'NONE',  ( 140.6539576904058606, 275.0000000000000568, -11.50000000000000000 ) ) ;
#55252=ORIENTED_EDGE ( 'NONE', *, *, #46092, .T. ) ;
#55262=DIRECTION ( 'NONE',  ( -0.000000000000000000, -1.000000000000000000, -0.000000000000000000 ) ) ;
#55263=CARTESIAN_POINT ( 'NONE',  ( 175.2296996224750103, 250.0000000000000568, 0.000000000000000000 ) ) ;
#55276=EDGE_CURVE ( 'NONE', #68989, #41691, #46478, .T. ) ;
#55282=CARTESIAN_POINT ( 'NONE',  ( 185.4166944662902665, 214.7015631973135044, 22.87680765314684095 ) ) ;
#55283=CARTESIAN_POINT ( 'NONE',  ( 156.5191989162425727, 214.5000000000000568, 16.58062614384861178 ) ) ;
#55284=DIRECTION ( 'NONE',  ( -1.000000000000000000, 0.000000000000000000, 0.000000000000000000 ) ) ;
#55294=CARTESIAN_POINT ( 'NONE',  ( 195.5052121915463772, 42.19797087126539736, 12.84284333379224208 ) ) ;
#55295=EDGE_CURVE ( 'NONE', #7087, #80534, #63188, .T. ) ;
#55297=EDGE_LOOP ( 'NONE', ( #70500, #29083, #3927, #63793 ) ) ;
#55298=EDGE_LOOP ( 'NONE', ( #45832, #20313, #58803, #65803, #32396, #93187 ) ) ;
#55299=CARTESIAN_POINT ( 'NONE',  ( 175.2296996224750103, 249.5000000000000568, 0.000000000000000000 ) ) ;
#55314=DIRECTION ( 'NONE',  ( 0.5000000000000032196, -0.8660254037844368202, 0.000000000000000000 ) ) ;
#55315=ADVANCED_FACE ( 'NONE', ( #21003 ), #9159, .T. ) ;
#55316=CARTESIAN_POINT ( 'NONE',  ( 196.5149767539403172, 40.96976812506227361, 12.79486244754526147 ) ) ;
#55331=FACE_OUTER_BOUND ( 'NONE', #92142, .T. ) ;
#55340=CARTESIAN_POINT ( 'NONE',  ( 195.6816644507675562, 41.22368217153885439, 14.37939295600229528 ) ) ;
#55348=EDGE_LOOP ( 'NONE', ( #48601, #2815, #79528, #82159, #39457, #19070 ) ) ;
#55349=DIRECTION ( 'NONE',  ( 0.000000000000000000, 0.000000000000000000, 1.000000000000000000 ) ) ;
#55351=LINE ( 'NONE', #83267, #48958 ) ;
#55361=ORIENTED_EDGE ( 'NONE', *, *, #39899, .F. ) ;
#55373=CARTESIAN_POINT ( 'NONE',  ( 219.8344101925596021, 35.72494958537217968, -7.000000000000000888 ) ) ;
#55374=CARTESIAN_POINT ( 'NONE',  ( 196.2268097803946318, 25.02946980243403985, 13.57081821020089585 ) ) ;
#55384=AXIS2_PLACEMENT_3D ( 'NONE', #38225, #72383, #7500 ) ;
#55393=ORIENTED_EDGE ( 'NONE', *, *, #6101, .F. ) ;
#55394=CARTESIAN_POINT ( 'NONE',  ( 156.1711712139736505, 21.00000000000000000, -14.59590564729795226 ) ) ;
#55410=CARTESIAN_POINT ( 'NONE',  ( 193.6552470326849402, 275.5000000000000568, 16.89672165344822119 ) ) ;
#55434=CARTESIAN_POINT ( 'NONE',  ( 208.4306832106271088, 0.04196010845015941959, 7.500000000000013323 ) ) ;
#55442=PLANE ( 'NONE',  #19927 ) ;
#55444=LINE ( 'NONE', #93171, #76185 ) ;
#55456=ORIENTED_EDGE ( 'NONE', *, *, #24948, .T. ) ;
#55461=AXIS2_PLACEMENT_3D ( 'NONE', #52901, #7957, #878 ) ;
#55472=( BOUNDED_SURFACE ( )  B_SPLINE_SURFACE ( 3, 2, ( 
 ( #74509, #51438, #3476 ),
 ( #81604, #9640, #25254 ),
 ( #16752, #39903, #68824 ),
 ( #3954, #15011, #45607 ),
 ( #43870, #38527, #7890 ),
 ( #84866, #34237, #47482 ) ),
 .UNSPECIFIED., .F., .F., .F. ) 
 B_SPLINE_SURFACE_WITH_KNOTS ( ( 4, 2, 4 ),
 ( 3, 3 ),
 ( -1.292368989602721285E-16, 0.001862880473700399137, 0.003725760947400927510 ),
 ( 0.000000000000000000, 1.000000000000000000 ),
 .UNSPECIFIED. ) 
 GEOMETRIC_REPRESENTATION_ITEM ( )  RATIONAL_B_SPLINE_SURFACE ( (
 ( 1.000000000000000000, 0.7071067811865238140, 1.000000000000000000),
 ( 1.000000000000000000, 0.7252627170954408786, 1.000000000000000000),
 ( 1.000000000000000000, 0.7411712618955165199, 1.000000000000000000),
 ( 1.000000000000000000, 0.7689234021729055568, 1.000000000000000000),
 ( 1.000000000000000000, 0.7808378870534314897, 1.000000000000000000),
 ( 1.000000000000000000, 0.7905694150420944366, 1.000000000000000000) ) ) 
 REPRESENTATION_ITEM ( '' )  SURFACE ( )  );
#55474=CARTESIAN_POINT ( 'NONE',  ( 138.6539576904058606, 275.0000000000000568, -10.49999999999999822 ) ) ;
#55475=LINE ( 'NONE', #19474, #87375 ) ;
#55489=ORIENTED_EDGE ( 'NONE', *, *, #90062, .F. ) ;
#55491=ORIENTED_EDGE ( 'NONE', *, *, #27827, .F. ) ;
#55492=TOROIDAL_SURFACE ( 'NONE', #47890, 2.500000000000009770, 0.5000000000000000000 ) ;
#55514=ORIENTED_EDGE ( 'NONE', *, *, #75328, .F. ) ;
#55522=CARTESIAN_POINT ( 'NONE',  ( 169.2744399300530347, 8.542400036368780647, 10.00000000000000000 ) ) ;
#55526=VERTEX_POINT ( 'NONE', #84444 ) ;
#55527=EDGE_CURVE ( 'NONE', #88648, #41136, #1682, .T. ) ;
#55534=FACE_OUTER_BOUND ( 'NONE', #41508, .T. ) ;
#55539=DIRECTION ( 'NONE',  ( -0.000000000000000000, -1.000000000000000000, -0.000000000000000000 ) ) ;
#55550=CARTESIAN_POINT ( 'NONE',  ( 156.4851178187871312, 15.00000000000000000, 7.000000000000000888 ) ) ;
#55557=CARTESIAN_POINT ( 'NONE',  ( 193.2782748703399420, 250.0348692542015385, 16.89756558802352870 ) ) ;
#55559=ORIENTED_EDGE ( 'NONE', *, *, #53042, .T. ) ;
#55560=CARTESIAN_POINT ( 'NONE',  ( 155.8055003384352801, 17.52828139914646499, -8.087387968560612705 ) ) ;
#55565=CARTESIAN_POINT ( 'NONE',  ( 156.6530531571843028, 18.17946993580008197, -9.832064661606517930 ) ) ;
#55575=ORIENTED_EDGE ( 'NONE', *, *, #74260, .T. ) ;
#55578=CARTESIAN_POINT ( 'NONE',  ( 207.5211292351690417, 36.67813790105583394, 13.69055975427937000 ) ) ;
#55580=VERTEX_POINT ( 'NONE', #6335 ) ;
#55582=DIRECTION ( 'NONE',  ( 0.000000000000000000, 0.000000000000000000, 1.000000000000000000 ) ) ;
#55610=ORIENTED_EDGE ( 'NONE', *, *, #54326, .T. ) ;
#55613=ORIENTED_EDGE ( 'NONE', *, *, #72108, .T. ) ;
#55616=EDGE_CURVE ( 'NONE', #32542, #69284, #40918, .T. ) ;
#55630=ORIENTED_EDGE ( 'NONE', *, *, #70399, .F. ) ;
#55650=DIRECTION ( 'NONE',  ( 1.000000000000000000, -0.000000000000000000, -0.000000000000000000 ) ) ;
#55657=CARTESIAN_POINT ( 'NONE',  ( 153.6937476593222982, 20.34834636856922430, 12.69848024943771314 ) ) ;
#55660=TOROIDAL_SURFACE ( 'NONE', #58709, 24.49999999999999645, 0.5000000000000000000 ) ;
#55668=DIRECTION ( 'NONE',  ( -0.000000000000000000, -0.000000000000000000, -1.000000000000000000 ) ) ;
#55672=CARTESIAN_POINT ( 'NONE',  ( 200.4972393895363041, 64.43555889006553627, 7.250946725472672050 ) ) ;
#55676=ADVANCED_FACE ( 'NONE', ( #58853 ), #42762, .F. ) ;
#55685=DIRECTION ( 'NONE',  ( -0.000000000000000000, -1.000000000000000000, -0.000000000000000000 ) ) ;
#55688=CARTESIAN_POINT ( 'NONE',  ( 196.1963538710216994, 282.2246705312485915, -40.00000000000000711 ) ) ;
#55706=CARTESIAN_POINT ( 'NONE',  ( 198.4642567341846018, 298.3489338295183302, -6.693632019895620289 ) ) ;
#55716=ORIENTED_EDGE ( 'NONE', *, *, #19155, .F. ) ;
#55726=CARTESIAN_POINT ( 'NONE',  ( 180.5131398354828320, 249.5000000000000568, -23.92352941176472569 ) ) ;
#55740=ORIENTED_EDGE ( 'NONE', *, *, #48576, .T. ) ;
#55746=CARTESIAN_POINT ( 'NONE',  ( 160.5350683151633291, 275.0000000000000568, 20.22542485937379908 ) ) ;
#55747=CARTESIAN_POINT ( 'NONE',  ( 201.2104617360081704, 60.19600395700749829, 10.00000000000000000 ) ) ;
#55748=CARTESIAN_POINT ( 'NONE',  ( 155.4148940283180309, 19.61091623264239558, 11.07022379048214766 ) ) ;
#55757=CARTESIAN_POINT ( 'NONE',  ( 189.9243309297870610, 249.5000000000000568, 20.22542485937349355 ) ) ;
#55759=ORIENTED_EDGE ( 'NONE', *, *, #63139, .T. ) ;
#55760=ORIENTED_EDGE ( 'NONE', *, *, #66040, .T. ) ;
#55761=CARTESIAN_POINT ( 'NONE',  ( 180.6209651459523968, 250.0000000000000568, -24.41176470588237635 ) ) ;
#55776=LINE ( 'NONE', #39197, #23191 ) ;
#55789=ADVANCED_FACE ( 'NONE', ( #36597 ), #80289, .T. ) ;
#55790=CARTESIAN_POINT ( 'NONE',  ( 222.8344101925596306, 0.000000000000000000, -7.000000000000000888 ) ) ;
#55792=LINE ( 'NONE', #33527, #65671 ) ;
#55802=CARTESIAN_POINT ( 'NONE',  ( 195.8576258688865721, 41.78303943026349998, 14.12515198783110826 ) ) ;
#55810=ORIENTED_EDGE ( 'NONE', *, *, #40105, .T. ) ;
#55811=CARTESIAN_POINT ( 'NONE',  ( 152.5497490326716274, 19.93678331745992693, 10.54177645506989514 ) ) ;
#55813=CARTESIAN_POINT ( 'NONE',  ( 202.9738562182569694, 293.9636489450776367, -54.00000000000000000 ) ) ;
#55823=ORIENTED_EDGE ( 'NONE', *, *, #34144, .F. ) ;
#55824=CARTESIAN_POINT ( 'NONE',  ( 194.7276689066472954, 39.51856478053394994, 14.01265887717885050 ) ) ;
#55830=EDGE_LOOP ( 'NONE', ( #60692, #18796, #55610, #73688 ) ) ;
#55834=AXIS2_PLACEMENT_3D ( 'NONE', #33294, #77806, #39912 ) ;
#55838=CARTESIAN_POINT ( 'NONE',  ( 159.4851178187871312, 69.18068689461284748, -7.000000000000000888 ) ) ;
#55842=ORIENTED_EDGE ( 'NONE', *, *, #56649, .F. ) ;
#55843=EDGE_CURVE ( 'NONE', #15987, #4883, #87838, .T. ) ;
#55846=ADVANCED_FACE ( 'NONE', ( #65976 ), #51261, .F. ) ;
#55852=ORIENTED_EDGE ( 'NONE', *, *, #15423, .F. ) ;
#55897=CARTESIAN_POINT ( 'NONE',  ( 200.2296996224750103, 68.12454877784578855, 2.194831983258790586 ) ) ;
#55904=AXIS2_PLACEMENT_3D ( 'NONE', #29110, #70354, #22016 ) ;
#55936=CARTESIAN_POINT ( 'NONE',  ( 185.1905923765118587, 275.0000000000000568, 21.83530662808691503 ) ) ;
#55937=CARTESIAN_POINT ( 'NONE',  ( 185.5586831021499563, 214.8268611780448509, 22.89084223187800049 ) ) ;
#55943=EDGE_CURVE ( 'NONE', #42552, #54877, #19800, .T. ) ;
#55965=AXIS2_PLACEMENT_3D ( 'NONE', #76227, #26971, #68191 ) ;
#55970=DIRECTION ( 'NONE',  ( 0.000000000000000000, 0.000000000000000000, 1.000000000000000000 ) ) ;
#55975=VERTEX_POINT ( 'NONE', #6813 ) ;
#55982=ORIENTED_EDGE ( 'NONE', *, *, #34585, .T. ) ;
#55993=LINE ( 'NONE', #90996, #8187 ) ;
#56010=CARTESIAN_POINT ( 'NONE',  ( 175.2296996224750103, 215.0000000000000568, 0.000000000000000000 ) ) ;
#56017=CARTESIAN_POINT ( 'NONE',  ( 200.6103193995254230, 250.0000000000000568, -2.464576988612307229 ) ) ;
#56018=ADVANCED_FACE ( 'NONE', ( #93427 ), #89317, .T. ) ;
#56020=( BOUNDED_CURVE ( )  B_SPLINE_CURVE ( 3, ( #60591, #47268, #91297, #19348 ),
 .UNSPECIFIED., .F., .F. ) 
 B_SPLINE_CURVE_WITH_KNOTS ( ( 4, 4 ),
 ( 6.022196528194273313, 6.283185307179586232 ),
 .UNSPECIFIED. ) 
 CURVE ( )  GEOMETRIC_REPRESENTATION_ITEM ( )  RATIONAL_B_SPLINE_CURVE ( ( 1.000000000000000000, 0.9943317885200936290, 0.9943317885200936290, 1.000000000000000000 ) ) 
 REPRESENTATION_ITEM ( '' )  );
#56021=CARTESIAN_POINT ( 'NONE',  ( 200.4738562182569694, 293.9636489450776367, -54.00000000000000000 ) ) ;
#56031=( BOUNDED_SURFACE ( )  B_SPLINE_SURFACE ( 3, 2, ( 
 ( #62784, #69382, #34345 ),
 ( #4514, #54235, #39530 ),
 ( #47110, #33391, #61822 ),
 ( #76017, #84049, #4989 ),
 ( #19195, #75551, #12087 ),
 ( #90206, #48054, #18257 ) ),
 .UNSPECIFIED., .F., .F., .F. ) 
 B_SPLINE_SURFACE_WITH_KNOTS ( ( 4, 2, 4 ),
 ( 3, 3 ),
 ( 0.006706248180543205976, 0.007337862909626279365, 0.007969477638709351885 ),
 ( 0.000000000000000000, 1.000000000000000000 ),
 .UNSPECIFIED. ) 
 GEOMETRIC_REPRESENTATION_ITEM ( )  RATIONAL_B_SPLINE_SURFACE ( (
 ( 1.000000000000000000, 0.7791885400064301193, 1.000000000000000000),
 ( 1.000000000000000000, 0.7898969217198510417, 1.000000000000000000),
 ( 1.000000000000000000, 0.7999169422268818108, 1.000000000000000000),
 ( 1.000000000000000000, 0.8184003267333962439, 1.000000000000000000),
 ( 1.000000000000000000, 0.8267394355353160362, 1.000000000000000000),
 ( 1.000000000000000000, 0.8333723006562909763, 1.000000000000000000) ) ) 
 REPRESENTATION_ITEM ( '' )  SURFACE ( )  );
#56035=AXIS2_PLACEMENT_3D ( 'NONE', #74794, #18894, #47749 ) ;
#56036=VERTEX_POINT ( 'NONE', #44623 ) ;
#56038=AXIS2_PLACEMENT_3D ( 'NONE', #16775, #52292, #1638 ) ;
#56042=ORIENTED_EDGE ( 'NONE', *, *, #32302, .F. ) ;
#56056=EDGE_CURVE ( 'NONE', #23662, #17402, #12228, .T. ) ;
#56059=DIRECTION ( 'NONE',  ( -1.000000000000000000, 0.000000000000000000, 0.000000000000000000 ) ) ;
#56067=DIRECTION ( 'NONE',  ( -0.7453559924999217934, 0.000000000000000000, -0.6666666666666758445 ) ) ;
#56075=ORIENTED_EDGE ( 'NONE', *, *, #19615, .T. ) ;
#56078=ORIENTED_EDGE ( 'NONE', *, *, #13000, .F. ) ;
#56081=ADVANCED_FACE ( 'NONE', ( #43694 ), #29968, .T. ) ;
#56096=ORIENTED_EDGE ( 'NONE', *, *, #49490, .T. ) ;
#56102=ORIENTED_EDGE ( 'NONE', *, *, #19615, .F. ) ;
#56109=AXIS2_PLACEMENT_3D ( 'NONE', #35204, #64133, #92967 ) ;
#56113=LINE ( 'NONE', #48042, #3352 ) ;
#56126=FACE_OUTER_BOUND ( 'NONE', #23482, .T. ) ;
#56131=DIRECTION ( 'NONE',  ( 0.000000000000000000, 0.000000000000000000, 1.000000000000000000 ) ) ;
#56134=LINE ( 'NONE', #20142, #17911 ) ;
#56137=DIRECTION ( 'NONE',  ( 0.000000000000000000, 0.000000000000000000, 1.000000000000000000 ) ) ;
#56138=DIRECTION ( 'NONE',  ( 0.000000000000000000, 0.000000000000000000, -1.000000000000000000 ) ) ;
#56142=EDGE_CURVE ( 'NONE', #77260, #54214, #28579, .T. ) ;
#56152=CARTESIAN_POINT ( 'NONE',  ( 186.6539576904058890, 293.9636489450775230, 0.000000000000000000 ) ) ;
#56168=ADVANCED_FACE ( 'NONE', ( #29517 ), #58397, .F. ) ;
#56173=CARTESIAN_POINT ( 'NONE',  ( 198.3053063117764907, 298.1794517842361643, -6.802035004563411924 ) ) ;
#56183=ORIENTED_EDGE ( 'NONE', *, *, #27622, .T. ) ;
#56184=ORIENTED_EDGE ( 'NONE', *, *, #27047, .T. ) ;
#56189=ADVANCED_FACE ( 'NONE', ( #21464 ), #157, .T. ) ;
#56195=DIRECTION ( 'NONE',  ( 0.000000000000000000, 0.000000000000000000, -1.000000000000000000 ) ) ;
#56196=CYLINDRICAL_SURFACE ( 'NONE', #78031, 2.000000000000000000 ) ;
#56213=ORIENTED_EDGE ( 'NONE', *, *, #60067, .T. ) ;
#56216=CARTESIAN_POINT ( 'NONE',  ( 155.0601170292805193, 20.95974790765944107, -14.78042489204667120 ) ) ;
#56217=EDGE_CURVE ( 'NONE', #39182, #49216, #47008, .T. ) ;
#56218=DIRECTION ( 'NONE',  ( 0.000000000000000000, 1.000000000000000000, 0.000000000000000000 ) ) ;
#56224=CARTESIAN_POINT ( 'NONE',  ( 208.2166030336615563, 27.61833517603036725, 14.22786471510347184 ) ) ;
#56225=LINE ( 'NONE', #49574, #45584 ) ;
#56227=EDGE_LOOP ( 'NONE', ( #32429, #43280, #13207, #77734 ) ) ;
#56228=ORIENTED_EDGE ( 'NONE', *, *, #82755, .T. ) ;
#56238=VECTOR ( 'NONE', #66130, 1000.000000000000000 ) ;
#56245=CARTESIAN_POINT ( 'NONE',  ( 196.9534188175200029, 25.84350552936208700, 12.42857142857141817 ) ) ;
#56246=CARTESIAN_POINT ( 'NONE',  ( 207.3481610410795213, 36.16742558173439193, 14.95883904121434682 ) ) ;
#56263=DIRECTION ( 'NONE',  ( 0.9693563597868444237, 0.2456588035076248677, 0.000000000000000000 ) ) ;
#56275=CARTESIAN_POINT ( 'NONE',  ( 196.4497209205300692, 41.67145302791455208, 13.67271671015795675 ) ) ;
#56283=ORIENTED_EDGE ( 'NONE', *, *, #53042, .F. ) ;
#56284=CARTESIAN_POINT ( 'NONE',  ( 150.4957602436334696, 20.00000000000000355, 3.637614988394419324 ) ) ;
#56296=ORIENTED_EDGE ( 'NONE', *, *, #67159, .F. ) ;
#56297=DIRECTION ( 'NONE',  ( 0.000000000000000000, 0.000000000000000000, 1.000000000000000000 ) ) ;
#56307=AXIS2_PLACEMENT_3D ( 'NONE', #18245, #60874, #89253 ) ;
#56309=CARTESIAN_POINT ( 'NONE',  ( 198.0020767287909962, 65.94727227685316961, -9.918438920559909278 ) ) ;
#56310=AXIS2_PLACEMENT_3D ( 'NONE', #53921, #9895, #68135 ) ;
#56312=CARTESIAN_POINT ( 'NONE',  ( 197.8941236165608473, 42.00370313906616104, 9.707778735729039710 ) ) ;
#56323=ORIENTED_EDGE ( 'NONE', *, *, #54849, .T. ) ;
#56330=EDGE_CURVE ( 'NONE', #43712, #34296, #73971, .T. ) ;
#56333=LINE ( 'NONE', #12788, #19659 ) ;
#56349=DIRECTION ( 'NONE',  ( 0.000000000000000000, 0.000000000000000000, 1.000000000000000000 ) ) ;
#56357=DIRECTION ( 'NONE',  ( 0.000000000000000000, 0.000000000000000000, 1.000000000000000000 ) ) ;
#56360=EDGE_CURVE ( 'NONE', #12543, #64179, #77247, .T. ) ;
#56364=DIRECTION ( 'NONE',  ( 0.000000000000000000, 1.000000000000000000, 0.000000000000000000 ) ) ;
#56372=DIRECTION ( 'NONE',  ( -0.000000000000000000, -0.000000000000000000, 1.000000000000000000 ) ) ;
#56374=FACE_OUTER_BOUND ( 'NONE', #61772, .T. ) ;
#56378=AXIS2_PLACEMENT_3D ( 'NONE', #5091, #60523, #26860 ) ;
#56386=EDGE_CURVE ( 'NONE', #20929, #39726, #36433, .T. ) ;
#56388=AXIS2_PLACEMENT_3D ( 'NONE', #57622, #86945, #22097 ) ;
#56402=ORIENTED_EDGE ( 'NONE', *, *, #54344, .F. ) ;
#56405=CARTESIAN_POINT ( 'NONE',  ( 208.4306832106271088, 0.000000000000000000, 0.000000000000000000 ) ) ;
#56411=AXIS2_PLACEMENT_3D ( 'NONE', #33199, #69192, #70144 ) ;
#56419=CARTESIAN_POINT ( 'NONE',  ( 164.6329196456214277, 250.5000000000000568, 23.09031830825856346 ) ) ;
#56432=ORIENTED_EDGE ( 'NONE', *, *, #93286, .T. ) ;
#56434=CIRCLE ( 'NONE', #73049, 0.5000000000000004441 ) ;
#56446=AXIS2_PLACEMENT_3D ( 'NONE', #23132, #52015, #80901 ) ;
#56456=VERTEX_POINT ( 'NONE', #37965 ) ;
#56458=AXIS2_PLACEMENT_3D ( 'NONE', #73622, #59893, #46117 ) ;
#56462=EDGE_CURVE ( 'NONE', #73850, #44442, #31896, .T. ) ;
#56477=DIRECTION ( 'NONE',  ( 0.000000000000000000, 0.000000000000000000, -1.000000000000000000 ) ) ;
#56479=AXIS2_PLACEMENT_3D ( 'NONE', #37259, #81272, #73720 ) ;
#56490=CIRCLE ( 'NONE', #5029, 9.550761578869391144 ) ;
#56496=CARTESIAN_POINT ( 'NONE',  ( 196.0143093133015384, 20.19615242270662847, 11.99999999999998934 ) ) ;
#56497=CARTESIAN_POINT ( 'NONE',  ( 208.4306832106271088, 20.44233620800389772, 0.000000000000000000 ) ) ;
#56503=EDGE_CURVE ( 'NONE', #48026, #87609, #81981, .T. ) ;
#56510=DIRECTION ( 'NONE',  ( 1.000000000000000000, 0.000000000000000000, -0.000000000000000000 ) ) ;
#56521=EDGE_CURVE ( 'NONE', #83682, #24951, #70031, .T. ) ;
#56526=CARTESIAN_POINT ( 'NONE',  ( 175.2296996224750103, 154.6894116713782807, 20.15985230015483154 ) ) ;
#56528=ORIENTED_EDGE ( 'NONE', *, *, #30594, .T. ) ;
#56532=CIRCLE ( 'NONE', #35358, 0.9999999999999955591 ) ;
#56543=VECTOR ( 'NONE', #92618, 1000.000000000000114 ) ;
#56553=ADVANCED_FACE ( 'NONE', ( #74430 ), #25180, .F. ) ;
#56555=CARTESIAN_POINT ( 'NONE',  ( 199.7700033442230279, 63.22432295887225706, 10.15684170342042236 ) ) ;
#56561=VECTOR ( 'NONE', #91666, 1000.000000000000000 ) ;
#56583=ORIENTED_EDGE ( 'NONE', *, *, #20778, .T. ) ;
#56589=ORIENTED_EDGE ( 'NONE', *, *, #17514, .F. ) ;
#56605=DIRECTION ( 'NONE',  ( 0.000000000000000000, 1.000000000000000000, 0.000000000000000000 ) ) ;
#56614=DIRECTION ( 'NONE',  ( 0.000000000000000000, 1.000000000000000000, 0.000000000000000000 ) ) ;
#56619=DIRECTION ( 'NONE',  ( -0.000000000000000000, 1.000000000000000000, -0.000000000000000000 ) ) ;
#56623=DIRECTION ( 'NONE',  ( 0.7484200282493165268, 0.000000000000000000, 0.6632250457539224930 ) ) ;
#56627=CARTESIAN_POINT ( 'NONE',  ( 197.0790555737925445, 71.90044526202932218, -12.15580537966067354 ) ) ;
#56640=CYLINDRICAL_SURFACE ( 'NONE', #82844, 25.00000000000000355 ) ;
#56643=DIRECTION ( 'NONE',  ( -0.6056179655966478226, 0.7957555401921982963, -0.000000000000000000 ) ) ;
#56649=EDGE_CURVE ( 'NONE', #86001, #91341, #30406, .T. ) ;
#56671=ORIENTED_EDGE ( 'NONE', *, *, #28405, .F. ) ;
#56675=AXIS2_PLACEMENT_3D ( 'NONE', #65377, #36934, #66741 ) ;
#56682=CARTESIAN_POINT ( 'NONE',  ( 199.4392256788250677, 65.82574266882504332, 7.741079165001067963 ) ) ;
#56696=EDGE_LOOP ( 'NONE', ( #13112, #88651, #32304, #3219 ) ) ;
#56700=VERTEX_POINT ( 'NONE', #75375 ) ;
#56701=LINE ( 'NONE', #33968, #82463 ) ;
#56702=DIRECTION ( 'NONE',  ( 0.000000000000000000, 0.000000000000000000, -1.000000000000000000 ) ) ;
#56710=CARTESIAN_POINT ( 'NONE',  ( 201.2929949297285077, 65.04117685566218654, -7.250946725472672938 ) ) ;
#56712=ORIENTED_EDGE ( 'NONE', *, *, #26148, .F. ) ;
#56713=ORIENTED_EDGE ( 'NONE', *, *, #26684, .F. ) ;
#56718=EDGE_CURVE ( 'NONE', #64817, #30244, #10488, .T. ) ;
#56743=EDGE_CURVE ( 'NONE', #3669, #77618, #13798, .T. ) ;
#56745=EDGE_CURVE ( 'NONE', #9610, #40624, #25863, .T. ) ;
#56746=CARTESIAN_POINT ( 'NONE',  ( 151.2975037349265790, 130.0000000000000568, -12.50000000000000000 ) ) ;
#56763=CARTESIAN_POINT ( 'NONE',  ( 195.6044778036177547, 41.09067717743725723, 14.48841315576171951 ) ) ;
#56772=VERTEX_POINT ( 'NONE', #5174 ) ;
#56775=CARTESIAN_POINT ( 'NONE',  ( 158.6539576904058606, 276.0000000000000568, 11.60392986742922616 ) ) ;
#56784=ORIENTED_EDGE ( 'NONE', *, *, #69037, .F. ) ;
#56785=CARTESIAN_POINT ( 'NONE',  ( 194.4860589715128185, 40.74925082751673955, 14.32478396798074805 ) ) ;
#56796=DIRECTION ( 'NONE',  ( 1.000000000000000000, 0.000000000000000000, 0.000000000000000000 ) ) ;
#56829=AXIS2_PLACEMENT_3D ( 'NONE', #51876, #80303, #9246 ) ;
#56834=ORIENTED_EDGE ( 'NONE', *, *, #1219, .F. ) ;
#56850=DIRECTION ( 'NONE',  ( 0.000000000000000000, 1.000000000000000000, 0.000000000000000000 ) ) ;
#56859=FACE_OUTER_BOUND ( 'NONE', #42056, .T. ) ;
#56870=FACE_OUTER_BOUND ( 'NONE', #89596, .T. ) ;
#56872=ADVANCED_FACE ( 'NONE', ( #20773 ), #9233, .T. ) ;
#56873=CARTESIAN_POINT ( 'NONE',  ( 197.9854405158082784, 69.89761265382871613, -11.10143562203536582 ) ) ;
#56881=EDGE_CURVE ( 'NONE', #3669, #50859, #19829, .T. ) ;
#56885=DIRECTION ( 'NONE',  ( -0.8660254037844410391, 0.000000000000000000, -0.4999999999999960032 ) ) ;
#56900=DIRECTION ( 'NONE',  ( -0.000000000000000000, -1.000000000000000000, -0.000000000000000000 ) ) ;
#56901=CARTESIAN_POINT ( 'NONE',  ( 157.7238125175282732, 19.47471017779398750, 10.32097897594415059 ) ) ;
#56914=ORIENTED_EDGE ( 'NONE', *, *, #82272, .T. ) ;
#56929=CARTESIAN_POINT ( 'NONE',  ( 165.0427047786672290, 249.5000000000000568, 23.37680765314704701 ) ) ;
#56930=EDGE_CURVE ( 'NONE', #24992, #49098, #48696, .T. ) ;
#56935=ORIENTED_EDGE ( 'NONE', *, *, #49001, .T. ) ;
#56943=CARTESIAN_POINT ( 'NONE',  ( 199.0061125298537377, 215.0000000000000568, -7.725424859374024678 ) ) ;
#56953=DIRECTION ( 'NONE',  ( -1.110223024625156383E-14, 0.000000000000000000, 1.000000000000000000 ) ) ;
#56969=CARTESIAN_POINT ( 'NONE',  ( 189.9243309297870610, 250.5000000000000568, 20.22542485937349355 ) ) ;
#56970=CARTESIAN_POINT ( 'NONE',  ( 153.7618860799040590, 19.60619416575235263, 12.81536571218043719 ) ) ;
#56978=CARTESIAN_POINT ( 'NONE',  ( 199.0743954165634761, 275.0000000000000568, -2.725891136377211144 ) ) ;
#56981=DIRECTION ( 'NONE',  ( -0.000000000000000000, -1.000000000000000000, -0.000000000000000000 ) ) ;
#56982=CARTESIAN_POINT ( 'NONE',  ( 157.4851178187871312, 15.28877977928703658, -6.999999999998999023 ) ) ;
#56992=EDGE_LOOP ( 'NONE', ( #53705, #24618, #58615, #44639, #82212, #22888, #72806, #51742, #10981, #48988, #77880, #88615, #1003, #53828, #73104, #23911, #1131, #36634, #78129 ) ) ;
#56995=CARTESIAN_POINT ( 'NONE',  ( 175.2296996224749250, 275.0000000000000568, -29.99999999999998224 ) ) ;
#56997=ORIENTED_EDGE ( 'NONE', *, *, #10314, .T. ) ;
#56999=ORIENTED_EDGE ( 'NONE', *, *, #56718, .F. ) ;
#57008=CIRCLE ( 'NONE', #67593, 5.568361562975243650 ) ;
#57022=LINE ( 'NONE', #34750, #21359 ) ;
#57029=VERTEX_POINT ( 'NONE', #21235 ) ;
#57032=EDGE_LOOP ( 'NONE', ( #56999, #3174, #73074, #33121, #68763, #85187 ) ) ;
#57049=EDGE_CURVE ( 'NONE', #61449, #45666, #77320, .T. ) ;
#57052=EDGE_LOOP ( 'NONE', ( #16654, #44899, #26873, #65424 ) ) ;
#57067=DIRECTION ( 'NONE',  ( 0.000000000000000000, 1.000000000000000000, 0.000000000000000000 ) ) ;
#57072=LINE ( 'NONE', #28640, #26348 ) ;
#57078=DIRECTION ( 'NONE',  ( 0.000000000000000000, 0.000000000000000000, 1.000000000000000000 ) ) ;
#57085=CARTESIAN_POINT ( 'NONE',  ( 208.6208076322478746, 32.98517505407394168, 15.00000000000000000 ) ) ;
#57105=DIRECTION ( 'NONE',  ( -0.2156506209390900430, 0.000000000000000000, -0.9764705882352960886 ) ) ;
#57131=ORIENTED_EDGE ( 'NONE', *, *, #67705, .T. ) ;
#57142=LINE ( 'NONE', #85983, #18724 ) ;
#57147=ORIENTED_EDGE ( 'NONE', *, *, #72919, .F. ) ;
#57151=ADVANCED_FACE ( 'NONE', ( #85161 ), #59057, .T. ) ;
#57156=ORIENTED_EDGE ( 'NONE', *, *, #60783, .F. ) ;
#57160=ORIENTED_EDGE ( 'NONE', *, *, #79357, .F. ) ;
#57161=CARTESIAN_POINT ( 'NONE',  ( 157.4970531492008661, 250.0000000000000568, 16.90571646082702983 ) ) ;
#57162=CARTESIAN_POINT ( 'NONE',  ( 155.3778607292159677, 20.99999999999999645, -15.20506116941400165 ) ) ;
#57170=PLANE ( 'NONE',  #59357 ) ;
#57171=DIRECTION ( 'NONE',  ( 0.000000000000000000, 0.000000000000000000, 1.000000000000000000 ) ) ;
#57175=FACE_OUTER_BOUND ( 'NONE', #48130, .T. ) ;
#57189=CARTESIAN_POINT ( 'NONE',  ( 140.6539576904058606, 249.5000000000000568, -10.49999999999999822 ) ) ;
#57203=DIRECTION ( 'NONE',  ( 0.000000000000000000, 0.000000000000000000, 1.000000000000000000 ) ) ;
#57212=PLANE ( 'NONE',  #86721 ) ;
#57229=ORIENTED_EDGE ( 'NONE', *, *, #16334, .F. ) ;
#57230=CARTESIAN_POINT ( 'NONE',  ( 189.9243309297870610, 275.5000000000000568, 20.22542485937349355 ) ) ;
#57232=DIRECTION ( 'NONE',  ( 0.000000000000000000, 0.000000000000000000, 1.000000000000000000 ) ) ;
#57241=EDGE_LOOP ( 'NONE', ( #5181, #84592, #91534, #9315 ) ) ;
#57248=EDGE_CURVE ( 'NONE', #75719, #7041, #23081, .T. ) ;
#57249=ORIENTED_EDGE ( 'NONE', *, *, #90014, .F. ) ;
#57255=CARTESIAN_POINT ( 'NONE',  ( 196.2775840954750208, 71.85475162903931334, -11.57395220326623964 ) ) ;
#57265=ORIENTED_EDGE ( 'NONE', *, *, #44269, .F. ) ;
#57272=ADVANCED_FACE ( 'NONE', ( #81770 ), #43924, .T. ) ;
#57275=VERTEX_POINT ( 'NONE', #30198 ) ;
#57276=CIRCLE ( 'NONE', #10322, 25.00000000000000355 ) ;
#57291=EDGE_LOOP ( 'NONE', ( #85326, #90368, #4135, #3198, #87233 ) ) ;
#57292=EDGE_LOOP ( 'NONE', ( #16965, #89466, #2949, #68532 ) ) ;
#57307=DIRECTION ( 'NONE',  ( 0.5370370370370221025, -0.000000000000000000, 0.8435586647355927115 ) ) ;
#57308=CARTESIAN_POINT ( 'NONE',  ( 180.6209651459523968, 250.5000000000000568, -24.41176470588238345 ) ) ;
#57320=CARTESIAN_POINT ( 'NONE',  ( 152.1970976711774597, 130.7369940202023884, 11.50000000000000178 ) ) ;
#57329=CARTESIAN_POINT ( 'NONE',  ( 194.7453183674696220, 20.99999999999998934, 15.62500000000049205 ) ) ;
#57331=CARTESIAN_POINT ( 'NONE',  ( 197.0505512480903008, 72.68507397627607247, -12.20517631820067272 ) ) ;
#57342=CIRCLE ( 'NONE', #86022, 0.5000000000000014433 ) ;
#57344=ORIENTED_EDGE ( 'NONE', *, *, #24741, .F. ) ;
#57347=FACE_OUTER_BOUND ( 'NONE', #64149, .T. ) ;
#57358=DIRECTION ( 'NONE',  ( -0.000000000000000000, 1.000000000000000000, -0.000000000000000000 ) ) ;
#57359=DIRECTION ( 'NONE',  ( 0.000000000000000000, 1.000000000000000000, 0.000000000000000000 ) ) ;
#57360=EDGE_CURVE ( 'NONE', #67960, #72522, #66653, .T. ) ;
#57371=EDGE_LOOP ( 'NONE', ( #4372, #63819, #10538, #27425, #17199 ) ) ;
#57380=ORIENTED_EDGE ( 'NONE', *, *, #60977, .T. ) ;
#57386=DIRECTION ( 'NONE',  ( 0.8620390091940283162, 0.000000000000000000, -0.5068419345592647396 ) ) ;
#57398=CARTESIAN_POINT ( 'NONE',  ( 195.9255997734375683, 26.17269670437365647, 13.45023288292440711 ) ) ;
#57404=CIRCLE ( 'NONE', #81550, 5.103083949679981579 ) ;
#57415=DIRECTION ( 'NONE',  ( -0.7806247497997887974, 0.000000000000000000, 0.6250000000000137668 ) ) ;
#57433=CARTESIAN_POINT ( 'NONE',  ( 165.2424497756046549, 250.5000000000000568, 22.91843887563435800 ) ) ;
#57438=CARTESIAN_POINT ( 'NONE',  ( 195.8564219449220616, 25.05878860812877562, 14.12689474711300086 ) ) ;
#57454=EDGE_LOOP ( 'NONE', ( #92298, #89944, #75739, #68189 ) ) ;
#57463=ORIENTED_EDGE ( 'NONE', *, *, #17448, .F. ) ;
#57468=EDGE_CURVE ( 'NONE', #13227, #23700, #30479, .T. ) ;
#57470=CARTESIAN_POINT ( 'NONE',  ( 170.7304434856092143, 250.5000000000000568, -24.91818181818181088 ) ) ;
#57473=AXIS2_PLACEMENT_3D ( 'NONE', #3312, #47791, #32201 ) ;
#57506=VERTEX_POINT ( 'NONE', #40073 ) ;
#57512=ORIENTED_EDGE ( 'NONE', *, *, #39378, .F. ) ;
#57514=EDGE_CURVE ( 'NONE', #85888, #86239, #75817, .T. ) ;
#57515=ORIENTED_EDGE ( 'NONE', *, *, #15094, .F. ) ;
#57524=DIRECTION ( 'NONE',  ( 0.000000000000000000, 0.000000000000000000, 1.000000000000000000 ) ) ;
#57533=VECTOR ( 'NONE', #43911, 1000.000000000000000 ) ;
#57546=CARTESIAN_POINT ( 'NONE',  ( 198.5111534495024159, 66.01618214920664229, -10.78140162895428666 ) ) ;
#57561=EDGE_CURVE ( 'NONE', #49742, #73850, #75613, .T. ) ;
#57596=FACE_OUTER_BOUND ( 'NONE', #21508, .T. ) ;
#57599=CIRCLE ( 'NONE', #12161, 1.000000000000000888 ) ;
#57613=CARTESIAN_POINT ( 'NONE',  ( 165.2688068684385883, 250.0000000000000568, 21.83530662808711398 ) ) ;
#57616=CARTESIAN_POINT ( 'NONE',  ( 155.8109286537083733, 19.19772955881940391, 9.232252220100694018 ) ) ;
#57622=CARTESIAN_POINT ( 'NONE',  ( 0.000000000000000000, 0.000000000000000000, -7.500000000000000000 ) ) ;
#57642=CARTESIAN_POINT ( 'NONE',  ( 195.8262106289358258, 26.26158389346358746, 13.54803344068640314 ) ) ;
#57643=DIRECTION ( 'NONE',  ( -0.000000000000000000, -1.000000000000000000, -0.000000000000000000 ) ) ;
#57656=CYLINDRICAL_SURFACE ( 'NONE', #3297, 2.000000000000000000 ) ;
#57659=ADVANCED_BREP_SHAPE_REPRESENTATION ( '', ( #26626, #27724, #18940 ), #37050 ) ;
#57669=EDGE_CURVE ( 'NONE', #65802, #56772, #51611, .T. ) ;
#57675=LINE ( 'NONE', #2585, #14074 ) ;
#57685=EDGE_LOOP ( 'NONE', ( #90605, #46390, #17638, #46250, #77406 ) ) ;
#57686=CARTESIAN_POINT ( 'NONE',  ( 200.5815643859950512, 65.97596549932490007, 9.780880230328994784 ) ) ;
#57688=DIRECTION ( 'NONE',  ( -0.000000000000000000, -1.000000000000000000, -0.000000000000000000 ) ) ;
#57697=ORIENTED_EDGE ( 'NONE', *, *, #48992, .F. ) ;
#57698=CARTESIAN_POINT ( 'NONE',  ( 195.8598878520694200, 40.68233701717534956, 13.45727524496615324 ) ) ;
#57704=EDGE_LOOP ( 'NONE', ( #43004, #70659, #54309, #18591 ) ) ;
#57710=FACE_OUTER_BOUND ( 'NONE', #89350, .T. ) ;
#57712=CARTESIAN_POINT ( 'NONE',  ( 139.4823848151520735, 130.0000000000000568, -12.50000000000000000 ) ) ;
#57715=ORIENTED_EDGE ( 'NONE', *, *, #47694, .F. ) ;
#57731=CIRCLE ( 'NONE', #86419, 6.000000000000005329 ) ;
#57733=CIRCLE ( 'NONE', #81829, 4.499999999999993783 ) ;
#57744=CIRCLE ( 'NONE', #32032, 4.999999999999985789 ) ;
#57747=VERTEX_POINT ( 'NONE', #47656 ) ;
#57748=VERTEX_POINT ( 'NONE', #82708 ) ;
#57765=CARTESIAN_POINT ( 'NONE',  ( 200.1126601882107252, 214.5000000000000568, -2.416251949619908856 ) ) ;
#57775=CARTESIAN_POINT ( 'NONE',  ( 175.2296996224750103, 250.5000000000000568, 0.000000000000000000 ) ) ;
#57777=CARTESIAN_POINT ( 'NONE',  ( 199.6702811234769115, 65.52214591209386185, 9.100946541886349550 ) ) ;
#57788=CARTESIAN_POINT ( 'NONE',  ( 196.9830144044668430, 72.62791770022455751, -12.32215356455109578 ) ) ;
#57789=CARTESIAN_POINT ( 'NONE',  ( 207.4724402404595196, 29.73442829110643615, 14.90057469441958560 ) ) ;
#57795=EDGE_CURVE ( 'NONE', #19033, #92829, #32543, .T. ) ;
#57798=VECTOR ( 'NONE', #42349, 1000.000000000000000 ) ;
#57814=CARTESIAN_POINT ( 'NONE',  ( 200.7065524281981936, 64.16053070458296759, -8.800381594948186503 ) ) ;
#57854=DIRECTION ( 'NONE',  ( 0.000000000000000000, 1.000000000000000000, 0.000000000000000000 ) ) ;
#57870=AXIS2_PLACEMENT_3D ( 'NONE', #21911, #71646, #79212 ) ;
#57872=AXIS2_PLACEMENT_3D ( 'NONE', #35379, #44317, #73229 ) ;
#57879=EDGE_CURVE ( 'NONE', #85558, #52800, #38686, .T. ) ;
#57887=CYLINDRICAL_SURFACE ( 'NONE', #41050, 7.999911143031724237 ) ;
#57892=CARTESIAN_POINT ( 'NONE',  ( 195.0943219309016001, 27.07095573865049332, 15.17888833493343270 ) ) ;
#57901=EDGE_CURVE ( 'NONE', #47569, #10831, #46710, .T. ) ;
#57902=EDGE_CURVE ( 'NONE', #65856, #75719, #60695, .T. ) ;
#57907=CARTESIAN_POINT ( 'NONE',  ( 222.8344101925596306, 0.000000000000000000, 7.000000000000000000 ) ) ;
#57909=ORIENTED_EDGE ( 'NONE', *, *, #70691, .F. ) ;
#57922=CARTESIAN_POINT ( 'NONE',  ( 196.8102870837257967, 295.2234712781319104, -7.903912273553234336 ) ) ;
#57925=DIRECTION ( 'NONE',  ( 0.000000000000000000, 1.000000000000000000, 0.000000000000000000 ) ) ;
#57926=AXIS2_PLACEMENT_3D ( 'NONE', #70235, #27599, #34236 ) ;
#57928=AXIS2_PLACEMENT_3D ( 'NONE', #34209, #18586, #48387 ) ;
#57966=EDGE_LOOP ( 'NONE', ( #17964, #91296, #39618, #24873 ) ) ;
#57970=AXIS2_PLACEMENT_3D ( 'NONE', #45892, #51594, #22719 ) ;
#57978=ORIENTED_EDGE ( 'NONE', *, *, #3303, .T. ) ;
#57988=DIRECTION ( 'NONE',  ( -1.000000000000000000, 0.000000000000000000, -0.000000000000000000 ) ) ;
#57993=CARTESIAN_POINT ( 'NONE',  ( 209.3673903755802428, 36.49853773373599353, 14.70256938371377586 ) ) ;
#57994=CIRCLE ( 'NONE', #32279, 0.5000000000000004441 ) ;
#58000=CARTESIAN_POINT ( 'NONE',  ( 155.3770881450913066, 21.00000000067704065, 15.20409621215158147 ) ) ;
#58001=CIRCLE ( 'NONE', #64029, 1.000000000000000888 ) ;
#58003=VECTOR ( 'NONE', #69142, 1000.000000000000000 ) ;
#58009=DIRECTION ( 'NONE',  ( 1.000000000000000000, 0.000000000000000000, 0.000000000000000000 ) ) ;
#58017=AXIS2_PLACEMENT_3D ( 'NONE', #4758, #33638, #62548 ) ;
#58026=CARTESIAN_POINT ( 'NONE',  ( 170.0287519320418426, 214.7033776542919270, -24.48382199637804391 ) ) ;
#58033=AXIS2_PLACEMENT_3D ( 'NONE', #3639, #18784, #17392 ) ;
#58035=ADVANCED_FACE ( 'NONE', ( #17859 ), #40983, .T. ) ;
#58069=TOROIDAL_SURFACE ( 'NONE', #17228, 2.103083949679977582, 2.000000000000000000 ) ;
#58077=AXIS2_PLACEMENT_3D ( 'NONE', #5252, #91389, #10910 ) ;
#58084=EDGE_LOOP ( 'NONE', ( #10048, #34761, #80647, #38102, #66781, #81203 ) ) ;
#58086=FACE_OUTER_BOUND ( 'NONE', #19281, .T. ) ;
#58087=AXIS2_PLACEMENT_3D ( 'NONE', #88494, #8945, #45384 ) ;
#58088=AXIS2_PLACEMENT_3D ( 'NONE', #27788, #64726, #14043 ) ;
#58096=PLANE ( 'NONE',  #56388 ) ;
#58098=CARTESIAN_POINT ( 'NONE',  ( 189.9243309297870610, 276.0000000000000568, 24.72542485937349710 ) ) ;
#58101=CIRCLE ( 'NONE', #3679, 2.000000000000000000 ) ;
#58119=CARTESIAN_POINT ( 'NONE',  ( 195.4888831047267104, 26.84972106461252039, 13.90636001966099222 ) ) ;
#58120=DIRECTION ( 'NONE',  ( -0.6056179655966479336, 0.7957555401921982963, 0.000000000000000000 ) ) ;
#58133=DIRECTION ( 'NONE',  ( 0.000000000000000000, 1.000000000000000000, 0.000000000000000000 ) ) ;
#58141=DIRECTION ( 'NONE',  ( 0.000000000000000000, 1.000000000000000000, 0.000000000000000000 ) ) ;
#58144=CARTESIAN_POINT ( 'NONE',  ( 219.8344101925596021, 35.72494958537217968, 10.00000000000000000 ) ) ;
#58146=AXIS2_PLACEMENT_3D ( 'NONE', #69519, #61956, #34012 ) ;
#58155=VECTOR ( 'NONE', #54087, 1000.000000000000000 ) ;
#58161=VECTOR ( 'NONE', #24793, 1000.000000000000000 ) ;
#58163=CARTESIAN_POINT ( 'NONE',  ( 208.0840766214418522, 28.61636207333354420, 12.00000001296747598 ) ) ;
#58172=AXIS2_PLACEMENT_3D ( 'NONE', #59687, #89920, #45904 ) ;
#58173=EDGE_CURVE ( 'NONE', #91480, #51603, #45612, .T. ) ;
#58175=ORIENTED_EDGE ( 'NONE', *, *, #8991, .T. ) ;
#58176=CARTESIAN_POINT ( 'NONE',  ( 195.4218348477629092, 41.23934650999667895, 12.97788390064105712 ) ) ;
#58187=CARTESIAN_POINT ( 'NONE',  ( 196.8324751178603833, 70.49344883866203304, -10.86630005027734569 ) ) ;
#58198=ORIENTED_EDGE ( 'NONE', *, *, #907, .T. ) ;
#58208=CARTESIAN_POINT ( 'NONE',  ( 175.2296996224750103, 250.5000000000000568, 24.50000000000000355 ) ) ;
#58215=EDGE_CURVE ( 'NONE', #39726, #27101, #1162, .T. ) ;
#58227=CIRCLE ( 'NONE', #61263, 0.4999999999999935052 ) ;
#58239=CARTESIAN_POINT ( 'NONE',  ( 198.5394373321410342, 68.65923120348695363, -9.381478303811002561 ) ) ;
#58240=DIRECTION ( 'NONE',  ( 0.000000000000000000, 0.000000000000000000, 1.000000000000000000 ) ) ;
#58251=CYLINDRICAL_SURFACE ( 'NONE', #5146, 2.842139515347646750 ) ;
#58252=CLOSED_SHELL ( 'NONE', ( #92683, #58529, #90026, #25257, #82147, #87034, #77003, #41191, #43816, #59205, #67596, #52132, #31682, #31341, #15433, #72327, #17993, #66836, #30221, #41631, #18149, #4837, #5502, #24859, #86183, #51223, #21442, #76775, #45395, #13225, #66737, #13052, #43859, #77537, #70288, #84146, #53185, #52625, #10271, #38489, #56018, #13841, #10942, #29646, #62814, #90829, #14803, #72008, #28527, #38335, #56081, #79860, #64861, #1631, #83076, #59271, #28927, #22669, #76783, #68498, #85346, #38195, #74144, #58937, #85166, #32454, #75267, #44377, #42814, #52270, #30630, #4958, #6973, #92890, #21416, #48436, #46300, #37222, #40296, #7788, #63117, #91854, #3675, #2609, #38970, #63476, #48568, #16586, #82928, #52756, #61417, #71813, #50812, #54454, #68562, #42940, #1831, #17782, #87868, #56189, #2812, #7211, #10178, #63535, #54893, #30283, #48700, #72456, #1134, #85699, #52089, #2312, #75605, #13400, #68094, #8314, #53290, #40719, #1014, #1892, #31175, #67429, #32951, #13626, #45549, #27900, #6143, #8827, #64547, #30099, #59617, #36576, #61256, #90539, #71036, #55846, #77210, #69195, #84997, #76515, #76454, #20466, #63995, #73159, #24600, #81252, #92708, #32311, #89888, #40950, #41758, #30720, #42458, #55145, #66216, #35093, #65915, #47478, #93660, #24690, #92039, #53415, #70885, #58322, #20933, #35611, #84860, #23761, #40192, #53824, #58334, #58444, #77562, #34163, #53164, #2434, #87818, #39778, #83171, #74527, #71360, #52694, #19377, #47387, #35478, #60971, #34616, #36344, #89910, #47528, #58505, #78240, #20022, #23916, #7862, #23002, #58035, #37569, #29801, #32709, #15001, #49369, #18678, #78720, #36172, #87961, #17890, #60271, #10599, #8362, #31672, #60568, #32973, #54354, #15807, #52404, #26565, #28586, #1197, #45203, #24208, #34009, #63880, #69560, #69319, #10065, #2313, #68887, #46741, #55315, #54748, #84092, #5848, #84345, #39026, #84672, #37681, #25727, #70112, #26016, #77023, #85344, #60900, #17776, #60144, #56553, #3608, #17677, #55789, #45266, #74804, #3941, #86713, #87240, #84255, #84490, #81481, #252, #65384, #88007, #75532, #5978, #62812, #61198, #59259, #46843, #90425, #69403, #11435, #77948, #42691, #91502, #21708, #62569, #35201, #61331, #59744, #10468, #36645, #60323, #70920, #64764, #87985, #44278, #37625, #6358, #64359, #92926, #79887, #29347, #40830, #34937, #52105, #45119, #25673, #2438, #20581, #20670, #35229, #83283, #67083, #35412, #43303, #67333, #37647, #72625, #21564, #2508, #86068, #89714, #91293, #36378, #26437, #7209, #21734, #39537, #36468, #27856, #45040, #77757, #57151, #71464, #61972, #13104, #49426, #10404, #27767, #89310, #59198, #62917, #22100, #7668, #70518, #64114, #33097, #38716, #47143, #70036, #1421, #44517, #66466, #25489, #87693, #14921, #30229, #83034, #14701, #7949, #47870, #57272, #30159, #91186, #68020, #20124, #77049, #10542, #55676, #14279, #16836, #4299, #81856, #63762, #8974, #3883, #3670, #45140, #49758, #65467, #16602, #56168 ) ) ;
#58266=CARTESIAN_POINT ( 'NONE',  ( 199.8757083317008494, 66.90342950747972850, -8.069961554617966826 ) ) ;
#58276=ORIENTED_EDGE ( 'NONE', *, *, #41871, .T. ) ;
#58290=CARTESIAN_POINT ( 'NONE',  ( 160.5350683151633291, 215.0000000000000568, 20.22542485937379908 ) ) ;
#58291=CARTESIAN_POINT ( 'NONE',  ( 208.6208076322478746, 32.98517505407394168, 10.50000000000000000 ) ) ;
#58302=CIRCLE ( 'NONE', #50718, 5.103083949679981579 ) ;
#58317=CARTESIAN_POINT ( 'NONE',  ( 209.7827226070571385, 36.64741339240061535, 13.08022668053247983 ) ) ;
#58322=ADVANCED_FACE ( 'NONE', ( #10112 ), #78874, .T. ) ;
#58330=EDGE_LOOP ( 'NONE', ( #21872, #34669 ) ) ;
#58331=FACE_OUTER_BOUND ( 'NONE', #83906, .T. ) ;
#58334=ADVANCED_FACE ( 'NONE', ( #9648 ), #13721, .T. ) ;
#58345=DIRECTION ( 'NONE',  ( -0.6250000000000095479, -0.000000000000000000, -0.7806247497997922391 ) ) ;
#58358=DIRECTION ( 'NONE',  ( 0.000000000000000000, 1.000000000000000000, 0.000000000000000000 ) ) ;
#58364=CARTESIAN_POINT ( 'NONE',  ( 152.4536156746142410, 275.0000000000000568, 14.50000000000000000 ) ) ;
#58377=EDGE_LOOP ( 'NONE', ( #78012, #41504, #24595, #55165 ) ) ;
#58380=DIRECTION ( 'NONE',  ( -0.000000000000000000, -1.000000000000000000, -0.000000000000000000 ) ) ;
#58394=CARTESIAN_POINT ( 'NONE',  ( 189.9243309297870610, 250.5000000000000568, 25.22542485937350065 ) ) ;
#58397=CYLINDRICAL_SURFACE ( 'NONE', #24316, 6.286090667950827715 ) ;
#58411=ORIENTED_EDGE ( 'NONE', *, *, #66440, .T. ) ;
#58419=EDGE_CURVE ( 'NONE', #21613, #28948, #53685, .T. ) ;
#58444=ADVANCED_FACE ( 'NONE', ( #26189 ), #33054, .T. ) ;
#58451=EDGE_CURVE ( 'NONE', #65076, #50614, #45588, .T. ) ;
#58455=CARTESIAN_POINT ( 'NONE',  ( 202.9738562182569694, 293.9636489450776367, -44.00000000000000000 ) ) ;
#58460=CARTESIAN_POINT ( 'NONE',  ( 208.4939861239905667, 36.53598741959982732, 14.76870368707861481 ) ) ;
#58469=DIRECTION ( 'NONE',  ( 0.000000000000000000, 0.000000000000000000, 1.000000000000000000 ) ) ;
#58471=CARTESIAN_POINT ( 'NONE',  ( 155.4202369374232262, 19.37982107812039700, -12.54055055082732295 ) ) ;
#58477=CARTESIAN_POINT ( 'NONE',  ( 185.8264795993290477, 215.0000000000000568, 23.09031830825835385 ) ) ;
#58488=CARTESIAN_POINT ( 'NONE',  ( 170.2305261370685798, 214.9910457053126720, -24.90909090909089940 ) ) ;
#58505=ADVANCED_FACE ( 'NONE', ( #3481 ), #39109, .T. ) ;
#58519=( BOUNDED_CURVE ( )  B_SPLINE_CURVE ( 3, ( #34437, #85077, #27331, #34898 ),
 .UNSPECIFIED., .F., .F. ) 
 B_SPLINE_CURVE_WITH_KNOTS ( ( 4, 4 ),
 ( 3.665191429188093597, 4.712388980384689674 ),
 .UNSPECIFIED. ) 
 CURVE ( )  GEOMETRIC_REPRESENTATION_ITEM ( )  RATIONAL_B_SPLINE_CURVE ( ( 1.000000000000000000, 0.9106836025229593234, 0.9106836025229593234, 1.000000000000000000 ) ) 
 REPRESENTATION_ITEM ( '' )  );
#58523=( BOUNDED_SURFACE ( )  B_SPLINE_SURFACE ( 3, 2, ( 
 ( #15255, #73490, #73938 ),
 ( #74397, #81042, #2453 ),
 ( #22814, #73019, #60216 ),
 ( #51683, #23286, #1055 ),
 ( #17589, #16641, #87664 ),
 ( #66388, #2902, #37030 ) ),
 .UNSPECIFIED., .F., .F., .F. ) 
 B_SPLINE_SURFACE_WITH_KNOTS ( ( 4, 2, 4 ),
 ( 3, 3 ),
 ( 4.712388980384689674, 5.132923315668655562, 5.553457650952622338 ),
 ( 0.000000000000000000, 1.000000000000000000 ),
 .UNSPECIFIED. ) 
 GEOMETRIC_REPRESENTATION_ITEM ( )  RATIONAL_B_SPLINE_SURFACE ( (
 ( 1.000000000000000000, 0.7071067811865487940, 1.000000000000000000),
 ( 1.000000000000000000, 0.7192895461638224575, 1.000000000000000000),
 ( 1.000000000000000000, 0.7311219824186969696, 1.000000000000000000),
 ( 1.000000000000000000, 0.7523130761999332616, 1.000000000000000000),
 ( 1.000000000000000000, 0.7616706333086389336, 1.000000000000000000),
 ( 1.000000000000000000, 0.7691239371209216413, 1.000000000000000000) ) ) 
 REPRESENTATION_ITEM ( '' )  SURFACE ( )  );
#58529=ADVANCED_FACE ( 'NONE', ( #49832, #93390 ), #57887, .F. ) ;
#58546=ORIENTED_EDGE ( 'NONE', *, *, #21848, .T. ) ;
#58547=DIRECTION ( 'NONE',  ( 0.000000000000000000, 0.000000000000000000, 1.000000000000000000 ) ) ;
#58549=EDGE_CURVE ( 'NONE', #11198, #89964, #57733, .T. ) ;
#58555=CARTESIAN_POINT ( 'NONE',  ( 155.0601170292804625, 20.95974790765943396, 14.78042489204666587 ) ) ;
#58559=DIRECTION ( 'NONE',  ( 0.000000000000000000, 0.000000000000000000, -1.000000000000000000 ) ) ;
#58563=DIRECTION ( 'NONE',  ( 0.000000000000000000, -1.000000000000000000, 0.000000000000000000 ) ) ;
#58566=EDGE_CURVE ( 'NONE', #6460, #31, #18432, .T. ) ;
#58578=DIRECTION ( 'NONE',  ( 0.000000000000000000, 0.000000000000000000, 1.000000000000000000 ) ) ;
#58587=DIRECTION ( 'NONE',  ( -0.4472135954999804652, 0.4472135955001954599, -0.7745966692413333021 ) ) ;
#58592=DIRECTION ( 'NONE',  ( 0.000000000000000000, 0.000000000000000000, 1.000000000000000000 ) ) ;
#58594=CYLINDRICAL_SURFACE ( 'NONE', #91155, 3.000000000000000000 ) ;
#58603=DIRECTION ( 'NONE',  ( -0.3024135303179465439, -0.9531768234071978929, 0.000000000000000000 ) ) ;
#58615=ORIENTED_EDGE ( 'NONE', *, *, #57902, .F. ) ;
#58627=ORIENTED_EDGE ( 'NONE', *, *, #50291, .F. ) ;
#58637=PLANE ( 'NONE',  #91134 ) ;
#58657=CARTESIAN_POINT ( 'NONE',  ( 158.6539576904058606, 276.0000000000000568, 11.60392986742922616 ) ) ;
#58669=DIRECTION ( 'NONE',  ( 0.000000000000000000, 0.000000000000000000, 1.000000000000000000 ) ) ;
#58674=EDGE_LOOP ( 'NONE', ( #59728, #29494 ) ) ;
#58679=EDGE_CURVE ( 'NONE', #88979, #30715, #6298, .T. ) ;
#58682=VECTOR ( 'NONE', #33418, 1000.000000000000000 ) ;
#58690=CARTESIAN_POINT ( 'NONE',  ( 196.0143093133015384, 42.36571313990103249, 11.99999999999998757 ) ) ;
#58698=FACE_OUTER_BOUND ( 'NONE', #63874, .T. ) ;
#58702=DIRECTION ( 'NONE',  ( 0.000000000000000000, 0.000000000000000000, 1.000000000000000000 ) ) ;
#58709=AXIS2_PLACEMENT_3D ( 'NONE', #66771, #44516, #17043 ) ;
#58727=FACE_BOUND ( 'NONE', #30005, .T. ) ;
#58730=FACE_OUTER_BOUND ( 'NONE', #82938, .T. ) ;
#58734=EDGE_CURVE ( 'NONE', #68290, #307, #6365, .T. ) ;
#58741=ORIENTED_EDGE ( 'NONE', *, *, #21988, .T. ) ;
#58744=CARTESIAN_POINT ( 'NONE',  ( 201.2104617360081704, 60.19600395700752671, -9.000000000000000000 ) ) ;
#58745=DIRECTION ( 'NONE',  ( 0.000000000000000000, 1.000000000000000000, 0.000000000000000000 ) ) ;
#58749=FACE_OUTER_BOUND ( 'NONE', #71330, .T. ) ;
#58766=ORIENTED_EDGE ( 'NONE', *, *, #45672, .F. ) ;
#58773=DIRECTION ( 'NONE',  ( 0.8435586647355688417, 0.000000000000000000, -0.5370370370370596280 ) ) ;
#58785=ORIENTED_EDGE ( 'NONE', *, *, #54006, .F. ) ;
#58786=CARTESIAN_POINT ( 'NONE',  ( 194.9126400680597442, 26.32064278049061912, 13.74612429362717769 ) ) ;
#58796=DIRECTION ( 'NONE',  ( 0.000000000000000000, 0.000000000000000000, 1.000000000000000000 ) ) ;
#58803=ORIENTED_EDGE ( 'NONE', *, *, #1737, .F. ) ;
#58811=CARTESIAN_POINT ( 'NONE',  ( 170.2297021224755724, 215.0000000000000568, -25.00499999999998835 ) ) ;
#58817=CARTESIAN_POINT ( 'NONE',  ( 175.2296996224749250, 250.0000000000000568, -24.99999999999999289 ) ) ;
#58822=CARTESIAN_POINT ( 'NONE',  ( 189.4188515237862589, 293.9636489450775798, 9.103929867429222611 ) ) ;
#58823=CARTESIAN_POINT ( 'NONE',  ( 170.2305261370685798, 215.0000000000000568, -24.90909090909089940 ) ) ;
#58832=ORIENTED_EDGE ( 'NONE', *, *, #30098, .T. ) ;
#58836=CARTESIAN_POINT ( 'NONE',  ( 156.4947056272797852, 20.00000000000000000, 15.00000000000000000 ) ) ;
#58853=FACE_OUTER_BOUND ( 'NONE', #81698, .T. ) ;
#58866=ORIENTED_EDGE ( 'NONE', *, *, #84969, .F. ) ;
#58876=AXIS2_PLACEMENT_3D ( 'NONE', #17129, #87221, #45053 ) ;
#58897=ORIENTED_EDGE ( 'NONE', *, *, #67975, .T. ) ;
#58900=EDGE_LOOP ( 'NONE', ( #38425, #36578, #29412, #78084 ) ) ;
#58910=CARTESIAN_POINT ( 'NONE',  ( 197.4027394742815602, 40.84896208771628068, 12.00000000000000000 ) ) ;
#58915=CARTESIAN_POINT ( 'NONE',  ( 208.3202200382901026, 36.51146326664311914, 14.79041613504217167 ) ) ;
#58921=FACE_OUTER_BOUND ( 'NONE', #9488, .T. ) ;
#58924=LINE ( 'NONE', #51794, #31701 ) ;
#58937=ADVANCED_FACE ( 'NONE', ( #44584 ), #81039, .F. ) ;
#58939=AXIS2_PLACEMENT_3D ( 'NONE', #78177, #13315, #27993 ) ;
#58944=AXIS2_PLACEMENT_3D ( 'NONE', #74047, #9166, #38044 ) ;
#59002=ORIENTED_EDGE ( 'NONE', *, *, #43223, .T. ) ;
#59003=DIRECTION ( 'NONE',  ( 0.3262578496237564796, 0.000000000000000000, 0.9452808130703185263 ) ) ;
#59005=VECTOR ( 'NONE', #19816, 1000.000000000000114 ) ;
#59011=CARTESIAN_POINT ( 'NONE',  ( 140.6539576904058606, 249.5000000000000568, 10.50000000000000000 ) ) ;
#59029=CARTESIAN_POINT ( 'NONE',  ( 153.1588060538193190, 19.71797249535330465, 10.20021433907233899 ) ) ;
#59038=CYLINDRICAL_SURFACE ( 'NONE', #11067, 5.999999999999998224 ) ;
#59046=DIRECTION ( 'NONE',  ( 0.000000000000000000, 0.000000000000000000, 1.000000000000000000 ) ) ;
#59052=CARTESIAN_POINT ( 'NONE',  ( 196.2236821186898794, 42.37849173453419382, 11.63735566334416660 ) ) ;
#59055=CARTESIAN_POINT ( 'NONE',  ( 207.9698821865255525, 1.063508326896293932, 7.500000000000007105 ) ) ;
#59057=( BOUNDED_SURFACE ( )  B_SPLINE_SURFACE ( 3, 2, ( 
 ( #28352, #34516, #27896 ),
 ( #84680, #55824, #78999 ),
 ( #71441, #63423, #86084 ),
 ( #13679, #12751, #50104 ),
 ( #14153, #20314, #93654 ),
 ( #56785, #41592, #92252 ),
 ( #43018, #70514, #49184 ),
 ( #64830, #43473, #13221 ),
 ( #42057, #72370, #35456 ),
 ( #28814, #85627, #57698 ),
 ( #86541, #21711, #7487 ),
 ( #45778, #58176, #9813 ),
 ( #80853, #16000, #72820 ),
 ( #390, #7945, #51961 ),
 ( #37745, #29279, #45306 ),
 ( #87930, #36840, #87018 ) ),
 .UNSPECIFIED., .F., .F., .F. ) 
 B_SPLINE_SURFACE_WITH_KNOTS ( ( 4, 2, 2, 2, 2, 2, 2, 4 ),
 ( 3, 3 ),
 ( 0.000000000000000000, 0.0006169105258908347050, 0.001233821051781669410, 0.001850731577672504007, 0.002467642103563338820, 0.003084552629454173633, 0.003701463155345008013, 0.004935284207126677640 ),
 ( 0.000000000000000000, 1.000000000000000000 ),
 .UNSPECIFIED. ) 
 GEOMETRIC_REPRESENTATION_ITEM ( )  RATIONAL_B_SPLINE_SURFACE ( (
 ( 1.000000000000000000, 0.8966167345234253849, 1.000000000000000000),
 ( 1.000000000000000000, 0.9004139148593394149, 1.000000000000000000),
 ( 1.000000000000000000, 0.9032061010809223633, 1.000000000000000000),
 ( 1.000000000000000000, 0.9067734849426619670, 1.000000000000000000),
 ( 1.000000000000000000, 0.9075308745978637459, 1.000000000000000000),
 ( 1.000000000000000000, 0.9069696504598226960, 1.000000000000000000),
 ( 1.000000000000000000, 0.9056888044671186355, 1.000000000000000000),
 ( 1.000000000000000000, 0.9012558131653337634, 1.000000000000000000),
 ( 1.000000000000000000, 0.8981641526238748341, 1.000000000000000000),
 ( 1.000000000000000000, 0.8905754532997738337, 1.000000000000000000),
 ( 1.000000000000000000, 0.8860218362694791683, 1.000000000000000000),
 ( 1.000000000000000000, 0.8759703649558354677, 1.000000000000000000),
 ( 1.000000000000000000, 0.8704567387601739314, 1.000000000000000000),
 ( 1.000000000000000000, 0.8526573370801874274, 1.000000000000000000),
 ( 1.000000000000000000, 0.8394012181881534973, 1.000000000000000000),
 ( 1.000000000000000000, 0.8255171224912161154, 1.000000000000000000) ) ) 
 REPRESENTATION_ITEM ( '' )  SURFACE ( )  );
#59065=( BOUNDED_CURVE ( )  B_SPLINE_CURVE ( 3, ( #51533, #37788, #16041, #1823 ),
 .UNSPECIFIED., .F., .F. ) 
 B_SPLINE_CURVE_WITH_KNOTS ( ( 4, 4 ),
 ( 0.5235987755983022574, 1.570796326794897224 ),
 .UNSPECIFIED. ) 
 CURVE ( )  GEOMETRIC_REPRESENTATION_ITEM ( )  RATIONAL_B_SPLINE_CURVE ( ( 1.000000000000000000, 0.9106836025229594345, 0.9106836025229594345, 1.000000000000000000 ) ) 
 REPRESENTATION_ITEM ( '' )  );
#59069=EDGE_CURVE ( 'NONE', #38347, #14152, #90998, .T. ) ;
#59070=AXIS2_PLACEMENT_3D ( 'NONE', #54176, #83046, #32871 ) ;
#59073=ORIENTED_EDGE ( 'NONE', *, *, #17361, .F. ) ;
#59087=ORIENTED_EDGE ( 'NONE', *, *, #34052, .F. ) ;
#59092=EDGE_CURVE ( 'NONE', #19714, #15987, #63834, .T. ) ;
#59099=FACE_OUTER_BOUND ( 'NONE', #70562, .T. ) ;
#59100=DIRECTION ( 'NONE',  ( 1.000000000000000000, 0.000000000000000000, -0.000000000000000000 ) ) ;
#59112=VERTEX_POINT ( 'NONE', #29932 ) ;
#59121=CARTESIAN_POINT ( 'NONE',  ( 156.9788746593517033, 250.1588552167596333, 16.89623126087882099 ) ) ;
#59130=CARTESIAN_POINT ( 'NONE',  ( 219.8344101925596021, 35.72494958537217968, -7.000000000000000888 ) ) ;
#59134=VERTEX_POINT ( 'NONE', #51680 ) ;
#59135=ORIENTED_EDGE ( 'NONE', *, *, #92101, .F. ) ;
#59136=CARTESIAN_POINT ( 'NONE',  ( 196.8803347170859865, 42.36571313990103249, 12.49999999999999289 ) ) ;
#59139=EDGE_CURVE ( 'NONE', #55081, #26459, #67319, .T. ) ;
#59151=CARTESIAN_POINT ( 'NONE',  ( 197.0217226327351909, 214.8115906558234371, -12.45424042348861704 ) ) ;
#59152=CARTESIAN_POINT ( 'NONE',  ( 155.1244896729671439, 20.04296953158265993, -14.86678859756603543 ) ) ;
#59160=DIRECTION ( 'NONE',  ( -0.000000000000000000, -1.000000000000000000, -0.000000000000000000 ) ) ;
#59163=DIRECTION ( 'NONE',  ( -1.000000000000000000, 0.000000000000000000, -0.000000000000000000 ) ) ;
#59187=ORIENTED_EDGE ( 'NONE', *, *, #6569, .F. ) ;
#59188=LINE ( 'NONE', #87118, #71047 ) ;
#59191=CARTESIAN_POINT ( 'NONE',  ( 154.1407330040854333, 249.5000000000000568, 13.42592592592592915 ) ) ;
#59198=ADVANCED_FACE ( 'NONE', ( #73487 ), #37929, .T. ) ;
#59205=ADVANCED_FACE ( 'NONE', ( #16183 ), #92511, .T. ) ;
#59206=CARTESIAN_POINT ( 'NONE',  ( 198.6884013828325521, 64.61450673763174279, 9.555809373750800972 ) ) ;
#59209=CARTESIAN_POINT ( 'NONE',  ( 196.1963538710216994, 282.2246705312485915, 13.99999999999999112 ) ) ;
#59246=CARTESIAN_POINT ( 'NONE',  ( 175.2296996224750103, 149.6461846693799487, -24.00000000000001066 ) ) ;
#59259=ADVANCED_FACE ( 'NONE', ( #66837 ), #2449, .F. ) ;
#59264=EDGE_LOOP ( 'NONE', ( #17953, #38993 ) ) ;
#59271=ADVANCED_FACE ( 'NONE', ( #88598 ), #16639, .T. ) ;
#59273=AXIS2_PLACEMENT_3D ( 'NONE', #46989, #61699, #73230 ) ;
#59280=AXIS2_PLACEMENT_3D ( 'NONE', #124, #65482, #15258 ) ;
#59285=CARTESIAN_POINT ( 'NONE',  ( 197.7051530045995094, 41.80213891112349245, 12.00000000000000355 ) ) ;
#59295=EDGE_LOOP ( 'NONE', ( #39735, #10312, #25660, #47300 ) ) ;
#59299=CARTESIAN_POINT ( 'NONE',  ( 195.4709818679464490, 27.30234762113502711, 15.00000000000000000 ) ) ;
#59311=CARTESIAN_POINT ( 'NONE',  ( 156.4851178187871312, 15.24064981607324754, 6.999999999998999023 ) ) ;
#59326=EDGE_CURVE ( 'NONE', #37103, #24392, #16953, .T. ) ;
#59332=VERTEX_POINT ( 'NONE', #53079 ) ;
#59342=ORIENTED_EDGE ( 'NONE', *, *, #27631, .T. ) ;
#59343=AXIS2_PLACEMENT_3D ( 'NONE', #41401, #27701, #70790 ) ;
#59346=AXIS2_PLACEMENT_3D ( 'NONE', #11301, #40154, #69071 ) ;
#59357=AXIS2_PLACEMENT_3D ( 'NONE', #50029, #78923, #14072 ) ;
#59367=EDGE_LOOP ( 'NONE', ( #76666, #79513, #73108, #31697 ) ) ;
#59380=EDGE_CURVE ( 'NONE', #1828, #48224, #47594, .T. ) ;
#59384=DIRECTION ( 'NONE',  ( 0.000000000000000000, -0.000000000000000000, 1.000000000000000000 ) ) ;
#59391=CARTESIAN_POINT ( 'NONE',  ( 175.2296996224750103, 160.0000000000000568, 0.000000000000000000 ) ) ;
#59396=CARTESIAN_POINT ( 'NONE',  ( 221.4259212729440094, 36.93618551656547311, 10.00000000000000000 ) ) ;
#59402=CARTESIAN_POINT ( 'NONE',  ( 197.1123855246551955, 18.41506350946087522, -10.91506350946096759 ) ) ;
#59416=FACE_OUTER_BOUND ( 'NONE', #76339, .T. ) ;
#59418=AXIS2_PLACEMENT_3D ( 'NONE', #29938, #74890, #88605 ) ;
#59420=VECTOR ( 'NONE', #38695, 1000.000000000000000 ) ;
#59424=CIRCLE ( 'NONE', #60898, 0.5000000000000004441 ) ;
#59426=PRODUCT_DEFINITION_SHAPE ( 'NONE', 'NONE',  #74824 ) ;
#59449=AXIS2_PLACEMENT_3D ( 'NONE', #91418, #68731, #40739 ) ;
#59473=VERTEX_POINT ( 'NONE', #90903 ) ;
#59474=CARTESIAN_POINT ( 'NONE',  ( 164.2231345125756263, 276.0000000000000568, 22.80382896337009058 ) ) ;
#59477=B_SPLINE_CURVE_WITH_KNOTS ( 'NONE', 3,
 ( #81712, #82190, #59029, #30146, #44801, #17344, #52377, #87876 ),
 .UNSPECIFIED., .F., .F.,
 ( 4, 2, 2, 4 ),
 ( 0.001027591722192180415, 0.003123856272695763915, 0.005220120823199347199, 0.009412649924206491214 ),
 .UNSPECIFIED. ) ;
#59479=AXIS2_PLACEMENT_3D ( 'NONE', #74994, #1157, #30040 ) ;
#59480=AXIS2_PLACEMENT_3D ( 'NONE', #83799, #83323, #84729 ) ;
#59485=CARTESIAN_POINT ( 'NONE',  ( 205.2296996224750103, 68.12454877777268791, 0.000000000000000000 ) ) ;
#59491=ORIENTED_EDGE ( 'NONE', *, *, #10705, .T. ) ;
#59492=DIRECTION ( 'NONE',  ( 0.000000000000000000, 0.000000000000000000, -1.000000000000000000 ) ) ;
#59494=CIRCLE ( 'NONE', #53463, 25.50000000000000355 ) ;
#59502=B_SPLINE_CURVE_WITH_KNOTS ( 'NONE', 3,
 ( #6051, #63837, #34923, #78488, #71389, #6521, #29221, #86030, #336, #50048, #21652, #14095, #79426, #86964, #22117, #12699, #62071, #46438, #10924, #47842, #54485, #90905, #40724, #28323, #12341, #76281, #19446, #62560, #61159, #4304 ),
 .UNSPECIFIED., .F., .F.,
 ( 4, 2, 2, 2, 2, 2, 2, 2, 2, 2, 2, 2, 2, 2, 4 ),
 ( 0.01214138644550194837, 0.01289762902330727004, 0.01365387160111258998, 0.01441011417891791165, 0.01516635675672323331, 0.01667884191233387492, 0.01743508449013913761, 0.01819132706794440030, 0.01970381222355477649, 0.02046005480135993509, 0.02121629737916509023, 0.02197253995697024537, 0.02272878253477540050, 0.02348502511258055564, 0.02424126769038571078 ),
 .UNSPECIFIED. ) ;
#59510=CIRCLE ( 'NONE', #71628, 2.500000000000002220 ) ;
#59527=DIRECTION ( 'NONE',  ( 0.000000000000000000, 1.000000000000000000, 0.000000000000000000 ) ) ;
#59545=CIRCLE ( 'NONE', #71653, 0.4999999999999947820 ) ;
#59560=CIRCLE ( 'NONE', #79162, 4.999999999999985789 ) ;
#59564=ORIENTED_EDGE ( 'NONE', *, *, #11999, .F. ) ;
#59568=AXIS2_PLACEMENT_3D ( 'NONE', #80455, #39674, #46785 ) ;
#59576=CARTESIAN_POINT ( 'NONE',  ( 175.2296996224750103, 275.5000000000000568, 0.000000000000000000 ) ) ;
#59598=EDGE_CURVE ( 'NONE', #15079, #36764, #44108, .T. ) ;
#59599=DIRECTION ( 'NONE',  ( 0.000000000000000000, 1.000000000000000000, 0.000000000000000000 ) ) ;
#59608=CARTESIAN_POINT ( 'NONE',  ( 207.0561972617101674, 35.35788477359428583, 14.50000000000000000 ) ) ;
#59612=ORIENTED_EDGE ( 'NONE', *, *, #30078, .T. ) ;
#59614=CARTESIAN_POINT ( 'NONE',  ( 196.5975808051812237, 18.84406744235292663, -11.77299963048744047 ) ) ;
#59617=ADVANCED_FACE ( 'NONE', ( #90443 ), #54483, .F. ) ;
#59618=EDGE_CURVE ( 'NONE', #79037, #76858, #9183, .T. ) ;
#59631=DIRECTION ( 'NONE',  ( -0.000000000000000000, -0.000000000000000000, -1.000000000000000000 ) ) ;
#59632=DIRECTION ( 'NONE',  ( 1.000000000000000000, 0.000000000000000000, -0.000000000000000000 ) ) ;
#59645=AXIS2_PLACEMENT_3D ( 'NONE', #64516, #13823, #28493 ) ;
#59647=CARTESIAN_POINT ( 'NONE',  ( 175.2296996224750103, 250.5000000000000568, 0.000000000000000000 ) ) ;
#59661=LINE ( 'NONE', #73841, #6786 ) ;
#59671=ORIENTED_EDGE ( 'NONE', *, *, #39759, .F. ) ;
#59672=DIRECTION ( 'NONE',  ( 0.000000000000000000, 1.000000000000000000, 0.000000000000000000 ) ) ;
#59675=CARTESIAN_POINT ( 'NONE',  ( 164.2231345125756263, 264.6571197653884155, -7.500000000000000000 ) ) ;
#59684=ORIENTED_EDGE ( 'NONE', *, *, #29223, .F. ) ;
#59687=CARTESIAN_POINT ( 'NONE',  ( 208.4306832106271088, 1.000000000000000888, 0.000000000000000000 ) ) ;
#59689=DIRECTION ( 'NONE',  ( -1.000000000000000000, 0.000000000000000000, 0.000000000000000000 ) ) ;
#59700=ORIENTED_EDGE ( 'NONE', *, *, #25372, .T. ) ;
#59709=ORIENTED_EDGE ( 'NONE', *, *, #82280, .F. ) ;
#59716=DIRECTION ( 'NONE',  ( 0.9452808130703184153, -0.000000000000000000, -0.3262578496237564796 ) ) ;
#59724=AXIS2_PLACEMENT_3D ( 'NONE', #48617, #78915, #6022 ) ;
#59728=ORIENTED_EDGE ( 'NONE', *, *, #63164, .T. ) ;
#59738=FACE_OUTER_BOUND ( 'NONE', #16552, .T. ) ;
#59744=ADVANCED_FACE ( 'NONE', ( #46436 ), #55442, .T. ) ;
#59752=CARTESIAN_POINT ( 'NONE',  ( 208.6208076322478746, 32.98517505407394168, 10.00000000000000000 ) ) ;
#59760=CARTESIAN_POINT ( 'NONE',  ( 175.2296996224750103, 134.0000000000000284, 0.000000000000000000 ) ) ;
#59763=CARTESIAN_POINT ( 'NONE',  ( 175.2296996224750103, 249.5000000000000568, 0.000000000000000000 ) ) ;
#59764=CARTESIAN_POINT ( 'NONE',  ( 221.8344101925596306, 1.000000000000000000, 10.00000000000000000 ) ) ;
#59773=ORIENTED_EDGE ( 'NONE', *, *, #78743, .T. ) ;
#59777=CARTESIAN_POINT ( 'NONE',  ( 160.5350683151633291, 250.5000000000000568, 25.22542485937379553 ) ) ;
#59782=AXIS2_PLACEMENT_3D ( 'NONE', #76115, #82278, #68547 ) ;
#59790=CARTESIAN_POINT ( 'NONE',  ( 156.3984609948130071, 15.95758591462568710, 7.138650918358441899 ) ) ;
#59807=VERTEX_POINT ( 'NONE', #76279 ) ;
#59830=ORIENTED_EDGE ( 'NONE', *, *, #69090, .F. ) ;
#59837=ORIENTED_EDGE ( 'NONE', *, *, #38620, .F. ) ;
#59838=CARTESIAN_POINT ( 'NONE',  ( 0.000000000000000000, 0.000000000000000000, -40.00000000000000711 ) ) ;
#59841=ORIENTED_EDGE ( 'NONE', *, *, #80919, .F. ) ;
#59859=CARTESIAN_POINT ( 'NONE',  ( 154.1415209985679269, 20.37991841447901820, -11.45812909362559040 ) ) ;
#59866=CARTESIAN_POINT ( 'NONE',  ( 197.2116943569230045, 215.0000000000000568, -12.92446933126075592 ) ) ;
#59867=B_SPLINE_CURVE_WITH_KNOTS ( 'NONE', 3,
 ( #25449, #39169, #32090, #68081, #61467, #83202, #31177, #45816 ),
 .UNSPECIFIED., .F., .F.,
 ( 4, 2, 2, 4 ),
 ( -8.944277078438763205E-06, 0.001321608365870415719, 0.001986884687344899272, 0.002652161008819382826 ),
 .UNSPECIFIED. ) ;
#59870=CARTESIAN_POINT ( 'NONE',  ( 157.4851178187871312, 17.34719063663031946, -6.999999999999998224 ) ) ;
#59872=CARTESIAN_POINT ( 'NONE',  ( 156.0793278192200830, 19.12150670425148036, -12.12861874973244269 ) ) ;
#59878=DIRECTION ( 'NONE',  ( -0.8660254037844404840, 0.000000000000000000, -0.4999999999999968359 ) ) ;
#59893=DIRECTION ( 'NONE',  ( -0.000000000000000000, -1.000000000000000000, -0.000000000000000000 ) ) ;
#59911=DIRECTION ( 'NONE',  ( 0.000000000000000000, 1.000000000000000000, 0.000000000000000000 ) ) ;
#59917=EDGE_CURVE ( 'NONE', #75628, #89903, #11870, .T. ) ;
#59920=EDGE_CURVE ( 'NONE', #70318, #81225, #69878, .T. ) ;
#59926=ORIENTED_EDGE ( 'NONE', *, *, #5542, .T. ) ;
#59928=VERTEX_POINT ( 'NONE', #62557 ) ;
#59947=CARTESIAN_POINT ( 'NONE',  ( 196.8936505956917244, 70.76315252099192321, -10.57021625195834424 ) ) ;
#59955=CARTESIAN_POINT ( 'NONE',  ( 208.4306832106271088, -74.55766379199613425, 7.500000000000013323 ) ) ;
#59961=CARTESIAN_POINT ( 'NONE',  ( 197.2116943569230330, 275.0000000000000568, -12.92446933126074882 ) ) ;
#59989=FACE_OUTER_BOUND ( 'NONE', #35841, .T. ) ;
#60002=DIRECTION ( 'NONE',  ( 0.000000000000000000, 0.000000000000000000, 1.000000000000000000 ) ) ;
#60013=EDGE_CURVE ( 'NONE', #2870, #83522, #45751, .T. ) ;
#60016=EDGE_LOOP ( 'NONE', ( #87484, #23495, #49536, #4706 ) ) ;
#60017=CARTESIAN_POINT ( 'NONE',  ( 196.8803347170859865, 73.40565171261611965, 12.50000000000000533 ) ) ;
#60030=ORIENTED_EDGE ( 'NONE', *, *, #31052, .F. ) ;
#60040=FACE_OUTER_BOUND ( 'NONE', #42669, .T. ) ;
#60041=CARTESIAN_POINT ( 'NONE',  ( 154.0370857100322723, 19.38211809614433534, -11.97004389447338291 ) ) ;
#60062=CARTESIAN_POINT ( 'NONE',  ( 151.7489156927949807, 20.88249531811356974, 8.613363710899784920 ) ) ;
#60067=EDGE_CURVE ( 'NONE', #68073, #30213, #52514, .T. ) ;
#60072=CARTESIAN_POINT ( 'NONE',  ( 175.2296996224750103, 249.5000000000000568, 0.000000000000000000 ) ) ;
#60077=ORIENTED_EDGE ( 'NONE', *, *, #81073, .T. ) ;
#60078=CARTESIAN_POINT ( 'NONE',  ( 200.1633050441426747, 15.87263057655165532, -10.05743975622730524 ) ) ;
#60092=CARTESIAN_POINT ( 'NONE',  ( 155.7140808774800007, 19.99999999999999645, -15.62500000000000178 ) ) ;
#60100=( LENGTH_UNIT ( ) NAMED_UNIT ( * ) SI_UNIT ( .MILLI., .METRE. ) );
#60104=CARTESIAN_POINT ( 'NONE',  ( 205.7381008070598227, 1.000000000000000888, 7.000000000000000000 ) ) ;
#60106=CARTESIAN_POINT ( 'NONE',  ( 175.2296996224750103, 214.5000000000000568, 0.000000000000000000 ) ) ;
#60113=B_SPLINE_CURVE_WITH_KNOTS ( 'NONE', 3,
 ( #79913, #7932, #54281, #52878, #39579, #61869, #53829, #33437, #88856, #89788 ),
 .UNSPECIFIED., .F., .F.,
 ( 4, 2, 2, 2, 4 ),
 ( -1.751965293301170726E-05, 0.002261625431216393936, 0.004540770515365799044, 0.006819915599515204152, 0.009099060683664610127 ),
 .UNSPECIFIED. ) ;
#60117=CARTESIAN_POINT ( 'NONE',  ( 206.9189553108847122, 30.70889394204684208, 15.00000000000001776 ) ) ;
#60129=FACE_OUTER_BOUND ( 'NONE', #92526, .T. ) ;
#60132=DIRECTION ( 'NONE',  ( 0.000000000000000000, 1.000000000000000000, 0.000000000000000000 ) ) ;
#60140=ORIENTED_EDGE ( 'NONE', *, *, #11778, .T. ) ;
#60143=CARTESIAN_POINT ( 'NONE',  ( 160.5350683151633291, 249.5000000000000568, 20.22542485937379908 ) ) ;
#60144=ADVANCED_FACE ( 'NONE', ( #10352 ), #81951, .T. ) ;
#60149=DIRECTION ( 'NONE',  ( 0.000000000000000000, 0.000000000000000000, 1.000000000000000000 ) ) ;
#60173=CARTESIAN_POINT ( 'NONE',  ( 152.0128028882535034, 20.82798718771465829, -9.301361753755829298 ) ) ;
#60184=ORIENTED_EDGE ( 'NONE', *, *, #44915, .T. ) ;
#60185=CARTESIAN_POINT ( 'NONE',  ( 208.4306832106271088, 0.04196010845015910040, -7.500000000000013323 ) ) ;
#60214=DIRECTION ( 'NONE',  ( -1.000000000000000000, 0.000000000000000000, 0.000000000000000000 ) ) ;
#60216=CARTESIAN_POINT ( 'NONE',  ( 199.8263553767660312, 25.49203953695227653, 10.63455718553152352 ) ) ;
#60219=CARTESIAN_POINT ( 'NONE',  ( 165.2494399300530290, 8.542400036368780647, 10.00000000000000000 ) ) ;
#60220=DIRECTION ( 'NONE',  ( -0.000000000000000000, -1.000000000000000000, -0.000000000000000000 ) ) ;
#60235=CARTESIAN_POINT ( 'NONE',  ( 195.4776723108872716, 27.11938025175527045, 14.98434631268485084 ) ) ;
#60247=DIRECTION ( 'NONE',  ( 0.000000000000000000, 0.000000000000000000, 1.000000000000000000 ) ) ;
#60248=EDGE_CURVE ( 'NONE', #35701, #54214, #50274, .T. ) ;
#60251=DIRECTION ( 'NONE',  ( 0.000000000000000000, 0.000000000000000000, 1.000000000000000000 ) ) ;
#60265=ORIENTED_EDGE ( 'NONE', *, *, #53277, .F. ) ;
#60268=ORIENTED_EDGE ( 'NONE', *, *, #80317, .F. ) ;
#60271=ADVANCED_FACE ( 'NONE', ( #25959 ), #61512, .F. ) ;
#60297=ORIENTED_EDGE ( 'NONE', *, *, #74314, .T. ) ;
#60298=CARTESIAN_POINT ( 'NONE',  ( 159.0442047513580235, 16.98551211945798656, 9.330684800570141491 ) ) ;
#60303=ORIENTED_EDGE ( 'NONE', *, *, #2955, .T. ) ;
#60320=DIRECTION ( 'NONE',  ( 0.000000000000000000, 1.000000000000000000, 0.000000000000000000 ) ) ;
#60323=ADVANCED_FACE ( 'NONE', ( #47256 ), #76169, .T. ) ;
#60330=LINE ( 'NONE', #44224, #10521 ) ;
#60333=CARTESIAN_POINT ( 'NONE',  ( 209.2599468862078140, 293.9636489450776367, -59.00000000000003553 ) ) ;
#60346=VERTEX_POINT ( 'NONE', #4199 ) ;
#60353=CARTESIAN_POINT ( 'NONE',  ( 151.3768371069326690, 130.9657748190496704, -11.49999999999999645 ) ) ;
#60371=FACE_OUTER_BOUND ( 'NONE', #68899, .T. ) ;
#60385=ORIENTED_EDGE ( 'NONE', *, *, #49429, .T. ) ;
#60388=EDGE_CURVE ( 'NONE', #28948, #10184, #65176, .T. ) ;
#60413=CARTESIAN_POINT ( 'NONE',  ( 151.0528680457204018, 20.99319481056665992, -6.529293081333598536 ) ) ;
#60418=CARTESIAN_POINT ( 'NONE',  ( 200.6103193995254230, 275.5000000000000568, -2.464576988612312114 ) ) ;
#60424=AXIS2_PLACEMENT_3D ( 'NONE', #88601, #38412, #23749 ) ;
#60431=CIRCLE ( 'NONE', #33240, 2.999999999999997780 ) ;
#60451=CARTESIAN_POINT ( 'NONE',  ( 208.6208076322478746, 32.98517505407394168, 10.00000000000000000 ) ) ;
#60454=CARTESIAN_POINT ( 'NONE',  ( 200.3186454232214828, 249.5000000000000568, -3.421094783296257713 ) ) ;
#60477=ORIENTED_EDGE ( 'NONE', *, *, #46440, .F. ) ;
#60480=LINE ( 'NONE', #43913, #2121 ) ;
#60490=DIRECTION ( 'NONE',  ( 0.6056179655966478226, -0.7957555401921982963, -0.000000000000000000 ) ) ;
#60500=CARTESIAN_POINT ( 'NONE',  ( 196.0143093133015384, 73.40565171261609123, 11.99999999999998757 ) ) ;
#60506=EDGE_LOOP ( 'NONE', ( #8650, #19852, #86083, #58627 ) ) ;
#60522=LINE ( 'NONE', #89358, #74773 ) ;
#60523=DIRECTION ( 'NONE',  ( -0.000000000000000000, -1.000000000000000000, -0.000000000000000000 ) ) ;
#60531=CARTESIAN_POINT ( 'NONE',  ( 207.7761861081325776, 35.69891260691533574, 14.41714557868295188 ) ) ;
#60535=EDGE_LOOP ( 'NONE', ( #81816, #28271, #34642 ) ) ;
#60536=CARTESIAN_POINT ( 'NONE',  ( 199.3270723581584321, 16.88338937786638994, -10.34008960743408245 ) ) ;
#60550=CYLINDRICAL_SURFACE ( 'NONE', #79111, 5.568361562975243650 ) ;
#60551=EDGE_CURVE ( 'NONE', #57747, #69256, #32093, .T. ) ;
#60552=CARTESIAN_POINT ( 'NONE',  ( 155.0589890788380387, 20.95955078618535694, -14.77888609070628334 ) ) ;
#60565=DIRECTION ( 'NONE',  ( 0.9693563597868444237, 0.2456588035076248955, 1.780678744869133453E-16 ) ) ;
#60567=CIRCLE ( 'NONE', #1537, 4.000000000000003553 ) ;
#60568=ADVANCED_FACE ( 'NONE', ( #42503 ), #92696, .T. ) ;
#60569=CARTESIAN_POINT ( 'NONE',  ( 152.4536156746142410, 250.5000000000000568, 12.49999999999999289 ) ) ;
#60574=AXIS2_PLACEMENT_3D ( 'NONE', #69882, #92573, #13537 ) ;
#60580=CARTESIAN_POINT ( 'NONE',  ( 180.7287904564219332, 275.5000000000000568, -24.90000000000003411 ) ) ;
#60590=ORIENTED_EDGE ( 'NONE', *, *, #76146, .T. ) ;
#60591=CARTESIAN_POINT ( 'NONE',  ( 200.2349812190172713, 66.43136063442170780, -7.741079165001072404 ) ) ;
#60602=VERTEX_POINT ( 'NONE', #26912 ) ;
#60605=DIRECTION ( 'NONE',  ( 0.000000000000000000, 1.000000000000000000, 0.000000000000000000 ) ) ;
#60607=LINE ( 'NONE', #30316, #28535 ) ;
#60610=DIRECTION ( 'NONE',  ( 0.000000000000000000, -0.7071067811865364705, -0.7071067811865584529 ) ) ;
#60611=CARTESIAN_POINT ( 'NONE',  ( 195.5045040238821059, 26.76854409577648397, 14.93905022940502469 ) ) ;
#60630=AXIS2_PLACEMENT_3D ( 'NONE', #89550, #12257, #62951 ) ;
#60635=CARTESIAN_POINT ( 'NONE',  ( 200.3691939013025092, 25.16710152838963666, 9.000000000000000000 ) ) ;
#60646=ORIENTED_EDGE ( 'NONE', *, *, #88318, .F. ) ;
#60647=DIRECTION ( 'NONE',  ( 0.000000000000000000, 1.000000000000000000, 0.000000000000000000 ) ) ;
#60657=FACE_OUTER_BOUND ( 'NONE', #83184, .T. ) ;
#60668=DIRECTION ( 'NONE',  ( 1.000000000000000000, 0.000000000000000000, 0.000000000000000000 ) ) ;
#60670=CARTESIAN_POINT ( 'NONE',  ( 196.9534188175200029, 25.84350552936208700, 12.42857142857142350 ) ) ;
#60682=CARTESIAN_POINT ( 'NONE',  ( 197.4288403404172243, 41.88980437486004149, 11.72798125285449267 ) ) ;
#60692=ORIENTED_EDGE ( 'NONE', *, *, #71569, .F. ) ;
#60695=CIRCLE ( 'NONE', #19863, 5.568361562975243650 ) ;
#60697=FACE_OUTER_BOUND ( 'NONE', #57032, .T. ) ;
#60708=CARTESIAN_POINT ( 'NONE',  ( 156.4851178187871312, 20.00000000000000000, -15.00000000000000000 ) ) ;
#60709=CARTESIAN_POINT ( 'NONE',  ( 194.2870706637141325, 39.36132622696000993, 14.58823529411763431 ) ) ;
#60711=CARTESIAN_POINT ( 'NONE',  ( 202.9738562182569694, 293.9636489450776367, -44.00000000000000000 ) ) ;
#60726=ORIENTED_EDGE ( 'NONE', *, *, #48544, .F. ) ;
#60728=ORIENTED_EDGE ( 'NONE', *, *, #3596, .T. ) ;
#60748=VERTEX_POINT ( 'NONE', #21206 ) ;
#60755=VERTEX_POINT ( 'NONE', #88386 ) ;
#60756=CARTESIAN_POINT ( 'NONE',  ( 140.6539576904058606, 250.0000000000000568, 12.00000000000000178 ) ) ;
#60769=VECTOR ( 'NONE', #80569, 1000.000000000000000 ) ;
#60776=AXIS2_PLACEMENT_3D ( 'NONE', #12221, #46783, #57203 ) ;
#60779=DIRECTION ( 'NONE',  ( 0.000000000000000000, 0.000000000000000000, -1.000000000000000000 ) ) ;
#60783=EDGE_CURVE ( 'NONE', #26361, #14181, #74581, .T. ) ;
#60787=CARTESIAN_POINT ( 'NONE',  ( 160.5350683151633291, 275.5000000000000568, 20.22542485937379908 ) ) ;
#60790=FACE_OUTER_BOUND ( 'NONE', #28052, .T. ) ;
#60792=CARTESIAN_POINT ( 'NONE',  ( 156.4972887742121372, 15.41695093167107444, -9.987829044571977732 ) ) ;
#60809=CARTESIAN_POINT ( 'NONE',  ( 139.6539576904058606, 275.0000000000000568, -10.49999999999999822 ) ) ;
#60812=DIRECTION ( 'NONE',  ( 0.000000000000000000, 1.000000000000000000, 0.000000000000000000 ) ) ;
#60830=VECTOR ( 'NONE', #51318, 1000.000000000000000 ) ;
#60832=AXIS2_PLACEMENT_3D ( 'NONE', #91760, #28326, #6076 ) ;
#60837=VECTOR ( 'NONE', #32943, 1000.000000000000000 ) ;
#60842=TOROIDAL_SURFACE ( 'NONE', #33581, 1.000000000000000000, 0.5000000000000000000 ) ;
#60850=EDGE_CURVE ( 'NONE', #25416, #4814, #23390, .T. ) ;
#60863=ORIENTED_EDGE ( 'NONE', *, *, #53345, .F. ) ;
#60868=ORIENTED_EDGE ( 'NONE', *, *, #69913, .T. ) ;
#60874=DIRECTION ( 'NONE',  ( 0.000000000000000000, 1.000000000000000000, 0.000000000000000000 ) ) ;
#60888=AXIS2_PLACEMENT_3D ( 'NONE', #85466, #20613, #85917 ) ;
#60895=AXIS2_PLACEMENT_3D ( 'NONE', #60072, #66695, #81812 ) ;
#60896=CARTESIAN_POINT ( 'NONE',  ( 198.0308761633362451, 68.10075688722794496, 9.048087686121785822 ) ) ;
#60898=AXIS2_PLACEMENT_3D ( 'NONE', #26558, #18992, #84298 ) ;
#60900=ADVANCED_FACE ( 'NONE', ( #28785 ), #65257, .F. ) ;
#60906=DIRECTION ( 'NONE',  ( 0.000000000000000000, 0.000000000000000000, -1.000000000000000000 ) ) ;
#60907=CARTESIAN_POINT ( 'NONE',  ( 197.1656530321902494, 41.90019538913895758, 12.64285714285713702 ) ) ;
#60913=CARTESIAN_POINT ( 'NONE',  ( 204.6539576904058606, 293.9636489450775230, 0.000000000000000000 ) ) ;
#60924=CARTESIAN_POINT ( 'NONE',  ( 193.9723528053802397, 215.0000000000000568, 17.29054515234648548 ) ) ;
#60939=VERTEX_POINT ( 'NONE', #58144 ) ;
#60942=CARTESIAN_POINT ( 'NONE',  ( 202.6701092853567445, 300.2474117005756966, -4.951178257753966250 ) ) ;
#60952=ORIENTED_EDGE ( 'NONE', *, *, #10009, .T. ) ;
#60953=CARTESIAN_POINT ( 'NONE',  ( 159.4851178187871312, 0.000000000000000000, -9.000000000000001776 ) ) ;
#60955=CIRCLE ( 'NONE', #79141, 4.000000000000003553 ) ;
#60962=CIRCLE ( 'NONE', #20131, 5.000000000000000888 ) ;
#60965=AXIS2_PLACEMENT_3D ( 'NONE', #54919, #89965, #25119 ) ;
#60966=DIRECTION ( 'NONE',  ( -1.000000000000000000, 0.000000000000000000, 0.000000000000000000 ) ) ;
#60970=EDGE_LOOP ( 'NONE', ( #56228, #86687, #92606, #71130 ) ) ;
#60971=ADVANCED_FACE ( 'NONE', ( #1290 ), #839, .F. ) ;
#60972=CIRCLE ( 'NONE', #83441, 0.5000000000000004441 ) ;
#60977=EDGE_CURVE ( 'NONE', #70200, #55010, #4924, .T. ) ;
#60980=AXIS2_PLACEMENT_3D ( 'NONE', #51916, #58587, #31097 ) ;
#60983=ORIENTED_EDGE ( 'NONE', *, *, #5338, .F. ) ;
#60993=EDGE_CURVE ( 'NONE', #61449, #15987, #21551, .T. ) ;
#60994=DIRECTION ( 'NONE',  ( 0.000000000000000000, 0.000000000000000000, 1.000000000000000000 ) ) ;
#61003=CARTESIAN_POINT ( 'NONE',  ( 194.2870706637141325, 39.36132622696000993, 14.58823529411763431 ) ) ;
#61005=TOROIDAL_SURFACE ( 'NONE', #9606, 25.50000000000000355, 0.5000000000000000000 ) ;
#61006=ORIENTED_EDGE ( 'NONE', *, *, #84888, .F. ) ;
#61021=CARTESIAN_POINT ( 'NONE',  ( 201.2104617360081704, 250.0000000000000568, -15.00000000000000000 ) ) ;
#61022=CARTESIAN_POINT ( 'NONE',  ( 165.2494399300530290, 8.542400036368780647, 9.974999999999996092 ) ) ;
#61030=DIRECTION ( 'NONE',  ( 0.000000000000000000, 0.000000000000000000, 1.000000000000000000 ) ) ;
#61035=CARTESIAN_POINT ( 'NONE',  ( 196.3496553477289979, 249.5000000000000568, -12.41762739670151205 ) ) ;
#61041=CIRCLE ( 'NONE', #85221, 27.00000000000000355 ) ;
#61047=AXIS2_PLACEMENT_3D ( 'NONE', #84991, #13525, #13989 ) ;
#61050=LINE ( 'NONE', #82338, #20427 ) ;
#61056=AXIS2_PLACEMENT_3D ( 'NONE', #50294, #92920, #1047 ) ;
#61061=EDGE_LOOP ( 'NONE', ( #46525, #32345, #25335, #8786, #80659, #69082, #34047 ) ) ;
#61062=FACE_OUTER_BOUND ( 'NONE', #46389, .T. ) ;
#61063=VECTOR ( 'NONE', #55314, 1000.000000000000114 ) ;
#61080=CARTESIAN_POINT ( 'NONE',  ( 197.9816010460261282, 65.99294033139044302, 9.931187365468728601 ) ) ;
#61085=LINE ( 'NONE', #90835, #87235 ) ;
#61086=CARTESIAN_POINT ( 'NONE',  ( 195.2312239546292574, 27.48493576247233250, 15.00000000000007638 ) ) ;
#61091=EDGE_CURVE ( 'NONE', #85305, #68325, #38660, .T. ) ;
#61096=ORIENTED_EDGE ( 'NONE', *, *, #73934, .F. ) ;
#61105=ORIENTED_EDGE ( 'NONE', *, *, #5615, .F. ) ;
#61108=DIRECTION ( 'NONE',  ( 0.000000000000000000, 1.000000000000000000, 0.000000000000000000 ) ) ;
#61130=AXIS2_PLACEMENT_3D ( 'NONE', #28711, #63321, #50002 ) ;
#61136=CARTESIAN_POINT ( 'NONE',  ( 199.7873597692581029, 25.48215708847424565, 10.49999999999999822 ) ) ;
#61137=VECTOR ( 'NONE', #29912, 1000.000000000000000 ) ;
#61143=VECTOR ( 'NONE', #15760, 1000.000000000000000 ) ;
#61159=CARTESIAN_POINT ( 'NONE',  ( 204.4184720700929745, 287.8409256575666859, -5.149838471383963778 ) ) ;
#61161=DIRECTION ( 'NONE',  ( -0.1455045995357750477, -0.000000000000000000, -0.9893575751536620722 ) ) ;
#61175=DIRECTION ( 'NONE',  ( 0.000000000000000000, 0.000000000000000000, -1.000000000000000000 ) ) ;
#61186=AXIS2_PLACEMENT_3D ( 'NONE', #5782, #20917, #55970 ) ;
#61187=CARTESIAN_POINT ( 'NONE',  ( 156.3365481965859374, 16.61859728808323666, 10.14856962220773617 ) ) ;
#61191=DIRECTION ( 'NONE',  ( -1.000000000000000000, 0.000000000000000000, 0.000000000000000000 ) ) ;
#61198=ADVANCED_FACE ( 'NONE', ( #83137 ), #83508, .T. ) ;
#61215=CARTESIAN_POINT ( 'NONE',  ( 196.8803347170859865, 20.19615242270662847, -12.49999999999999289 ) ) ;
#61227=CARTESIAN_POINT ( 'NONE',  ( 160.5350683151633291, 249.5000000000000568, 20.22542485937379908 ) ) ;
#61239=ORIENTED_EDGE ( 'NONE', *, *, #8590, .F. ) ;
#61244=ORIENTED_EDGE ( 'NONE', *, *, #56056, .F. ) ;
#61256=ADVANCED_FACE ( 'NONE', ( #82681 ), #44181, .T. ) ;
#61261=CYLINDRICAL_SURFACE ( 'NONE', #65721, 4.999999999999990230 ) ;
#61263=AXIS2_PLACEMENT_3D ( 'NONE', #89893, #81858, #17007 ) ;
#61267=CARTESIAN_POINT ( 'NONE',  ( 211.1232656141943949, 1.000000000000000888, 7.000000000000000000 ) ) ;
#61268=LINE ( 'NONE', #61716, #495 ) ;
#61273=ORIENTED_EDGE ( 'NONE', *, *, #32523, .F. ) ;
#61274=CARTESIAN_POINT ( 'NONE',  ( 208.1426553406905953, 36.40695478883779401, 14.84194439653754394 ) ) ;
#61276=AXIS2_PLACEMENT_3D ( 'NONE', #79954, #87499, #22648 ) ;
#61280=CARTESIAN_POINT ( 'NONE',  ( 154.8793480878648268, 20.01712742761865371, -11.60576973086971542 ) ) ;
#61295=EDGE_LOOP ( 'NONE', ( #47913, #4968, #82348, #88786 ) ) ;
#61297=CARTESIAN_POINT ( 'NONE',  ( 208.6208076322478746, 32.98517505407394168, 12.09245862095555601 ) ) ;
#61331=ADVANCED_FACE ( 'NONE', ( #82219 ), #23991, .F. ) ;
#61347=ORIENTED_EDGE ( 'NONE', *, *, #40483, .T. ) ;
#61348=VECTOR ( 'NONE', #63807, 1000.000000000000000 ) ;
#61353=ORIENTED_EDGE ( 'NONE', *, *, #77868, .T. ) ;
#61359=CARTESIAN_POINT ( 'NONE',  ( 151.6573119020006288, 20.00000000000000000, -4.897109440893268939 ) ) ;
#61373=FACE_OUTER_BOUND ( 'NONE', #65387, .T. ) ;
#61407=CIRCLE ( 'NONE', #29499, 4.000000000000003553 ) ;
#61417=ADVANCED_FACE ( 'NONE', ( #3622 ), #90238, .T. ) ;
#61420=ORIENTED_EDGE ( 'NONE', *, *, #58419, .F. ) ;
#61423=CYLINDRICAL_SURFACE ( 'NONE', #73166, 0.5000000000000004441 ) ;
#61435=DIRECTION ( 'NONE',  ( -0.000000000000000000, -1.000000000000000000, -0.000000000000000000 ) ) ;
#61445=CYLINDRICAL_SURFACE ( 'NONE', #5155, 7.910944475430059519 ) ;
#61449=VERTEX_POINT ( 'NONE', #54727 ) ;
#61463=CARTESIAN_POINT ( 'NONE',  ( 0.000000000000000000, 0.000000000000000000, -9.000000000000001776 ) ) ;
#61465=EDGE_CURVE ( 'NONE', #13609, #135, #66904, .T. ) ;
#61467=CARTESIAN_POINT ( 'NONE',  ( 153.1745786719506270, 129.2309077672098283, 12.62609896151546351 ) ) ;
#61468=CARTESIAN_POINT ( 'NONE',  ( 175.2296996224750103, 275.5000000000000568, 24.50000000000000355 ) ) ;
#61478=CARTESIAN_POINT ( 'NONE',  ( 196.8803347170859865, 20.19615242270663558, 12.49999999999999289 ) ) ;
#61491=LINE ( 'NONE', #90778, #88197 ) ;
#61492=CARTESIAN_POINT ( 'NONE',  ( 153.6987871352711181, 19.48326534539917887, -11.45812909362560639 ) ) ;
#61506=FACE_OUTER_BOUND ( 'NONE', #1557, .T. ) ;
#61512=CYLINDRICAL_SURFACE ( 'NONE', #6422, 0.5000000000000004441 ) ;
#61515=CARTESIAN_POINT ( 'NONE',  ( 175.2296996224750103, 247.0000000000001137, 0.000000000000000000 ) ) ;
#61525=DIRECTION ( 'NONE',  ( 0.7957555401921980742, 0.6056179655966482667, 0.000000000000000000 ) ) ;
#61527=CARTESIAN_POINT ( 'NONE',  ( 208.2002815004974252, 0.04196010845019423202, -7.500000000000014211 ) ) ;
#61536=ORIENTED_EDGE ( 'NONE', *, *, #899, .T. ) ;
#61540=CARTESIAN_POINT ( 'NONE',  ( 198.9506515269325178, 68.58287003106127599, -4.213754548338595640 ) ) ;
#61542=CARTESIAN_POINT ( 'NONE',  ( 156.8041522122653930, 275.5000000000000568, 16.89672165344857646 ) ) ;
#61546=CARTESIAN_POINT ( 'NONE',  ( 208.0393982316568326, 37.47427918878999265, 12.00000000000000000 ) ) ;
#61547=CARTESIAN_POINT ( 'NONE',  ( 195.2258176893294035, 27.09966188323243586, 15.00706248549522925 ) ) ;
#61560=EDGE_CURVE ( 'NONE', #90042, #63082, #16487, .T. ) ;
#61563=ORIENTED_EDGE ( 'NONE', *, *, #90310, .T. ) ;
#61564=DIRECTION ( 'NONE',  ( -0.000000000000000000, -1.000000000000000000, -0.000000000000000000 ) ) ;
#61581=CARTESIAN_POINT ( 'NONE',  ( 140.6539576904058606, 250.5000000000000568, 12.50000000000000000 ) ) ;
#61602=CARTESIAN_POINT ( 'NONE',  ( 164.7123623445222904, 3.000000000000000000, -9.000000000000001776 ) ) ;
#61608=EDGE_CURVE ( 'NONE', #79037, #90280, #44885, .T. ) ;
#61616=DIRECTION ( 'NONE',  ( -0.9893575751536621832, 0.000000000000000000, 0.1455045995357737432 ) ) ;
#61630=DIRECTION ( 'NONE',  ( -2.312964634635742267E-15, 0.000000000000000000, 1.000000000000000000 ) ) ;
#61641=FACE_OUTER_BOUND ( 'NONE', #23810, .T. ) ;
#61656=ORIENTED_EDGE ( 'NONE', *, *, #74648, .T. ) ;
#61658=ORIENTED_EDGE ( 'NONE', *, *, #39601, .F. ) ;
#61687=ORIENTED_EDGE ( 'NONE', *, *, #53825, .T. ) ;
#61688=DIRECTION ( 'NONE',  ( 0.000000000000000000, 0.000000000000000000, 1.000000000000000000 ) ) ;
#61692=ORIENTED_EDGE ( 'NONE', *, *, #53477, .F. ) ;
#61699=DIRECTION ( 'NONE',  ( -0.000000000000000000, -0.000000000000000000, -1.000000000000000000 ) ) ;
#61704=CARTESIAN_POINT ( 'NONE',  ( 209.3190042249899250, 30.23012903947020646, 14.26380412667039188 ) ) ;
#61715=DIRECTION ( 'NONE',  ( -0.000000000000000000, -1.000000000000000000, -0.000000000000000000 ) ) ;
#61716=CARTESIAN_POINT ( 'NONE',  ( 185.2169494693457921, 250.0000000000000568, 22.91843887563416615 ) ) ;
#61718=B_SPLINE_CURVE_WITH_KNOTS ( 'NONE', 3,
 ( #19208, #70361, #32489, #47606, #5486, #20145, #62303, #25828, #91143, #68942, #48067, #27251, #49028, #19669 ),
 .UNSPECIFIED., .F., .F.,
 ( 4, 2, 2, 2, 2, 2, 4 ),
 ( 0.000000000000000000, 0.001076125775146711833, 0.001614188662720042597, 0.002152251550293373793, 0.003228377325440022309, 0.003766440213013335508, 0.004304503100586647840 ),
 .UNSPECIFIED. ) ;
#61720=EDGE_CURVE ( 'NONE', #51424, #24735, #26062, .T. ) ;
#61721=DIRECTION ( 'NONE',  ( 0.000000000000000000, 1.000000000000000000, 0.000000000000000000 ) ) ;
#61723=CARTESIAN_POINT ( 'NONE',  ( 159.3464669004252130, 15.95758591462619336, -10.08665682397418983 ) ) ;
#61725=CYLINDRICAL_SURFACE ( 'NONE', #55834, 0.5000000000000004441 ) ;
#61740=CARTESIAN_POINT ( 'NONE',  ( 159.4851178187871312, 3.000000000000000000, -9.000000000000001776 ) ) ;
#61744=CARTESIAN_POINT ( 'NONE',  ( 197.0969223827550536, 71.90335919811118970, 12.15580473211910473 ) ) ;
#61772=EDGE_LOOP ( 'NONE', ( #33697, #90633, #74592, #35441 ) ) ;
#61775=VERTEX_POINT ( 'NONE', #37326 ) ;
#61781=CIRCLE ( 'NONE', #45121, 0.5000000000000017764 ) ;
#61792=ORIENTED_EDGE ( 'NONE', *, *, #24971, .F. ) ;
#61798=ORIENTED_EDGE ( 'NONE', *, *, #93067, .T. ) ;
#61801=ORIENTED_EDGE ( 'NONE', *, *, #4649, .F. ) ;
#61808=FACE_OUTER_BOUND ( 'NONE', #21842, .T. ) ;
#61812=CARTESIAN_POINT ( 'NONE',  ( 206.7809450508160865, 35.77530089738195329, 14.49999999999999822 ) ) ;
#61817=B_SPLINE_CURVE_WITH_KNOTS ( 'NONE', 3,
 ( #90544, #54124, #17690, #54584, #20379, #5702, #47475, #82539 ),
 .UNSPECIFIED., .F., .F.,
 ( 4, 2, 2, 4 ),
 ( 2.841933599792538093E-17, 0.001370196721548293728, 0.002055295082322467371, 0.002740393443096640798 ),
 .UNSPECIFIED. ) ;
#61822=CARTESIAN_POINT ( 'NONE',  ( 153.6947954963213760, 20.34868745056155959, -12.70025883435339864 ) ) ;
#61832=DIRECTION ( 'NONE',  ( -0.7071067811864494290, 8.659560562353731078E-17, 0.7071067811866457165 ) ) ;
#61840=EDGE_CURVE ( 'NONE', #64275, #26750, #89143, .T. ) ;
#61845=AXIS2_PLACEMENT_3D ( 'NONE', #42727, #36564, #51228 ) ;
#61869=CARTESIAN_POINT ( 'NONE',  ( 198.5843229385366726, 69.20886829666338258, 9.718619512930896320 ) ) ;
#61871=CARTESIAN_POINT ( 'NONE',  ( 164.2231345125756263, 300.2961574867697436, -7.500000000000000000 ) ) ;
#61882=VERTEX_POINT ( 'NONE', #52925 ) ;
#61893=CARTESIAN_POINT ( 'NONE',  ( 154.3984422716669940, 19.39780977728399591, -12.47739260116905236 ) ) ;
#61897=ORIENTED_EDGE ( 'NONE', *, *, #36317, .T. ) ;
#61906=ORIENTED_EDGE ( 'NONE', *, *, #12664, .F. ) ;
#61912=CARTESIAN_POINT ( 'NONE',  ( 180.2288731078812702, 214.9910457053126720, -24.90909090909092782 ) ) ;
#61913=VECTOR ( 'NONE', #81959, 1000.000000000000000 ) ;
#61921=CARTESIAN_POINT ( 'NONE',  ( 198.6884013828325521, 64.61450673763174279, 9.555809373750800972 ) ) ;
#61925=EDGE_LOOP ( 'NONE', ( #91244, #84808, #6681, #61239 ) ) ;
#61926=CARTESIAN_POINT ( 'NONE',  ( 198.6639115758706282, 17.12212513345059151, 10.45170682515551164 ) ) ;
#61942=CYLINDRICAL_SURFACE ( 'NONE', #3492, 4.103083949679980691 ) ;
#61956=DIRECTION ( 'NONE',  ( 0.9693563597868444237, 0.2456588035076248677, -0.000000000000000000 ) ) ;
#61958=FACE_OUTER_BOUND ( 'NONE', #47748, .T. ) ;
#61966=DIRECTION ( 'NONE',  ( 0.000000000000000000, -1.000000000000000000, 0.000000000000000000 ) ) ;
#61972=ADVANCED_FACE ( 'NONE', ( #38718 ), #36102, .T. ) ;
#61973=VECTOR ( 'NONE', #71547, 1000.000000000000000 ) ;
#61976=ORIENTED_EDGE ( 'NONE', *, *, #6158, .F. ) ;
#61978=DIRECTION ( 'NONE',  ( -0.000000000000000000, -1.000000000000000000, -0.000000000000000000 ) ) ;
#61979=AXIS2_PLACEMENT_3D ( 'NONE', #37587, #9645, #30982 ) ;
#61993=FACE_OUTER_BOUND ( 'NONE', #75072, .T. ) ;
#62000=DIRECTION ( 'NONE',  ( 0.000000000000000000, 1.000000000000000000, 0.000000000000000000 ) ) ;
#62001=CARTESIAN_POINT ( 'NONE',  ( 195.7694206965761623, 25.16799831920000940, 14.25285053635913535 ) ) ;
#62020=ORIENTED_EDGE ( 'NONE', *, *, #77692, .T. ) ;
#62021=B_SPLINE_CURVE_WITH_KNOTS ( 'NONE', 3,
 ( #22201, #66233, #15096, #30231, #59121, #79512, #86577, #23116 ),
 .UNSPECIFIED., .F., .F.,
 ( 4, 2, 2, 4 ),
 ( 0.000000000000000000, 0.0002353609534302958644, 0.0004707219068605917288, 0.0009414438137211129844 ),
 .UNSPECIFIED. ) ;
#62022=DIRECTION ( 'NONE',  ( -0.000000000000000000, 1.000000000000000000, -0.000000000000000000 ) ) ;
#62027=CARTESIAN_POINT ( 'NONE',  ( 152.9190334681021000, 20.54289017631687386, -11.30277777986246690 ) ) ;
#62038=CARTESIAN_POINT ( 'NONE',  ( 159.4851178187871312, 17.02694846567680642, -9.999999999999998224 ) ) ;
#62043=AXIS2_PLACEMENT_3D ( 'NONE', #82803, #76184, #9911 ) ;
#62059=CARTESIAN_POINT ( 'NONE',  ( 197.1844320129423807, 70.43964897667966341, 15.08154681515735440 ) ) ;
#62069=CARTESIAN_POINT ( 'NONE',  ( 153.9755810662746569, 128.3195885613610869, -13.16651113973756715 ) ) ;
#62071=CARTESIAN_POINT ( 'NONE',  ( 199.9020372526622680, 288.4596041913513886, -5.812224296395849699 ) ) ;
#62073=EDGE_CURVE ( 'NONE', #23700, #88648, #27648, .T. ) ;
#62086=VERTEX_POINT ( 'NONE', #4609 ) ;
#62087=DIRECTION ( 'NONE',  ( -0.000000000000000000, -1.000000000000000000, -0.000000000000000000 ) ) ;
#62090=DIRECTION ( 'NONE',  ( 0.000000000000000000, 0.000000000000000000, 1.000000000000000000 ) ) ;
#62095=( BOUNDED_CURVE ( )  B_SPLINE_CURVE ( 3, ( #75752, #26020, #26504, #69588 ),
 .UNSPECIFIED., .F., .F. ) 
 B_SPLINE_CURVE_WITH_KNOTS ( ( 4, 4 ),
 ( 5.759586531581287971, 6.283185307179586232 ),
 .UNSPECIFIED. ) 
 CURVE ( )  GEOMETRIC_REPRESENTATION_ITEM ( )  RATIONAL_B_SPLINE_CURVE ( ( 1.000000000000000000, 0.9772838841927120601, 0.9772838841927120601, 1.000000000000000000 ) ) 
 REPRESENTATION_ITEM ( '' )  );
#62102=( BOUNDED_CURVE ( )  B_SPLINE_CURVE ( 3, ( #38872, #73942, #8151, #1979 ),
 .UNSPECIFIED., .F., .T. ) 
 B_SPLINE_CURVE_WITH_KNOTS ( ( 4, 4 ),
 ( 3.141592653589793116, 4.712388980384689674 ),
 .UNSPECIFIED. ) 
 CURVE ( )  GEOMETRIC_REPRESENTATION_ITEM ( )  RATIONAL_B_SPLINE_CURVE ( ( 1.000000000000000000, 0.8047378541243649375, 0.8047378541243649375, 1.000000000000000000 ) ) 
 REPRESENTATION_ITEM ( '' )  );
#62106=AXIS2_PLACEMENT_3D ( 'NONE', #83989, #41349, #91551 ) ;
#62110=AXIS2_PLACEMENT_3D ( 'NONE', #16315, #52746, #31004 ) ;
#62121=ORIENTED_EDGE ( 'NONE', *, *, #4934, .F. ) ;
#62123=ORIENTED_EDGE ( 'NONE', *, *, #35848, .F. ) ;
#62140=CARTESIAN_POINT ( 'NONE',  ( 211.1232656141943949, 1.000000000000000000, -7.000000000000000888 ) ) ;
#62155=CARTESIAN_POINT ( 'NONE',  ( 221.8344101925596306, 35.72494958537217968, 10.00000000000000000 ) ) ;
#62159=ORIENTED_EDGE ( 'NONE', *, *, #10818, .T. ) ;
#62166=FACE_OUTER_BOUND ( 'NONE', #60506, .T. ) ;
#62181=FACE_OUTER_BOUND ( 'NONE', #53484, .T. ) ;
#62182=DIRECTION ( 'NONE',  ( 0.000000000000000000, -1.000000000000000000, 0.000000000000000000 ) ) ;
#62184=AXIS2_PLACEMENT_3D ( 'NONE', #1087, #80153, #71682 ) ;
#62186=VECTOR ( 'NONE', #28133, 1000.000000000000000 ) ;
#62187=CARTESIAN_POINT ( 'NONE',  ( 156.5058941793770657, 215.0000000000001705, 17.26454883540702312 ) ) ;
#62190=DIRECTION ( 'NONE',  ( -0.000000000000000000, -0.000000000000000000, -1.000000000000000000 ) ) ;
#62204=ORIENTED_EDGE ( 'NONE', *, *, #79269, .T. ) ;
#62207=DIRECTION ( 'NONE',  ( 0.000000000000000000, 0.000000000000000000, 1.000000000000000000 ) ) ;
#62209=ORIENTED_EDGE ( 'NONE', *, *, #39485, .T. ) ;
#62216=EDGE_CURVE ( 'NONE', #44839, #64177, #62454, .T. ) ;
#62243=ORIENTED_EDGE ( 'NONE', *, *, #6158, .T. ) ;
#62261=ORIENTED_EDGE ( 'NONE', *, *, #71290, .T. ) ;
#62268=ORIENTED_EDGE ( 'NONE', *, *, #64378, .F. ) ;
#62270=ORIENTED_EDGE ( 'NONE', *, *, #70753, .F. ) ;
#62277=CARTESIAN_POINT ( 'NONE',  ( 151.7270317713903296, 20.05858947365025102, -8.551724154019398227 ) ) ;
#62282=CARTESIAN_POINT ( 'NONE',  ( 197.0537578383379582, 24.40161896276961073, 12.19962234278438906 ) ) ;
#62295=CARTESIAN_POINT ( 'NONE',  ( 199.6702811234769683, 65.52214591209386185, 9.100946541886340668 ) ) ;
#62300=CARTESIAN_POINT ( 'NONE',  ( 195.4781563537916043, 39.36132622696000283, 14.00000000000000000 ) ) ;
#62303=CARTESIAN_POINT ( 'NONE',  ( 196.0790001906461271, 41.35036787528040492, 14.17104486492339888 ) ) ;
#62304=CARTESIAN_POINT ( 'NONE',  ( 199.4392256788250677, 65.82574266882504332, 7.741079165001067963 ) ) ;
#62309=CARTESIAN_POINT ( 'NONE',  ( 140.6539576904058606, 275.0000000000000568, -11.50000000000000000 ) ) ;
#62324=DIRECTION ( 'NONE',  ( 0.000000000000000000, 0.000000000000000000, 1.000000000000000000 ) ) ;
#62342=CARTESIAN_POINT ( 'NONE',  ( 175.2296996224750103, 140.2072866198470251, -24.00000000000002132 ) ) ;
#62353=VERTEX_POINT ( 'NONE', #41979 ) ;
#62363=DIRECTION ( 'NONE',  ( 1.000000000000000000, -0.000000000000000000, 0.000000000000000000 ) ) ;
#62364=DIRECTION ( 'NONE',  ( 0.000000000000000000, 0.000000000000000000, -1.000000000000000000 ) ) ;
#62382=DIRECTION ( 'NONE',  ( -0.3024135303179443235, -0.9531768234071985590, -1.474514954580288870E-14 ) ) ;
#62384=EDGE_CURVE ( 'NONE', #1828, #17769, #21619, .T. ) ;
#62385=CARTESIAN_POINT ( 'NONE',  ( 221.5917695054403111, 1.242640687119284992, -10.00000000000000000 ) ) ;
#62386=AXIS2_PLACEMENT_3D ( 'NONE', #14444, #215, #42824 ) ;
#62397=CARTESIAN_POINT ( 'NONE',  ( 159.4851178187871312, 15.00000000000000000, 7.000000000000000000 ) ) ;
#62399=CARTESIAN_POINT ( 'NONE',  ( 175.2296996224750103, 250.5000000000000568, 0.000000000000000000 ) ) ;
#62400=CONICAL_SURFACE ( 'NONE', #27660, 24.00000000000001066, 0.7853981633974361776 ) ;
#62402=ORIENTED_EDGE ( 'NONE', *, *, #17632, .T. ) ;
#62418=DIRECTION ( 'NONE',  ( -0.4646852846009910110, 0.2294442726657860421, -0.8552326654286331875 ) ) ;
#62420=AXIS2_PLACEMENT_3D ( 'NONE', #84778, #4786, #62090 ) ;
#62431=CARTESIAN_POINT ( 'NONE',  ( 0.000000000000000000, 15.00000000000000000, 10.00000000000000000 ) ) ;
#62433=DIRECTION ( 'NONE',  ( 0.000000000000000000, 1.000000000000000000, -0.000000000000000000 ) ) ;
#62442=CARTESIAN_POINT ( 'NONE',  ( 196.8872833010042598, 42.02416330566288138, 12.48796469961283684 ) ) ;
#62450=VECTOR ( 'NONE', #3586, 1000.000000000000000 ) ;
#62452=EDGE_LOOP ( 'NONE', ( #17660, #43571, #75751, #4040 ) ) ;
#62454=CIRCLE ( 'NONE', #56378, 0.5000000000000004441 ) ;
#62473=CIRCLE ( 'NONE', #70035, 22.83127060016883192 ) ;
#62476=EDGE_CURVE ( 'NONE', #84950, #27314, #58519, .T. ) ;
#62480=LINE ( 'NONE', #47289, #48800 ) ;
#62481=VECTOR ( 'NONE', #53427, 1000.000000000000000 ) ;
#62482=CARTESIAN_POINT ( 'NONE',  ( 195.6954295768035479, 25.61923908820089224, 14.35989702634663345 ) ) ;
#62492=AXIS2_PLACEMENT_3D ( 'NONE', #56405, #35561, #87120 ) ;
#62493=ORIENTED_EDGE ( 'NONE', *, *, #13958, .F. ) ;
#62500=EDGE_CURVE ( 'NONE', #52231, #70265, #36686, .T. ) ;
#62503=ORIENTED_EDGE ( 'NONE', *, *, #25613, .F. ) ;
#62504=CARTESIAN_POINT ( 'NONE',  ( 175.2296996224750103, 149.6461846693799487, 0.000000000000000000 ) ) ;
#62519=ORIENTED_EDGE ( 'NONE', *, *, #61608, .T. ) ;
#62522=AXIS2_PLACEMENT_3D ( 'NONE', #93263, #71510, #28417 ) ;
#62528=CIRCLE ( 'NONE', #45864, 0.5000000000000004441 ) ;
#62530=DIRECTION ( 'NONE',  ( 0.000000000000000000, 0.000000000000000000, -1.000000000000000000 ) ) ;
#62531=AXIS2_PLACEMENT_3D ( 'NONE', #43176, #80081, #64986 ) ;
#62544=AXIS2_PLACEMENT_3D ( 'NONE', #59752, #81033, #30380 ) ;
#62546=CARTESIAN_POINT ( 'NONE',  ( 175.2296996224750103, 140.2072866198470251, 24.00000000000002132 ) ) ;
#62548=DIRECTION ( 'NONE',  ( 1.000000000000000000, 4.095251346825558428E-15, 0.000000000000000000 ) ) ;
#62557=CARTESIAN_POINT ( 'NONE',  ( 153.2628468892384603, 20.37991841447902175, -11.93555113919331134 ) ) ;
#62560=CARTESIAN_POINT ( 'NONE',  ( 204.1749232501770450, 287.7883336863533259, -5.086027127806754145 ) ) ;
#62562=CARTESIAN_POINT ( 'NONE',  ( 0.000000000000000000, 15.00000000000000000, 9.000000000000001776 ) ) ;
#62569=ADVANCED_FACE ( 'NONE', ( #63809 ), #20697, .F. ) ;
#62572=ORIENTED_EDGE ( 'NONE', *, *, #3543, .F. ) ;
#62589=CARTESIAN_POINT ( 'NONE',  ( 153.4180177809303416, 19.62189878706044865, -10.83803683443614396 ) ) ;
#62600=VECTOR ( 'NONE', #66728, 1000.000000000000000 ) ;
#62610=CIRCLE ( 'NONE', #30834, 4.999999999999990230 ) ;
#62620=EDGE_LOOP ( 'NONE', ( #13140, #74835, #7065, #1101, #56432, #13355 ) ) ;
#62633=ORIENTED_EDGE ( 'NONE', *, *, #78401, .T. ) ;
#62637=AXIS2_PLACEMENT_3D ( 'NONE', #42045, #78530, #14143 ) ;
#62643=DIRECTION ( 'NONE',  ( -0.000000000000000000, 1.000000000000000000, 0.000000000000000000 ) ) ;
#62646=EDGE_CURVE ( 'NONE', #20445, #69103, #42765, .T. ) ;
#62671=DIRECTION ( 'NONE',  ( 0.000000000000000000, 0.000000000000000000, -1.000000000000000000 ) ) ;
#62672=FACE_OUTER_BOUND ( 'NONE', #63806, .T. ) ;
#62674=AXIS2_PLACEMENT_3D ( 'NONE', #66941, #51323, #88700 ) ;
#62677=CARTESIAN_POINT ( 'NONE',  ( 209.8744251295252354, 28.03846817292548366, 10.50000000000000000 ) ) ;
#62680=CARTESIAN_POINT ( 'NONE',  ( 208.3418117619748102, 38.42745601219717599, 14.33494424848941406 ) ) ;
#62682=( BOUNDED_SURFACE ( )  B_SPLINE_SURFACE ( 3, 2, ( 
 ( #23013, #16847, #2652 ),
 ( #23496, #800, #16386 ),
 ( #74141, #44325, #52819 ),
 ( #51892, #29680, #22551 ),
 ( #52364, #15454, #2188 ),
 ( #79858, #87404, #51425 ) ),
 .UNSPECIFIED., .F., .F., .F. ) 
 B_SPLINE_SURFACE_WITH_KNOTS ( ( 4, 2, 4 ),
 ( 3, 3 ),
 ( 3.871320309816757010, 4.291854645100723786, 4.712388980384689674 ),
 ( 0.000000000000000000, 1.000000000000000000 ),
 .UNSPECIFIED. ) 
 GEOMETRIC_REPRESENTATION_ITEM ( )  RATIONAL_B_SPLINE_SURFACE ( (
 ( 1.000000000000000000, 0.7827533893364934103, 1.000000000000000000),
 ( 1.000000000000000000, 0.7737378266060769283, 1.000000000000000000),
 ( 1.000000000000000000, 0.7623946665110049592, 1.000000000000000000),
 ( 1.000000000000000000, 0.7365781863221951831, 1.000000000000000000),
 ( 1.000000000000000000, 0.7221049971011784807, 1.000000000000000000),
 ( 1.000000000000000000, 0.7071067811865479058, 1.000000000000000000) ) ) 
 REPRESENTATION_ITEM ( '' )  SURFACE ( )  );
#62683=DIRECTION ( 'NONE',  ( 0.8660254037844359321, 0.5000000000000046629, -0.000000000000000000 ) ) ;
#62686=CARTESIAN_POINT ( 'NONE',  ( 156.3051094419662945, 18.69637893469953838, -10.18000837680961723 ) ) ;
#62693=AXIS2_PLACEMENT_3D ( 'NONE', #29240, #20738, #28316 ) ;
#62694=( BOUNDED_SURFACE ( )  B_SPLINE_SURFACE ( 3, 2, ( 
 ( #4664, #18885, #62929 ),
 ( #78518, #91763, #76638 ),
 ( #92700, #77103, #83725 ),
 ( #48674, #26451, #70491 ),
 ( #27870, #70948, #84191 ),
 ( #6080, #11763, #34954 ),
 ( #63866, #12234, #26915 ),
 ( #47740, #56763, #78056 ),
 ( #41081, #55340, #40615 ),
 ( #13655, #70005, #6551 ),
 ( #55802, #13198, #77575 ),
 ( #42034, #35430, #33537 ),
 ( #69531, #20289, #56275 ),
 ( #5619, #19806, #34494 ),
 ( #90803, #84654, #19339 ),
 ( #85604, #62442, #20751 ) ),
 .UNSPECIFIED., .F., .F., .F. ) 
 B_SPLINE_SURFACE_WITH_KNOTS ( ( 4, 2, 2, 2, 2, 2, 2, 4 ),
 ( 3, 3 ),
 ( -6.938893903907228378E-18, 0.0006169105258908286335, 0.001233821051781664206, 0.001850731577672499670, 0.002467642103563335351, 0.003084552629454171031, 0.003701463155345006278, 0.004935284207126677640 ),
 ( 0.000000000000000000, 1.000000000000000000 ),
 .UNSPECIFIED. ) 
 GEOMETRIC_REPRESENTATION_ITEM ( )  RATIONAL_B_SPLINE_SURFACE ( (
 ( 1.000000000000000000, 0.8966167345234229424, 1.000000000000000000),
 ( 1.000000000000000000, 0.9004139148586555175, 1.000000000000000000),
 ( 1.000000000000000000, 0.9032061010818291935, 1.000000000000000000),
 ( 1.000000000000000000, 0.9067734849417629084, 1.000000000000000000),
 ( 1.000000000000000000, 0.9075308745986051528, 1.000000000000000000),
 ( 1.000000000000000000, 0.9069696504590781805, 1.000000000000000000),
 ( 1.000000000000000000, 0.9056888044683030214, 1.000000000000000000),
 ( 1.000000000000000000, 0.9012558131641384973, 1.000000000000000000),
 ( 1.000000000000000000, 0.8981641526222049476, 1.000000000000000000),
 ( 1.000000000000000000, 0.8905754533014459406, 1.000000000000000000),
 ( 1.000000000000000000, 0.8860218362703521366, 1.000000000000000000),
 ( 1.000000000000000000, 0.8759703649549664961, 1.000000000000000000),
 ( 1.000000000000000000, 0.8704567387598657335, 1.000000000000000000),
 ( 1.000000000000000000, 0.8526573370808110397, 1.000000000000000000),
 ( 1.000000000000000000, 0.8394012181876917555, 1.000000000000000000),
 ( 1.000000000000000000, 0.8255171224912107864, 1.000000000000000000) ) ) 
 REPRESENTATION_ITEM ( '' )  SURFACE ( )  );
#62695=AXIS2_PLACEMENT_3D ( 'NONE', #16141, #59716, #29427 ) ;
#62699=ORIENTED_EDGE ( 'NONE', *, *, #45671, .T. ) ;
#62702=DIRECTION ( 'NONE',  ( -0.000000000000000000, -1.000000000000000000, -0.000000000000000000 ) ) ;
#62706=CARTESIAN_POINT ( 'NONE',  ( 170.7304434856092143, 249.5000000000000568, -24.91818181818180733 ) ) ;
#62710=AXIS2_PLACEMENT_3D ( 'NONE', #3874, #48812, #12371 ) ;
#62739=ORIENTED_EDGE ( 'NONE', *, *, #25508, .F. ) ;
#62755=ORIENTED_EDGE ( 'NONE', *, *, #82892, .F. ) ;
#62761=ORIENTED_EDGE ( 'NONE', *, *, #51451, .F. ) ;
#62772=CARTESIAN_POINT ( 'NONE',  ( 197.2116943569230045, 249.5000000000000568, -11.92446933126075415 ) ) ;
#62777=CARTESIAN_POINT ( 'NONE',  ( 197.4836817735085219, 24.47698789593438917, 11.66666666666666785 ) ) ;
#62784=CARTESIAN_POINT ( 'NONE',  ( 154.7659666677267580, 19.56018909072084710, -12.94946946941271726 ) ) ;
#62789=CARTESIAN_POINT ( 'NONE',  ( 198.7884250876676049, 66.56295291868792674, 9.416620882813951710 ) ) ;
#62796=CARTESIAN_POINT ( 'NONE',  ( 164.2231345125756263, 300.2961574867697436, 7.500000000000000000 ) ) ;
#62801=CARTESIAN_POINT ( 'NONE',  ( 207.6275970751953537, 36.17632364500597220, 14.41714557868297852 ) ) ;
#62809=PLANE ( 'NONE',  #78748 ) ;
#62810=DIRECTION ( 'NONE',  ( 1.000000000000000000, -0.000000000000000000, 0.000000000000000000 ) ) ;
#62812=ADVANCED_FACE ( 'NONE', ( #42929 ), #74532, .T. ) ;
#62814=ADVANCED_FACE ( 'NONE', ( #62874 ), #20228, .T. ) ;
#62832=CARTESIAN_POINT ( 'NONE',  ( 204.1778867865513405, 300.1383591958309012, -5.086762277128879184 ) ) ;
#62842=AXIS2_PLACEMENT_3D ( 'NONE', #39718, #47771, #12272 ) ;
#62853=CARTESIAN_POINT ( 'NONE',  ( 197.9737958995921190, 68.21405198623872934, 9.113933396921945373 ) ) ;
#62858=ORIENTED_EDGE ( 'NONE', *, *, #83602, .T. ) ;
#62867=ORIENTED_EDGE ( 'NONE', *, *, #34695, .T. ) ;
#62871=ORIENTED_EDGE ( 'NONE', *, *, #75705, .F. ) ;
#62874=FACE_OUTER_BOUND ( 'NONE', #52783, .T. ) ;
#62881=CARTESIAN_POINT ( 'NONE',  ( 154.2407877675970269, 20.33090418404277955, 11.64082518123277943 ) ) ;
#62883=FACE_OUTER_BOUND ( 'NONE', #31414, .T. ) ;
#62886=CARTESIAN_POINT ( 'NONE',  ( 175.2296996224750103, 247.0000000000001137, -9.550761578869391144 ) ) ;
#62901=CARTESIAN_POINT ( 'NONE',  ( 197.2116943569230330, 250.5000000000000568, -12.92446933126074882 ) ) ;
#62916=DIRECTION ( 'NONE',  ( 0.000000000000000000, 0.000000000000000000, 1.000000000000000000 ) ) ;
#62917=ADVANCED_FACE ( 'NONE', ( #64292 ), #4033, .F. ) ;
#62926=CARTESIAN_POINT ( 'NONE',  ( 156.4851178187871312, 1.734723475976806897E-15, -8.757359312880714342 ) ) ;
#62929=CARTESIAN_POINT ( 'NONE',  ( 195.4781563537916043, 39.36132622696000283, 15.00000000000000000 ) ) ;
#62937=ORIENTED_EDGE ( 'NONE', *, *, #53136, .F. ) ;
#62938=DIRECTION ( 'NONE',  ( 0.000000000000000000, 0.000000000000000000, 1.000000000000000000 ) ) ;
#62950=ORIENTED_EDGE ( 'NONE', *, *, #49823, .T. ) ;
#62951=DIRECTION ( 'NONE',  ( 1.110223024625156343E-15, 0.000000000000000000, 1.000000000000000000 ) ) ;
#62954=CARTESIAN_POINT ( 'NONE',  ( 200.6103193995254230, 215.0000000000000568, -2.464576988612307229 ) ) ;
#62963=CARTESIAN_POINT ( 'NONE',  ( 200.4551663813218454, 64.49084098419280053, -2.617322427804798401 ) ) ;
#62986=VERTEX_POINT ( 'NONE', #52240 ) ;
#62987=CARTESIAN_POINT ( 'NONE',  ( 155.2898987420118431, 20.78850644404472092, -13.36622507082863187 ) ) ;
#63003=PLANE ( 'NONE',  #60965 ) ;
#63027=CARTESIAN_POINT ( 'NONE',  ( 140.6539576904058606, 130.0000000000000568, 12.50000000000000000 ) ) ;
#63038=DIRECTION ( 'NONE',  ( 0.000000000000000000, 0.000000000000000000, -1.000000000000000000 ) ) ;
#63047=EDGE_CURVE ( 'NONE', #56700, #30213, #35207, .T. ) ;
#63050=B_SPLINE_CURVE_WITH_KNOTS ( 'NONE', 3,
 ( #58811, #15247, #80563, #79200 ),
 .UNSPECIFIED., .F., .F.,
 ( 4, 4 ),
 ( 3.469446951953614189E-18, 9.632970524405874116E-05 ),
 .UNSPECIFIED. ) ;
#63051=VERTEX_POINT ( 'NONE', #60756 ) ;
#63054=CARTESIAN_POINT ( 'NONE',  ( 152.4536156746142410, 249.5000000000000568, 14.50000000000000000 ) ) ;
#63065=FACE_OUTER_BOUND ( 'NONE', #21635, .T. ) ;
#63082=VERTEX_POINT ( 'NONE', #39405 ) ;
#63083=TOROIDAL_SURFACE ( 'NONE', #2573, 1.000000000000000000, 0.5000000000000000000 ) ;
#63093=EDGE_LOOP ( 'NONE', ( #74009, #38010, #69805, #59700 ) ) ;
#63114=CARTESIAN_POINT ( 'NONE',  ( 165.4421947725420523, 249.5000000000000568, 22.46007009812167254 ) ) ;
#63117=ADVANCED_FACE ( 'NONE', ( #16265, #2531 ), #66922, .F. ) ;
#63139=EDGE_CURVE ( 'NONE', #4038, #85072, #68736, .T. ) ;
#63143=DIRECTION ( 'NONE',  ( -0.9693563597868444237, -0.2456588035076248677, 0.000000000000000000 ) ) ;
#63150=DIRECTION ( 'NONE',  ( -0.000000000000000000, 1.000000000000000000, -9.656854691831248164E-17 ) ) ;
#63152=DIRECTION ( 'NONE',  ( -0.5987926743825080500, -0.8009040723493942027, 0.000000000000000000 ) ) ;
#63155=CARTESIAN_POINT ( 'NONE',  ( 156.6695768423672632, 18.03393767897209443, -8.087387968559699658 ) ) ;
#63164=EDGE_CURVE ( 'NONE', #33465, #50260, #48776, .T. ) ;
#63169=CARTESIAN_POINT ( 'NONE',  ( 206.1919228894574303, 35.96217941443950394, 14.00000000000000000 ) ) ;
#63171=ORIENTED_EDGE ( 'NONE', *, *, #76146, .F. ) ;
#63188=LINE ( 'NONE', #12496, #90793 ) ;
#63203=ORIENTED_EDGE ( 'NONE', *, *, #36505, .F. ) ;
#63206=ORIENTED_EDGE ( 'NONE', *, *, #17291, .F. ) ;
#63223=ORIENTED_EDGE ( 'NONE', *, *, #66418, .F. ) ;
#63229=ORIENTED_EDGE ( 'NONE', *, *, #22620, .F. ) ;
#63231=EDGE_CURVE ( 'NONE', #30244, #77857, #66971, .T. ) ;
#63232=ORIENTED_EDGE ( 'NONE', *, *, #1762, .T. ) ;
#63234=AXIS2_PLACEMENT_3D ( 'NONE', #4334, #63538, #77242 ) ;
#63240=PLANE ( 'NONE',  #48707 ) ;
#63252=DIRECTION ( 'NONE',  ( 0.000000000000000000, 0.000000000000000000, 1.000000000000000000 ) ) ;
#63261=DIRECTION ( 'NONE',  ( -1.000000000000000000, 0.000000000000000000, 0.000000000000000000 ) ) ;
#63265=CARTESIAN_POINT ( 'NONE',  ( 138.6539576904058606, 275.5000000000000568, 10.50000000000000000 ) ) ;
#63278=FACE_OUTER_BOUND ( 'NONE', #66449, .T. ) ;
#63281=DIRECTION ( 'NONE',  ( 0.000000000000000000, 0.000000000000000000, 1.000000000000000000 ) ) ;
#63294=EDGE_CURVE ( 'NONE', #52690, #84307, #32162, .T. ) ;
#63300=CARTESIAN_POINT ( 'NONE',  ( 155.3967522965732257, 18.12362412296499770, 8.741384835539003362 ) ) ;
#63311=ORIENTED_EDGE ( 'NONE', *, *, #1954, .T. ) ;
#63321=DIRECTION ( 'NONE',  ( 0.000000000000000000, 1.000000000000000000, 0.000000000000000000 ) ) ;
#63322=CARTESIAN_POINT ( 'NONE',  ( 185.4166944662832179, 249.5000000000000568, 23.37680765314684095 ) ) ;
#63326=ORIENTED_EDGE ( 'NONE', *, *, #63818, .F. ) ;
#63335=ORIENTED_EDGE ( 'NONE', *, *, #19699, .T. ) ;
#63342=CARTESIAN_POINT ( 'NONE',  ( 154.1779308144228935, 20.65864417925001462, -13.49368544356955901 ) ) ;
#63343=CARTESIAN_POINT ( 'NONE',  ( 153.9079962421555763, 20.48904911123736383, 11.76949543550875354 ) ) ;
#63351=EDGE_CURVE ( 'NONE', #63777, #35022, #33258, .T. ) ;
#63352=DIRECTION ( 'NONE',  ( 0.000000000000000000, 1.000000000000000000, 0.000000000000000000 ) ) ;
#63354=ORIENTED_EDGE ( 'NONE', *, *, #30500, .T. ) ;
#63356=DIRECTION ( 'NONE',  ( 0.000000000000000000, 0.7071067811865561215, 0.7071067811865389130 ) ) ;
#63363=VECTOR ( 'NONE', #27610, 1000.000000000000000 ) ;
#63371=CARTESIAN_POINT ( 'NONE',  ( 175.2296996224750103, 140.2072866198470251, 0.000000000000000000 ) ) ;
#63372=LINE ( 'NONE', #53900, #6556 ) ;
#63385=CARTESIAN_POINT ( 'NONE',  ( 222.8344101925596306, 3.000000000000000000, 10.00000000000000000 ) ) ;
#63406=EDGE_CURVE ( 'NONE', #84959, #3069, #85078, .T. ) ;
#63409=ORIENTED_EDGE ( 'NONE', *, *, #80190, .T. ) ;
#63410=CARTESIAN_POINT ( 'NONE',  ( 151.9308040601938217, 19.99432900747112285, 6.268121358094561835 ) ) ;
#63412=CARTESIAN_POINT ( 'NONE',  ( 219.8344101925596021, 35.72494958537217968, 10.00000000000000000 ) ) ;
#63422=VERTEX_POINT ( 'NONE', #55522 ) ;
#63423=CARTESIAN_POINT ( 'NONE',  ( 194.7288575836260804, 39.67451392790587050, 14.01013636219982672 ) ) ;
#63426=CARTESIAN_POINT ( 'NONE',  ( 200.4551663812866025, 64.49084098423909950, -2.633798379906725273 ) ) ;
#63428=ORIENTED_EDGE ( 'NONE', *, *, #19673, .T. ) ;
#63435=DIRECTION ( 'NONE',  ( 0.000000000000000000, 0.000000000000000000, -1.000000000000000000 ) ) ;
#63436=CARTESIAN_POINT ( 'NONE',  ( 200.3186454232214828, 250.5000000000000568, -3.421094783296261710 ) ) ;
#63444=ORIENTED_EDGE ( 'NONE', *, *, #1761, .F. ) ;
#63453=ORIENTED_EDGE ( 'NONE', *, *, #47800, .F. ) ;
#63469=ORIENTED_EDGE ( 'NONE', *, *, #29709, .F. ) ;
#63470=ORIENTED_EDGE ( 'NONE', *, *, #20244, .T. ) ;
#63476=ADVANCED_FACE ( 'NONE', ( #41755 ), #19986, .T. ) ;
#63486=DIRECTION ( 'NONE',  ( 0.000000000000000000, 0.000000000000000000, -1.000000000000000000 ) ) ;
#63496=VECTOR ( 'NONE', #54499, 1000.000000000000000 ) ;
#63497=CARTESIAN_POINT ( 'NONE',  ( 209.6315158418980502, 36.17082498069705565, 14.26380412667038655 ) ) ;
#63508=CYLINDRICAL_SURFACE ( 'NONE', #1542, 5.000000000000000888 ) ;
#63521=ORIENTED_EDGE ( 'NONE', *, *, #80099, .T. ) ;
#63522=FACE_OUTER_BOUND ( 'NONE', #30589, .T. ) ;
#63535=ADVANCED_FACE ( 'NONE', ( #90519 ), #83573, .T. ) ;
#63537=CARTESIAN_POINT ( 'NONE',  ( 175.2296996224749250, 275.5000000000000568, -24.99999999999999289 ) ) ;
#63538=DIRECTION ( 'NONE',  ( -0.000000000000000000, -1.000000000000000000, -0.000000000000000000 ) ) ;
#63552=ORIENTED_EDGE ( 'NONE', *, *, #75701, .T. ) ;
#63559=CIRCLE ( 'NONE', #43843, 0.5000000000000009992 ) ;
#63562=ORIENTED_EDGE ( 'NONE', *, *, #25879, .T. ) ;
#63565=CIRCLE ( 'NONE', #30280, 1.000000000000006439 ) ;
#63570=DIRECTION ( 'NONE',  ( -1.000000000000000000, 0.000000000000000000, 0.000000000000000000 ) ) ;
#63576=ORIENTED_EDGE ( 'NONE', *, *, #51225, .F. ) ;
#63583=VERTEX_POINT ( 'NONE', #40799 ) ;
#63584=LINE ( 'NONE', #92409, #477 ) ;
#63587=EDGE_CURVE ( 'NONE', #48695, #13368, #17090, .T. ) ;
#63595=CARTESIAN_POINT ( 'NONE',  ( 0.000000000000000000, 3.000000000000000000, -10.00000000000000000 ) ) ;
#63611=CARTESIAN_POINT ( 'NONE',  ( 140.6539576904058606, 275.5000000000000568, -12.00000000000000000 ) ) ;
#63612=CARTESIAN_POINT ( 'NONE',  ( 153.2628468892384603, 20.37991841447901820, 11.93555113919331312 ) ) ;
#63618=CARTESIAN_POINT ( 'NONE',  ( 139.6539576904058606, 275.0000000000000568, -10.49999999999999822 ) ) ;
#63620=CARTESIAN_POINT ( 'NONE',  ( 160.5350683151633291, 250.0000000000000568, 20.22542485937379908 ) ) ;
#63622=DIRECTION ( 'NONE',  ( -0.000000000000000000, -0.000000000000000000, -1.000000000000000000 ) ) ;
#63625=CARTESIAN_POINT ( 'NONE',  ( 157.4851178187871312, 14.99999999999999467, -7.000000000000000888 ) ) ;
#63635=CIRCLE ( 'NONE', #22694, 5.568361562975243650 ) ;
#63636=VERTEX_POINT ( 'NONE', #76824 ) ;
#63640=FACE_OUTER_BOUND ( 'NONE', #62452, .T. ) ;
#63642=ORIENTED_EDGE ( 'NONE', *, *, #34990, .F. ) ;
#63657=DIRECTION ( 'NONE',  ( 5.551115123125777653E-14, 0.000000000000000000, 1.000000000000000000 ) ) ;
#63676=ORIENTED_EDGE ( 'NONE', *, *, #82014, .F. ) ;
#63694=ORIENTED_EDGE ( 'NONE', *, *, #31803, .T. ) ;
#63700=EDGE_LOOP ( 'NONE', ( #6329, #8967, #69251, #172 ) ) ;
#63702=EDGE_CURVE ( 'NONE', #33827, #67960, #12916, .T. ) ;
#63715=CARTESIAN_POINT ( 'NONE',  ( 0.000000000000000000, 15.00000000000000000, -9.000000000000001776 ) ) ;
#63727=DIRECTION ( 'NONE',  ( 1.000000000000000000, 0.000000000000000000, 0.000000000000000000 ) ) ;
#63745=CYLINDRICAL_SURFACE ( 'NONE', #60574, 3.842139515347647638 ) ;
#63746=CARTESIAN_POINT ( 'NONE',  ( 165.2494399300530290, 8.542400036368780647, 25.74970488511327815 ) ) ;
#63749=CARTESIAN_POINT ( 'NONE',  ( 201.2929949297285077, 65.04117685566218654, 7.250946725472672938 ) ) ;
#63762=ADVANCED_FACE ( 'NONE', ( #77290 ), #91942, .F. ) ;
#63767=AXIS2_PLACEMENT_3D ( 'NONE', #32059, #3652, #53361 ) ;
#63777=VERTEX_POINT ( 'NONE', #5342 ) ;
#63789=DIRECTION ( 'NONE',  ( 0.000000000000000000, 1.000000000000000000, -0.000000000000000000 ) ) ;
#63793=ORIENTED_EDGE ( 'NONE', *, *, #29767, .F. ) ;
#63806=EDGE_LOOP ( 'NONE', ( #90699, #20950, #67790, #93653, #81461 ) ) ;
#63807=DIRECTION ( 'NONE',  ( -0.000000000000000000, -0.000000000000000000, 1.000000000000000000 ) ) ;
#63809=FACE_OUTER_BOUND ( 'NONE', #35101, .T. ) ;
#63816=CARTESIAN_POINT ( 'NONE',  ( 189.9243309297870610, 250.5000000000000568, 24.72542485937349710 ) ) ;
#63818=EDGE_CURVE ( 'NONE', #82379, #64275, #63584, .T. ) ;
#63819=ORIENTED_EDGE ( 'NONE', *, *, #45978, .F. ) ;
#63820=VERTEX_POINT ( 'NONE', #27569 ) ;
#63834=CIRCLE ( 'NONE', #75892, 4.499999999999990230 ) ;
#63837=CARTESIAN_POINT ( 'NONE',  ( 196.6877655503061817, 293.7115289173626707, -7.999911143031724237 ) ) ;
#63838=LINE ( 'NONE', #20723, #54921 ) ;
#63852=CARTESIAN_POINT ( 'NONE',  ( 189.9243309297870610, 250.0000000000000568, 20.22542485937349355 ) ) ;
#63854=FACE_OUTER_BOUND ( 'NONE', #55298, .T. ) ;
#63866=CARTESIAN_POINT ( 'NONE',  ( 195.3516019189765132, 40.92429273362618858, 14.83660509754012047 ) ) ;
#63874=EDGE_LOOP ( 'NONE', ( #91211, #10291, #83399, #2986 ) ) ;
#63875=LINE ( 'NONE', #27882, #77183 ) ;
#63877=CARTESIAN_POINT ( 'NONE',  ( 208.7622976689241057, 29.39913517558109035, 13.48907645363312291 ) ) ;
#63880=ADVANCED_FACE ( 'NONE', ( #42217 ), #28506, .T. ) ;
#63888=ORIENTED_EDGE ( 'NONE', *, *, #69493, .F. ) ;
#63894=EDGE_LOOP ( 'NONE', ( #47083, #17204, #42529, #61906, #78587, #65103, #12786, #12659, #46149, #13591, #76197, #81576, #9445, #30437 ) ) ;
#63901=CYLINDRICAL_SURFACE ( 'NONE', #79092, 3.000000000000000888 ) ;
#63904=CARTESIAN_POINT ( 'NONE',  ( 196.7383257810085979, 42.27872732282705925, 11.00000000000000000 ) ) ;
#63907=CIRCLE ( 'NONE', #26137, 7.500000000000013323 ) ;
#63922=CARTESIAN_POINT ( 'NONE',  ( 175.2296996224750103, 154.6894116713782807, 0.000000000000000000 ) ) ;
#63936=ORIENTED_EDGE ( 'NONE', *, *, #23960, .F. ) ;
#63938=CARTESIAN_POINT ( 'NONE',  ( 165.2424497756046549, 214.5000000000000568, 22.91843887563435800 ) ) ;
#63953=CARTESIAN_POINT ( 'NONE',  ( 175.2296996224749250, 249.5000000000000568, -24.99999999999999289 ) ) ;
#63962=CARTESIAN_POINT ( 'NONE',  ( 175.2296996224750103, 140.2072866198470251, -21.95310499597075804 ) ) ;
#63964=CARTESIAN_POINT ( 'NONE',  ( 199.4757856505664790, 63.23505538068130249, 9.191047964627605538 ) ) ;
#63967=AXIS2_PLACEMENT_3D ( 'NONE', #35372, #44669, #92175 ) ;
#63973=VECTOR ( 'NONE', #37304, 1000.000000000000000 ) ;
#63977=CARTESIAN_POINT ( 'NONE',  ( 152.7546676148615745, 130.4533703983871931, 11.50000000000000000 ) ) ;
#63979=CARTESIAN_POINT ( 'NONE',  ( 198.5368075633269314, 65.94727227685316961, -10.76536576713345994 ) ) ;
#63991=CARTESIAN_POINT ( 'NONE',  ( 216.5288609127277084, 293.9636489450776935, -40.00000000000000711 ) ) ;
#63994=EDGE_CURVE ( 'NONE', #84679, #30244, #54930, .T. ) ;
#63995=ADVANCED_FACE ( 'NONE', ( #58331 ), #71131, .F. ) ;
#64007=CARTESIAN_POINT ( 'NONE',  ( 152.4536156746142410, 275.0000000000000568, -14.50000000000000000 ) ) ;
#64021=ORIENTED_EDGE ( 'NONE', *, *, #69913, .F. ) ;
#64023=VECTOR ( 'NONE', #59632, 1000.000000000000000 ) ;
#64029=AXIS2_PLACEMENT_3D ( 'NONE', #56496, #84865, #85807 ) ;
#64036=DIRECTION ( 'NONE',  ( 0.000000000000000000, 0.000000000000000000, 1.000000000000000000 ) ) ;
#64042=VERTEX_POINT ( 'NONE', #50261 ) ;
#64050=ORIENTED_EDGE ( 'NONE', *, *, #36204, .F. ) ;
#64051=CARTESIAN_POINT ( 'NONE',  ( 196.9534188175200029, 25.84350552936208700, 12.42857142857141994 ) ) ;
#64062=DIRECTION ( 'NONE',  ( -0.000000000000000000, -1.000000000000000000, -0.000000000000000000 ) ) ;
#64064=AXIS2_PLACEMENT_3D ( 'NONE', #82311, #17461, #46311 ) ;
#64073=CIRCLE ( 'NONE', #509, 2.000000000000000000 ) ;
#64080=DIRECTION ( 'NONE',  ( 0.000000000000000000, 1.000000000000000000, 0.000000000000000000 ) ) ;
#64081=CARTESIAN_POINT ( 'NONE',  ( 153.1901962297479827, 19.73438857712018901, 11.80184082122065981 ) ) ;
#64087=DIRECTION ( 'NONE',  ( -0.6056179655966483777, 0.7957555401921981852, 0.000000000000000000 ) ) ;
#64091=CARTESIAN_POINT ( 'NONE',  ( 156.1449889021179160, 250.0000000000000568, 16.91223866672558529 ) ) ;
#64094=CARTESIAN_POINT ( 'NONE',  ( 157.3189109369757261, 16.43186977800929682, -7.221609175748580967 ) ) ;
#64104=EDGE_CURVE ( 'NONE', #71459, #25330, #35276, .T. ) ;
#64106=EDGE_LOOP ( 'NONE', ( #66022, #22538, #13152, #55740, #32082, #73437, #62572, #71019, #13948, #23675, #9329, #82976, #55760, #65216, #66925, #91784, #8671, #46349, #27561, #5082, #53468, #30786 ) ) ;
#64110=LINE ( 'NONE', #56995, #33672 ) ;
#64114=ADVANCED_FACE ( 'NONE', ( #43626 ), #42726, .T. ) ;
#64117=VECTOR ( 'NONE', #9654, 1000.000000000000114 ) ;
#64128=AXIS2_PLACEMENT_3D ( 'NONE', #27012, #32717, #92327 ) ;
#64133=DIRECTION ( 'NONE',  ( -1.000000000000000000, 0.000000000000000000, 0.000000000000000000 ) ) ;
#64135=CIRCLE ( 'NONE', #73152, 4.999999999999984013 ) ;
#64142=DIRECTION ( 'NONE',  ( 0.000000000000000000, 0.000000000000000000, 1.000000000000000000 ) ) ;
#64149=EDGE_LOOP ( 'NONE', ( #54189, #89787, #42196, #42281 ) ) ;
#64152=ORIENTED_EDGE ( 'NONE', *, *, #49892, .F. ) ;
#64171=EDGE_LOOP ( 'NONE', ( #62503, #14533, #30920, #27066 ) ) ;
#64177=VERTEX_POINT ( 'NONE', #22780 ) ;
#64179=VERTEX_POINT ( 'NONE', #68210 ) ;
#64181=AXIS2_PLACEMENT_3D ( 'NONE', #15830, #72654, #59384 ) ;
#64187=DIRECTION ( 'NONE',  ( 0.000000000000000000, 0.000000000000000000, 1.000000000000000000 ) ) ;
#64191=EDGE_CURVE ( 'NONE', #4620, #56700, #15716, .T. ) ;
#64197=TOROIDAL_SURFACE ( 'NONE', #61186, 24.50000000000000355, 0.5000000000000000000 ) ;
#64202=CARTESIAN_POINT ( 'NONE',  ( 154.5625123364532101, 250.5000000000000568, 13.15740740740741899 ) ) ;
#64207=CARTESIAN_POINT ( 'NONE',  ( 151.4851178187871312, 21.00000000000000000, 0.000000000000000000 ) ) ;
#64220=ADVANCED_FACE ( 'NONE', ( #88092 ), #67290, .T. ) ;
#64227=FACE_OUTER_BOUND ( 'NONE', #48614, .T. ) ;
#64231=DIRECTION ( 'NONE',  ( 1.000000000000000000, 4.095251346825557639E-15, 0.000000000000000000 ) ) ;
#64260=ORIENTED_EDGE ( 'NONE', *, *, #9747, .T. ) ;
#64264=CONICAL_SURFACE ( 'NONE', #86914, 8.550761578869359170, 0.7853981633974639331 ) ;
#64271=CARTESIAN_POINT ( 'NONE',  ( 208.4306832106271088, -74.55766379199613425, 7.500000000000013323 ) ) ;
#64275=VERTEX_POINT ( 'NONE', #60185 ) ;
#64282=AXIS2_PLACEMENT_3D ( 'NONE', #60143, #81883, #80970 ) ;
#64289=DIRECTION ( 'NONE',  ( 0.000000000000000000, -0.000000000000000000, 1.000000000000000000 ) ) ;
#64290=CARTESIAN_POINT ( 'NONE',  ( 197.0544939925610777, 42.37846845930137363, 12.19834728626771891 ) ) ;
#64292=FACE_OUTER_BOUND ( 'NONE', #63700, .T. ) ;
#64300=VECTOR ( 'NONE', #81592, 1000.000000000000000 ) ;
#64304=CARTESIAN_POINT ( 'NONE',  ( 175.2296996224750103, 130.0000000000000568, 0.000000000000000000 ) ) ;
#64320=FACE_OUTER_BOUND ( 'NONE', #6150, .T. ) ;
#64332=CIRCLE ( 'NONE', #15897, 0.4999999999999989453 ) ;
#64334=LINE ( 'NONE', #63385, #84952 ) ;
#64337=CARTESIAN_POINT ( 'NONE',  ( 196.8803347170859865, 20.19615242270661426, 12.49999999999999289 ) ) ;
#64345=DIRECTION ( 'NONE',  ( 1.000000000000000000, -0.000000000000000000, -0.000000000000000000 ) ) ;
#64349=AXIS2_PLACEMENT_3D ( 'NONE', #63436, #20327, #13691 ) ;
#64352=CARTESIAN_POINT ( 'NONE',  ( 150.8012326218627948, 131.0000000000000568, -11.50000000000000000 ) ) ;
#64359=ADVANCED_FACE ( 'NONE', ( #81926 ), #45005, .F. ) ;
#64378=EDGE_CURVE ( 'NONE', #43923, #50859, #89717, .T. ) ;
#64386=CARTESIAN_POINT ( 'NONE',  ( 197.7363269526848057, 68.71792440747597652, -9.406972186202848363 ) ) ;
#64387=CARTESIAN_POINT ( 'NONE',  ( 138.6539576904058606, 132.0000000000000568, 10.50000000000000000 ) ) ;
#64395=ORIENTED_EDGE ( 'NONE', *, *, #38609, .F. ) ;
#64404=ORIENTED_EDGE ( 'NONE', *, *, #79357, .T. ) ;
#64420=ORIENTED_EDGE ( 'NONE', *, *, #36695, .T. ) ;
#64421=ORIENTED_EDGE ( 'NONE', *, *, #1899, .T. ) ;
#64436=FACE_OUTER_BOUND ( 'NONE', #16581, .T. ) ;
#64447=DIRECTION ( 'NONE',  ( 1.000000000000000000, 0.000000000000000000, 0.000000000000000000 ) ) ;
#64460=CARTESIAN_POINT ( 'NONE',  ( 197.0997303688997704, 71.85475162903931334, -12.14496016938517009 ) ) ;
#64489=CARTESIAN_POINT ( 'NONE',  ( 175.2296996224750103, 214.5000000000000568, 0.000000000000000000 ) ) ;
#64501=VERTEX_POINT ( 'NONE', #59246 ) ;
#64510=ORIENTED_EDGE ( 'NONE', *, *, #69553, .T. ) ;
#64516=CARTESIAN_POINT ( 'NONE',  ( 175.2296996224750103, 154.6894116713782807, 0.000000000000000000 ) ) ;
#64522=ORIENTED_EDGE ( 'NONE', *, *, #50647, .F. ) ;
#64530=CARTESIAN_POINT ( 'NONE',  ( 196.5570723171844350, 25.86847754248514875, 12.83135264428034539 ) ) ;
#64547=ADVANCED_FACE ( 'NONE', ( #74854 ), #21696, .T. ) ;
#64559=DIRECTION ( 'NONE',  ( 0.000000000000000000, 0.000000000000000000, 1.000000000000000000 ) ) ;
#64565=DIRECTION ( 'NONE',  ( -1.000000000000000000, 0.000000000000000000, 0.000000000000000000 ) ) ;
#64567=CARTESIAN_POINT ( 'NONE',  ( 159.4851178187871312, 17.43233815881133708, -9.000000000000000000 ) ) ;
#64570=DIRECTION ( 'NONE',  ( 0.000000000000000000, 1.000000000000000000, 0.000000000000000000 ) ) ;
#64571=CARTESIAN_POINT ( 'NONE',  ( 157.3811296300184210, 16.14910309754964501, -7.138650918358436570 ) ) ;
#64581=EDGE_LOOP ( 'NONE', ( #48355, #55759, #22772, #5448 ) ) ;
#64584=CARTESIAN_POINT ( 'NONE',  ( 197.5046084229020096, 41.86576550531665930, 12.19218485022636855 ) ) ;
#64586=ORIENTED_EDGE ( 'NONE', *, *, #76026, .F. ) ;
#64596=ORIENTED_EDGE ( 'NONE', *, *, #27071, .T. ) ;
#64636=ORIENTED_EDGE ( 'NONE', *, *, #68796, .T. ) ;
#64653=CARTESIAN_POINT ( 'NONE',  ( 222.8344101925596306, 0.000000000000000000, 10.00000000000000000 ) ) ;
#64665=PLANE ( 'NONE',  #20061 ) ;
#64669=PLANE ( 'NONE',  #83709 ) ;
#64672=PLANE ( 'NONE',  #73869 ) ;
#64687=CARTESIAN_POINT ( 'NONE',  ( 185.2169494693457921, 275.0000000000000568, 22.91843887563416615 ) ) ;
#64718=EDGE_CURVE ( 'NONE', #73473, #75506, #85040, .T. ) ;
#64726=DIRECTION ( 'NONE',  ( -0.000000000000000000, 1.000000000000000000, 0.000000000000000000 ) ) ;
#64731=EDGE_LOOP ( 'NONE', ( #45690, #55393, #85896, #5795 ) ) ;
#64739=ORIENTED_EDGE ( 'NONE', *, *, #30011, .F. ) ;
#64743=ORIENTED_EDGE ( 'NONE', *, *, #75497, .F. ) ;
#64747=EDGE_CURVE ( 'NONE', #93704, #38347, #26522, .T. ) ;
#64748=DIRECTION ( 'NONE',  ( 0.9764705882352960886, 0.000000000000000000, 0.2156506209390900708 ) ) ;
#64755=CARTESIAN_POINT ( 'NONE',  ( 209.1021009645937738, 27.84274218592230810, 12.05941621939738084 ) ) ;
#64756=DIRECTION ( 'NONE',  ( -0.000000000000000000, 0.000000000000000000, -1.000000000000000000 ) ) ;
#64760=ORIENTED_EDGE ( 'NONE', *, *, #34566, .F. ) ;
#64764=ADVANCED_FACE ( 'NONE', ( #25570 ), #63003, .F. ) ;
#64776=CARTESIAN_POINT ( 'NONE',  ( 193.6552470326849402, 275.5797763526087465, 16.89672165344822474 ) ) ;
#64777=CARTESIAN_POINT ( 'NONE',  ( 195.4781563537916043, 27.48493576247232895, 13.99999999999999822 ) ) ;
#64790=CARTESIAN_POINT ( 'NONE',  ( 152.4536156746142410, 275.0000000000000568, 11.49999999999999289 ) ) ;
#64792=CARTESIAN_POINT ( 'NONE',  ( 180.2288731078812702, 215.0000000000000568, -24.90909090909092782 ) ) ;
#64803=CARTESIAN_POINT ( 'NONE',  ( 156.4851178187871596, 16.95599219719301232, 6.999999999999998224 ) ) ;
#64817=VERTEX_POINT ( 'NONE', #55410 ) ;
#64818=CARTESIAN_POINT ( 'NONE',  ( 200.2349812190172713, 66.43136063442169359, 7.741079165001063522 ) ) ;
#64820=FACE_OUTER_BOUND ( 'NONE', #92496, .T. ) ;
#64829=ORIENTED_EDGE ( 'NONE', *, *, #5338, .T. ) ;
#64830=CARTESIAN_POINT ( 'NONE',  ( 194.6889851074543287, 41.25212764115960340, 14.04815903671776312 ) ) ;
#64836=ORIENTED_EDGE ( 'NONE', *, *, #1671, .F. ) ;
#64842=CARTESIAN_POINT ( 'NONE',  ( 196.1825486463387165, 72.66602830303396843, -11.70860092535009045 ) ) ;
#64843=CARTESIAN_POINT ( 'NONE',  ( 196.6877655503061533, 293.9636489450776367, -44.00000000000000000 ) ) ;
#64853=VERTEX_POINT ( 'NONE', #33612 ) ;
#64861=ADVANCED_FACE ( 'NONE', ( #47328 ), #91833, .T. ) ;
#64865=DIRECTION ( 'NONE',  ( 0.000000000000000000, 0.000000000000000000, -1.000000000000000000 ) ) ;
#64878=EDGE_LOOP ( 'NONE', ( #85973, #20567, #51506, #6733 ) ) ;
#64879=EDGE_LOOP ( 'NONE', ( #42185, #49088, #12968, #77652 ) ) ;
#64880=CARTESIAN_POINT ( 'NONE',  ( 170.8178014930282700, 8.542400036368780647, 9.000000000000001776 ) ) ;
#64895=CARTESIAN_POINT ( 'NONE',  ( 208.4306832106271088, 1.000000000000000888, 0.000000000000000000 ) ) ;
#64896=CARTESIAN_POINT ( 'NONE',  ( 153.9133111279456045, 20.47222690886501795, -13.06183683676589524 ) ) ;
#64905=CARTESIAN_POINT ( 'NONE',  ( 199.0061125298537377, 215.0000000000000568, -7.725424859374024678 ) ) ;
#64916=CARTESIAN_POINT ( 'NONE',  ( 154.9842916688210153, 128.0000000000000568, 12.88888888888890349 ) ) ;
#64918=CARTESIAN_POINT ( 'NONE',  ( 197.7156983550588052, 70.58049492527801760, -11.36724305494472453 ) ) ;
#64919=CARTESIAN_POINT ( 'NONE',  ( 0.000000000000000000, 15.00000000000000000, 15.00000000000000000 ) ) ;
#64928=AXIS2_PLACEMENT_3D ( 'NONE', #52728, #89632, #38535 ) ;
#64945=CARTESIAN_POINT ( 'NONE',  ( 219.8344101925596021, 35.72494958537217968, 7.000000000000000000 ) ) ;
#64946=EDGE_CURVE ( 'NONE', #14859, #92829, #30750, .T. ) ;
#64947=DIRECTION ( 'NONE',  ( 1.000000000000000000, 0.000000000000000000, 0.000000000000000000 ) ) ;
#64986=DIRECTION ( 'NONE',  ( 0.000000000000000000, 0.000000000000000000, 1.000000000000000000 ) ) ;
#64999=VECTOR ( 'NONE', #69282, 1000.000000000000000 ) ;
#65006=EDGE_CURVE ( 'NONE', #52785, #48386, #91206, .T. ) ;
#65011=EDGE_CURVE ( 'NONE', #9610, #10831, #80607, .T. ) ;
#65014=CARTESIAN_POINT ( 'NONE',  ( 201.2104617360081704, 15.00000000000000000, -10.00000000000000000 ) ) ;
#65021=CARTESIAN_POINT ( 'NONE',  ( 197.0327713505838290, 40.95653769364759711, 12.25939981568760295 ) ) ;
#65024=CARTESIAN_POINT ( 'NONE',  ( 154.1415209985679269, 20.37991841447902175, -11.45812909362557619 ) ) ;
#65025=FACE_OUTER_BOUND ( 'NONE', #16719, .T. ) ;
#65034=VERTEX_POINT ( 'NONE', #40686 ) ;
#65053=VECTOR ( 'NONE', #24115, 1000.000000000000000 ) ;
#65055=DIRECTION ( 'NONE',  ( 0.000000000000000000, 0.000000000000000000, 1.000000000000000000 ) ) ;
#65058=VECTOR ( 'NONE', #61564, 1000.000000000000000 ) ;
#65063=EDGE_CURVE ( 'NONE', #20922, #15791, #90541, .T. ) ;
#65065=EDGE_CURVE ( 'NONE', #24040, #21372, #46867, .T. ) ;
#65076=VERTEX_POINT ( 'NONE', #18469 ) ;
#65093=VERTEX_POINT ( 'NONE', #75771 ) ;
#65100=ORIENTED_EDGE ( 'NONE', *, *, #78211, .F. ) ;
#65103=ORIENTED_EDGE ( 'NONE', *, *, #13330, .F. ) ;
#65112=DIRECTION ( 'NONE',  ( 0.000000000000000000, 0.000000000000000000, -1.000000000000000000 ) ) ;
#65117=FACE_OUTER_BOUND ( 'NONE', #37875, .T. ) ;
#65123=CARTESIAN_POINT ( 'NONE',  ( 156.4947056272797852, 20.00000000000000000, 15.00000000000000000 ) ) ;
#65125=AXIS2_PLACEMENT_3D ( 'NONE', #25279, #89650, #31461 ) ;
#65132=DIRECTION ( 'NONE',  ( 0.000000000000000000, 1.000000000000000000, 0.000000000000000000 ) ) ;
#65136=CARTESIAN_POINT ( 'NONE',  ( 194.7453183674699915, 20.99999999999998934, -15.62500000000000355 ) ) ;
#65176=( BOUNDED_CURVE ( )  B_SPLINE_CURVE ( 3, ( #34491, #62926, #41078, #33534 ),
 .UNSPECIFIED., .F., .F. ) 
 B_SPLINE_CURVE_WITH_KNOTS ( ( 4, 4 ),
 ( 0.000000000000000000, 1.570796326794896336 ),
 .UNSPECIFIED. ) 
 CURVE ( )  GEOMETRIC_REPRESENTATION_ITEM ( )  RATIONAL_B_SPLINE_CURVE ( ( 1.000000000000000000, 0.8047378541243650485, 0.8047378541243650485, 1.000000000000000000 ) ) 
 REPRESENTATION_ITEM ( '' )  );
#65181=( BOUNDED_SURFACE ( )  B_SPLINE_SURFACE ( 3, 2, ( 
 ( #10688, #83585, #60907 ),
 ( #69396, #39087, #25829 ),
 ( #4528, #19209, #47124 ),
 ( #47607, #17809, #91631 ) ),
 .UNSPECIFIED., .F., .F., .F. ) 
 B_SPLINE_SURFACE_WITH_KNOTS ( ( 4, 4 ),
 ( 3, 3 ),
 ( 0.000000000000000000, 0.0009300155619514785879 ),
 ( 0.000000000000000000, 1.000000000000000000 ),
 .UNSPECIFIED. ) 
 GEOMETRIC_REPRESENTATION_ITEM ( )  RATIONAL_B_SPLINE_SURFACE ( (
 ( 1.000000000000000000, 0.8255171224912133399, 1.000000000000000000),
 ( 1.000000000000000000, 0.8158797882023690606, 1.000000000000000000),
 ( 1.000000000000000000, 0.8010468905540648610, 1.000000000000000000),
 ( 1.000000000000000000, 0.7827533893365004047, 1.000000000000000000) ) ) 
 REPRESENTATION_ITEM ( '' )  SURFACE ( )  );
#65192=AXIS2_PLACEMENT_3D ( 'NONE', #35687, #86783, #80605 ) ;
#65211=CARTESIAN_POINT ( 'NONE',  ( 208.9602656640649627, 27.80679762345980421, 14.02415587114433393 ) ) ;
#65212=FACE_OUTER_BOUND ( 'NONE', #18360, .T. ) ;
#65214=CYLINDRICAL_SURFACE ( 'NONE', #5117, 0.5000000000000004441 ) ;
#65216=ORIENTED_EDGE ( 'NONE', *, *, #45526, .F. ) ;
#65217=CARTESIAN_POINT ( 'NONE',  ( 219.8344101925596021, 3.000000000000000000, 10.00000000000000000 ) ) ;
#65247=DIRECTION ( 'NONE',  ( 0.000000000000000000, 1.000000000000000000, 0.000000000000000000 ) ) ;
#65257=CYLINDRICAL_SURFACE ( 'NONE', #51747, 0.5000000000000004441 ) ;
#65268=EDGE_CURVE ( 'NONE', #12757, #88799, #39313, .T. ) ;
#65271=ORIENTED_EDGE ( 'NONE', *, *, #66484, .T. ) ;
#65274=DIRECTION ( 'NONE',  ( -1.000000000000000000, 0.000000000000000000, 0.000000000000000000 ) ) ;
#65284=EDGE_LOOP ( 'NONE', ( #78236, #91934, #23000, #61976, #37561, #89102, #80768, #92166, #63203, #28283, #76542 ) ) ;
#65285=DIRECTION ( 'NONE',  ( 0.6056179655966478226, -0.7957555401921982963, -0.000000000000000000 ) ) ;
#65290=EDGE_CURVE ( 'NONE', #69004, #49537, #47205, .T. ) ;
#65297=FACE_OUTER_BOUND ( 'NONE', #59295, .T. ) ;
#65309=EDGE_CURVE ( 'NONE', #34178, #87468, #90148, .T. ) ;
#65320=TOROIDAL_SURFACE ( 'NONE', #10851, 4.499999999999990230, 0.5000000000000000000 ) ;
#65327=EDGE_CURVE ( 'NONE', #60755, #78077, #9562, .T. ) ;
#65334=AXIS2_PLACEMENT_3D ( 'NONE', #29238, #50544, #78502 ) ;
#65337=ORIENTED_EDGE ( 'NONE', *, *, #12869, .T. ) ;
#65338=EDGE_LOOP ( 'NONE', ( #50110, #12265, #21040 ) ) ;
#65352=CARTESIAN_POINT ( 'NONE',  ( 139.1539576904058606, 250.0000000000000568, -10.49999999999999822 ) ) ;
#65353=CARTESIAN_POINT ( 'NONE',  ( 164.6329196456214277, 214.9910457053126720, 23.09031830825856346 ) ) ;
#65365=CARTESIAN_POINT ( 'NONE',  ( 202.8019728163925492, 61.40723988820080592, 6.999999999999999112 ) ) ;
#65373=DIRECTION ( 'NONE',  ( 1.000000000000000000, 0.000000000000000000, 5.880589007913310608E-16 ) ) ;
#65376=CARTESIAN_POINT ( 'NONE',  ( 185.4166944662832179, 250.0000000000000568, 23.37680765314684095 ) ) ;
#65377=CARTESIAN_POINT ( 'NONE',  ( 169.7306087885279453, 275.0000000000000568, -24.89999999999999147 ) ) ;
#65384=ADVANCED_FACE ( 'NONE', ( #93706 ), #36826, .T. ) ;
#65387=EDGE_LOOP ( 'NONE', ( #90983, #6722, #3922, #54974 ) ) ;
#65388=DIRECTION ( 'NONE',  ( 1.000000000000000000, 0.000000000000000000, -0.000000000000000000 ) ) ;
#65394=CIRCLE ( 'NONE', #32105, 7.910944475430059519 ) ;
#65403=FACE_OUTER_BOUND ( 'NONE', #22215, .T. ) ;
#65405=CARTESIAN_POINT ( 'NONE',  ( 185.4166944662832179, 275.0000000000000568, 23.37680765314684450 ) ) ;
#65424=ORIENTED_EDGE ( 'NONE', *, *, #89197, .F. ) ;
#65443=CARTESIAN_POINT ( 'NONE',  ( 195.5206343625570753, 25.57665861450641742, 12.82293366630988629 ) ) ;
#65456=CARTESIAN_POINT ( 'NONE',  ( 156.4947056272797852, 21.00000000000000000, 15.00000000000000000 ) ) ;
#65467=ADVANCED_FACE ( 'NONE', ( #21764 ), #7089, .F. ) ;
#65470=CARTESIAN_POINT ( 'NONE',  ( 195.6096107219261171, 24.54133239209091499, 12.68062660795851571 ) ) ;
#65479=DIRECTION ( 'NONE',  ( 0.000000000000000000, 1.000000000000000000, 0.000000000000000000 ) ) ;
#65482=DIRECTION ( 'NONE',  ( 0.000000000000000000, 1.000000000000000000, 0.000000000000000000 ) ) ;
#65483=CARTESIAN_POINT ( 'NONE',  ( 157.1544330182169347, 16.98551211945809669, -7.440913067426857985 ) ) ;
#65495=CARTESIAN_POINT ( 'NONE',  ( 197.0539037881910929, 24.40160077877072098, 12.19936955022341607 ) ) ;
#65509=CARTESIAN_POINT ( 'NONE',  ( 200.1087902362374678, 299.5637500031161267, -5.714653251563827752 ) ) ;
#65513=CIRCLE ( 'NONE', #44312, 25.00000000000000355 ) ;
#65525=CIRCLE ( 'NONE', #18650, 5.103083949679981579 ) ;
#65536=VECTOR ( 'NONE', #17226, 1000.000000000000000 ) ;
#65555=ORIENTED_EDGE ( 'NONE', *, *, #49649, .T. ) ;
#65559=CIRCLE ( 'NONE', #21655, 4.025000000000000355 ) ;
#65568=UNCERTAINTY_MEASURE_WITH_UNIT (LENGTH_MEASURE( 1.000000000000000082E-05 ), #41729, 'distance_accuracy_value', 'NONE');
#65576=CARTESIAN_POINT ( 'NONE',  ( 198.2695878509457543, 40.57393790395538247, 11.03083405179679666 ) ) ;
#65581=DIRECTION ( 'NONE',  ( 0.5877852522924685852, 0.000000000000000000, -0.8090169943749507819 ) ) ;
#65589=AXIS2_PLACEMENT_3D ( 'NONE', #74280, #81841, #61030 ) ;
#65594=CIRCLE ( 'NONE', #38304, 3.000000000000000000 ) ;
#65603=CIRCLE ( 'NONE', #24739, 2.000000000000007105 ) ;
#65608=AXIS2_PLACEMENT_3D ( 'NONE', #18047, #70128, #5264 ) ;
#65612=DIRECTION ( 'NONE',  ( 0.000000000000000000, -0.000000000000000000, 1.000000000000000000 ) ) ;
#65618=B_SPLINE_CURVE_WITH_KNOTS ( 'NONE', 3,
 ( #37890, #36515, #79618, #16598, #14760, #66795, #38363, #58317 ),
 .UNSPECIFIED., .F., .F.,
 ( 4, 2, 2, 4 ),
 ( 0.000000000000000000, 0.001028958187123778451, 0.001543437280685668002, 0.002057916374247557769 ),
 .UNSPECIFIED. ) ;
#65620=VECTOR ( 'NONE', #6566, 1000.000000000000000 ) ;
#65647=EDGE_CURVE ( 'NONE', #34882, #17985, #43971, .T. ) ;
#65662=AXIS2_PLACEMENT_3D ( 'NONE', #57775, #21791, #21311 ) ;
#65669=ORIENTED_EDGE ( 'NONE', *, *, #17385, .T. ) ;
#65670=DIRECTION ( 'NONE',  ( -0.01818181818182024526, 0.000000000000000000, -0.9998346970812742596 ) ) ;
#65671=VECTOR ( 'NONE', #54834, 1000.000000000000000 ) ;
#65672=AXIS2_PLACEMENT_3D ( 'NONE', #49547, #93553, #6002 ) ;
#65674=CIRCLE ( 'NONE', #52051, 4.999999999999990230 ) ;
#65679=CARTESIAN_POINT ( 'NONE',  ( 183.0442525570908288, 264.6571197653884155, -7.500000000000000000 ) ) ;
#65685=EDGE_LOOP ( 'NONE', ( #89224, #10969, #30356, #50008 ) ) ;
#65686=FACE_OUTER_BOUND ( 'NONE', #57704, .T. ) ;
#65702=DIRECTION ( 'NONE',  ( 0.000000000000000000, 0.000000000000000000, 1.000000000000000000 ) ) ;
#65710=DIRECTION ( 'NONE',  ( 0.000000000000000000, 1.000000000000000000, 0.000000000000000000 ) ) ;
#65711=CARTESIAN_POINT ( 'NONE',  ( 185.0172044724083946, 249.5000000000000568, 22.46007009812148425 ) ) ;
#65721=AXIS2_PLACEMENT_3D ( 'NONE', #25248, #60320, #32820 ) ;
#65730=( BOUNDED_SURFACE ( )  B_SPLINE_SURFACE ( 3, 2, ( 
 ( #1378, #60092, #81369 ),
 ( #88931, #32126, #52955 ),
 ( #38749, #59152, #60552 ),
 ( #89390, #39198, #68110 ),
 ( #3236, #89868, #25028 ),
 ( #80442, #19315, #12209 ) ),
 .UNSPECIFIED., .F., .F., .F. ) 
 B_SPLINE_SURFACE_WITH_KNOTS ( ( 4, 2, 4 ),
 ( 3, 3 ),
 ( 0.000000000000000000, 0.001526582434089621522, 0.003053164868179243045 ),
 ( 0.000000000000000000, 1.000000000000000000 ),
 .UNSPECIFIED. ) 
 GEOMETRIC_REPRESENTATION_ITEM ( )  RATIONAL_B_SPLINE_SURFACE ( (
 ( 1.000000000000000000, 0.7071067811865483499, 1.000000000000000000),
 ( 1.000000000000000000, 0.7219865977747251806, 1.000000000000000000),
 ( 1.000000000000000000, 0.7353530398653037592, 1.000000000000000000),
 ( 1.000000000000000000, 0.7593109839641446479, 1.000000000000000000),
 ( 1.000000000000000000, 0.7699014431358679467, 1.000000000000000000),
 ( 1.000000000000000000, 0.7791885400064305633, 1.000000000000000000) ) ) 
 REPRESENTATION_ITEM ( '' )  SURFACE ( )  );
#65745=CARTESIAN_POINT ( 'NONE',  ( 197.8641554550088131, 70.83050013377537368, 10.83773308182944106 ) ) ;
#65747=DIRECTION ( 'NONE',  ( 0.000000000000000000, 0.000000000000000000, -1.000000000000000000 ) ) ;
#65755=CIRCLE ( 'NONE', #12822, 4.999999999999990230 ) ;
#65768=CARTESIAN_POINT ( 'NONE',  ( 209.7513585654923816, 282.2246705312486483, -40.00000000000000711 ) ) ;
#65773=VERTEX_POINT ( 'NONE', #63938 ) ;
#65802=VERTEX_POINT ( 'NONE', #92776 ) ;
#65803=ORIENTED_EDGE ( 'NONE', *, *, #42272, .F. ) ;
#65804=CARTESIAN_POINT ( 'NONE',  ( 197.1285099842352508, 19.08195175179129066, -12.05325424581438121 ) ) ;
#65821=EDGE_CURVE ( 'NONE', #3069, #80198, #22411, .T. ) ;
#65822=FACE_OUTER_BOUND ( 'NONE', #51193, .T. ) ;
#65834=CARTESIAN_POINT ( 'NONE',  ( 160.5350683151633291, 250.0000000000000568, 20.22542485937379908 ) ) ;
#65836=CARTESIAN_POINT ( 'NONE',  ( 151.0889892289287388, 131.0000000000000284, 11.50000000000000000 ) ) ;
#65856=VERTEX_POINT ( 'NONE', #64880 ) ;
#65857=CARTESIAN_POINT ( 'NONE',  ( 156.5440870305766055, 215.0000000000000568, 17.21343741151179429 ) ) ;
#65859=CARTESIAN_POINT ( 'NONE',  ( 210.8848006936870263, 293.9636489450776367, -54.00000000000000000 ) ) ;
#65868=ORIENTED_EDGE ( 'NONE', *, *, #66040, .F. ) ;
#65883=AXIS2_PLACEMENT_3D ( 'NONE', #72741, #88329, #81226 ) ;
#65884=ORIENTED_EDGE ( 'NONE', *, *, #793, .F. ) ;
#65891=VERTEX_POINT ( 'NONE', #66701 ) ;
#65897=DIRECTION ( 'NONE',  ( 0.000000000000000000, 0.000000000000000000, 1.000000000000000000 ) ) ;
#65911=DIRECTION ( 'NONE',  ( 0.000000000000000000, 0.000000000000000000, 1.000000000000000000 ) ) ;
#65915=ADVANCED_FACE ( 'NONE', ( #52479 ), #43304, .T. ) ;
#65936=DIRECTION ( 'NONE',  ( -0.3024135303179549816, -0.9531768234071953394, 0.000000000000000000 ) ) ;
#65944=DIRECTION ( 'NONE',  ( 0.000000000000000000, 1.000000000000000000, 0.000000000000000000 ) ) ;
#65947=CARTESIAN_POINT ( 'NONE',  ( 195.1467215189997546, 26.67165171595035389, 15.11006648940266039 ) ) ;
#65948=DIRECTION ( 'NONE',  ( 0.000000000000000000, -1.000000000000000000, 0.000000000000000000 ) ) ;
#65958=DIRECTION ( 'NONE',  ( 1.000000000000000000, 0.000000000000000000, 0.000000000000000000 ) ) ;
#65976=FACE_OUTER_BOUND ( 'NONE', #13779, .T. ) ;
#65990=ORIENTED_EDGE ( 'NONE', *, *, #73681, .F. ) ;
#66019=ORIENTED_EDGE ( 'NONE', *, *, #16970, .F. ) ;
#66022=ORIENTED_EDGE ( 'NONE', *, *, #72919, .T. ) ;
#66023=EDGE_CURVE ( 'NONE', #16112, #5855, #77773, .T. ) ;
#66033=LINE ( 'NONE', #93482, #21549 ) ;
#66038=CARTESIAN_POINT ( 'NONE',  ( 209.7064572754725873, 36.40703279031890816, 14.69807322781363546 ) ) ;
#66040=EDGE_CURVE ( 'NONE', #10890, #9221, #3499, .T. ) ;
#66048=CARTESIAN_POINT ( 'NONE',  ( 151.2975037349265790, 130.0000000000000568, -12.50000000000000000 ) ) ;
#66051=DIRECTION ( 'NONE',  ( 2.220446049250312686E-15, 0.000000000000000000, 1.000000000000000000 ) ) ;
#66060=EDGE_CURVE ( 'NONE', #87290, #87519, #8917, .T. ) ;
#66064=ORIENTED_EDGE ( 'NONE', *, *, #31573, .T. ) ;
#66088=LINE ( 'NONE', #73641, #54456 ) ;
#66104=EDGE_CURVE ( 'NONE', #17769, #36764, #92785, .T. ) ;
#66110=DIRECTION ( 'NONE',  ( 0.000000000000000000, 1.000000000000000000, 0.000000000000000000 ) ) ;
#66124=CARTESIAN_POINT ( 'NONE',  ( 152.4536156746142410, 275.0000000000000568, -12.49999999999999289 ) ) ;
#66130=DIRECTION ( 'NONE',  ( 0.000000000000000000, 1.000000000000000000, 0.000000000000000000 ) ) ;
#66136=CARTESIAN_POINT ( 'NONE',  ( 196.0143093133015384, 24.42324672360809856, 11.99999999999998934 ) ) ;
#66147=DIRECTION ( 'NONE',  ( 0.000000000000000000, 0.000000000000000000, 1.000000000000000000 ) ) ;
#66150=EDGE_CURVE ( 'NONE', #50859, #43923, #18710, .T. ) ;
#66157=CARTESIAN_POINT ( 'NONE',  ( 159.4851178187871312, 3.000000000000000000, -10.00000000000000000 ) ) ;
#66162=EDGE_CURVE ( 'NONE', #31737, #2308, #12193, .T. ) ;
#66163=DIRECTION ( 'NONE',  ( -0.000000000000000000, 1.000000000000000000, -0.000000000000000000 ) ) ;
#66187=CARTESIAN_POINT ( 'NONE',  ( 197.0504801697426274, 72.68537487628056226, 12.20529943163058384 ) ) ;
#66189=DIRECTION ( 'NONE',  ( -0.000000000000000000, -1.000000000000000000, -0.000000000000000000 ) ) ;
#66215=ORIENTED_EDGE ( 'NONE', *, *, #90373, .T. ) ;
#66216=ADVANCED_FACE ( 'NONE', ( #68095 ), #77882, .T. ) ;
#66230=DIRECTION ( 'NONE',  ( 0.000000000000000000, 0.000000000000000000, 1.000000000000000000 ) ) ;
#66233=CARTESIAN_POINT ( 'NONE',  ( 156.8041522122653930, 250.4202232226203648, 16.89672165344857646 ) ) ;
#66234=CARTESIAN_POINT ( 'NONE',  ( 175.2296996224750103, 20.00000000000000000, 15.00000000000000000 ) ) ;
#66242=CARTESIAN_POINT ( 'NONE',  ( 197.4487343191780440, 71.87628676167049946, -11.52796263498073159 ) ) ;
#66247=ORIENTED_EDGE ( 'NONE', *, *, #47379, .T. ) ;
#66248=CARTESIAN_POINT ( 'NONE',  ( 196.7775620068246951, 42.35718252767666314, 12.67800755580416450 ) ) ;
#66273=( BOUNDED_SURFACE ( )  B_SPLINE_SURFACE ( 3, 2, ( 
 ( #70983, #71453, #48709 ),
 ( #92736, #27908, #35924 ),
 ( #56309, #6589, #85174 ),
 ( #35467, #77612, #49195 ),
 ( #21247, #36384, #64386 ),
 ( #29291, #92263, #28363 ),
 ( #50116, #58187, #41604 ),
 ( #57255, #79012, #14166 ),
 ( #71933, #64842, #51048 ),
 ( #87940, #23575, #23092 ) ),
 .UNSPECIFIED., .F., .F., .F. ) 
 B_SPLINE_SURFACE_WITH_KNOTS ( ( 4, 2, 2, 2, 4 ),
 ( 3, 3 ),
 ( 0.000000000000000000, 0.002512116609398717254, 0.005024233218797434508, 0.007536349828196151762, 0.01004846643759486902 ),
 ( 0.000000000000000000, 1.000000000000000000 ),
 .UNSPECIFIED. ) 
 GEOMETRIC_REPRESENTATION_ITEM ( )  RATIONAL_B_SPLINE_SURFACE ( (
 ( 1.000000000000000000, 0.8168508380123967738, 1.000000000000000000),
 ( 1.000000000000000000, 0.8469983227716593177, 1.000000000000000000),
 ( 1.000000000000000000, 0.8738795229725790925, 1.000000000000000000),
 ( 1.000000000000000000, 0.9200744724124843010, 1.000000000000000000),
 ( 1.000000000000000000, 0.9393932456996403335, 1.000000000000000000),
 ( 1.000000000000000000, 0.9701270577444791599, 1.000000000000000000),
 ( 1.000000000000000000, 0.9814990972770829547, 1.000000000000000000),
 ( 1.000000000000000000, 0.9964108658798418450, 1.000000000000000000),
 ( 1.000000000000000000, 1.000001410412884040, 1.000000000000000000),
 ( 1.000000000000000000, 1.000000000000000000, 1.000000000000000000) ) ) 
 REPRESENTATION_ITEM ( '' )  SURFACE ( )  );
#66275=DIRECTION ( 'NONE',  ( 0.000000000000000000, 1.000000000000000000, 0.000000000000000000 ) ) ;
#66277=EDGE_CURVE ( 'NONE', #89964, #13924, #8162, .T. ) ;
#66278=CARTESIAN_POINT ( 'NONE',  ( 156.4217629211117355, 119.0463968525363327, 9.000000000000001776 ) ) ;
#66300=CARTESIAN_POINT ( 'NONE',  ( 199.1087447750284980, 64.61450673763175701, -10.46317447812566392 ) ) ;
#66313=ORIENTED_EDGE ( 'NONE', *, *, #21333, .T. ) ;
#66318=CIRCLE ( 'NONE', #14946, 3.842139515347647638 ) ;
#66323=EDGE_CURVE ( 'NONE', #27549, #86758, #53884, .T. ) ;
#66330=EDGE_LOOP ( 'NONE', ( #55716, #25260, #8524, #24529 ) ) ;
#66344=CARTESIAN_POINT ( 'NONE',  ( 165.4284657918965991, 2.965303559109564446, 10.00000000000000000 ) ) ;
#66355=ORIENTED_EDGE ( 'NONE', *, *, #81253, .F. ) ;
#66356=CARTESIAN_POINT ( 'NONE',  ( 202.9738562182569694, 293.9636489450776367, -40.00000000000000711 ) ) ;
#66372=ORIENTED_EDGE ( 'NONE', *, *, #608, .F. ) ;
#66379=CIRCLE ( 'NONE', #76980, 0.5000000000000007772 ) ;
#66380=CARTESIAN_POINT ( 'NONE',  ( 197.4878715644970555, 25.93102243561465414, 12.00000000000000178 ) ) ;
#66388=CARTESIAN_POINT ( 'NONE',  ( 197.4836817735085219, 24.47698789593440694, 11.66666666666668384 ) ) ;
#66391=CARTESIAN_POINT ( 'NONE',  ( 197.4878715644970555, 25.93102243561465414, 12.00000000000000000 ) ) ;
#66392=DIRECTION ( 'NONE',  ( 0.000000000000000000, 1.000000000000000000, 0.000000000000000000 ) ) ;
#66405=CARTESIAN_POINT ( 'NONE',  ( 140.6539576904058606, 275.5000000000000568, 10.50000000000000000 ) ) ;
#66417=CARTESIAN_POINT ( 'NONE',  ( 199.9041579857632200, 299.4540172553377602, -5.820662028140222155 ) ) ;
#66418=EDGE_CURVE ( 'NONE', #7087, #15166, #322, .T. ) ;
#66421=CARTESIAN_POINT ( 'NONE',  ( 175.2296996224750103, 250.5000000000000568, 0.000000000000000000 ) ) ;
#66437=ORIENTED_EDGE ( 'NONE', *, *, #25761, .F. ) ;
#66440=EDGE_CURVE ( 'NONE', #36747, #17168, #51948, .T. ) ;
#66445=AXIS2_PLACEMENT_3D ( 'NONE', #78402, #41446, #63281 ) ;
#66449=EDGE_LOOP ( 'NONE', ( #91832, #58175, #73003, #17672 ) ) ;
#66460=ORIENTED_EDGE ( 'NONE', *, *, #9747, .F. ) ;
#66466=ADVANCED_FACE ( 'NONE', ( #35385 ), #41990, .T. ) ;
#66468=VERTEX_POINT ( 'NONE', #77533 ) ;
#66469=CARTESIAN_POINT ( 'NONE',  ( 157.4221907153413724, 15.99782226686522790, 9.062927103449265331 ) ) ;
#66484=EDGE_CURVE ( 'NONE', #54755, #55081, #35348, .T. ) ;
#66489=CARTESIAN_POINT ( 'NONE',  ( 209.9972545312790544, 27.55378999303205845, 10.00000000000000000 ) ) ;
#66495=CARTESIAN_POINT ( 'NONE',  ( 154.7659666677267580, 19.56018909072084000, 12.94946946941269594 ) ) ;
#66505=DIRECTION ( 'NONE',  ( 0.000000000000000000, -1.000000000000000000, 0.000000000000000000 ) ) ;
#66512=TOROIDAL_SURFACE ( 'NONE', #12084, 2.500000000000009770, 0.5000000000000000000 ) ;
#66514=ORIENTED_EDGE ( 'NONE', *, *, #52243, .F. ) ;
#66519=DIRECTION ( 'NONE',  ( -0.000000000000000000, -1.000000000000000000, -0.000000000000000000 ) ) ;
#66522=CARTESIAN_POINT ( 'NONE',  ( 208.0393982316568326, 37.47427918878999265, 12.00000000000000000 ) ) ;
#66535=EDGE_CURVE ( 'NONE', #74021, #93112, #61041, .T. ) ;
#66553=EDGE_CURVE ( 'NONE', #74598, #48115, #34828, .T. ) ;
#66558=DIRECTION ( 'NONE',  ( -0.000000000000000000, -1.000000000000000000, -0.000000000000000000 ) ) ;
#66575=AXIS2_PLACEMENT_3D ( 'NONE', #82349, #11315, #55349 ) ;
#66580=FACE_OUTER_BOUND ( 'NONE', #54616, .T. ) ;
#66586=VERTEX_POINT ( 'NONE', #70903 ) ;
#66611=EDGE_CURVE ( 'NONE', #21221, #59134, #34448, .T. ) ;
#66613=DIRECTION ( 'NONE',  ( 1.000000000000000000, 0.000000000000000000, 0.000000000000000000 ) ) ;
#66625=DIRECTION ( 'NONE',  ( 0.000000000000000000, 1.000000000000000000, 0.000000000000000000 ) ) ;
#66636=AXIS2_PLACEMENT_3D ( 'NONE', #90150, #24361, #25298 ) ;
#66640=CARTESIAN_POINT ( 'NONE',  ( 154.1415209985679269, 20.37991841447902175, 11.45812909362559040 ) ) ;
#66642=CARTESIAN_POINT ( 'NONE',  ( 169.7306087885279453, 276.0000000000000568, -24.89999999999999147 ) ) ;
#66643=VECTOR ( 'NONE', #40854, 1000.000000000000000 ) ;
#66652=ORIENTED_EDGE ( 'NONE', *, *, #2889, .F. ) ;
#66653=LINE ( 'NONE', #15520, #16885 ) ;
#66682=CARTESIAN_POINT ( 'NONE',  ( 197.8563597697584839, 42.27872732282708057, 12.00000000000000355 ) ) ;
#66684=EDGE_CURVE ( 'NONE', #4576, #47569, #77722, .T. ) ;
#66686=CARTESIAN_POINT ( 'NONE',  ( 175.2296996224750103, 133.0000000000000000, -24.00000000000001066 ) ) ;
#66695=DIRECTION ( 'NONE',  ( -0.000000000000000000, -1.000000000000000000, -0.000000000000000000 ) ) ;
#66699=ORIENTED_EDGE ( 'NONE', *, *, #84888, .T. ) ;
#66701=CARTESIAN_POINT ( 'NONE',  ( 193.5659903145831038, 250.0000000000000568, 16.24901362097127233 ) ) ;
#66712=AXIS2_PLACEMENT_3D ( 'NONE', #3395, #32284, #61191 ) ;
#66716=CARTESIAN_POINT ( 'NONE',  ( 197.2116943569230898, 214.9331615741067765, -12.42446933126075592 ) ) ;
#66724=CARTESIAN_POINT ( 'NONE',  ( 206.6165621753558526, 0.01303144969186966970, 7.291618491801075130 ) ) ;
#66728=DIRECTION ( 'NONE',  ( 0.000000000000000000, 0.000000000000000000, 1.000000000000000000 ) ) ;
#66737=ADVANCED_FACE ( 'NONE', ( #7419 ), #6636, .T. ) ;
#66741=DIRECTION ( 'NONE',  ( 0.000000000000000000, 0.000000000000000000, 1.000000000000000000 ) ) ;
#66752=LINE ( 'NONE', #65857, #65053 ) ;
#66755=DIRECTION ( 'NONE',  ( 0.000000000000000000, 0.000000000000000000, 1.000000000000000000 ) ) ;
#66767=DIRECTION ( 'NONE',  ( 0.000000000000000000, 0.000000000000000000, 1.000000000000000000 ) ) ;
#66771=CARTESIAN_POINT ( 'NONE',  ( 175.2296996224750103, 275.5000000000000568, 0.000000000000000000 ) ) ;
#66781=ORIENTED_EDGE ( 'NONE', *, *, #72094, .T. ) ;
#66788=ORIENTED_EDGE ( 'NONE', *, *, #11852, .F. ) ;
#66795=CARTESIAN_POINT ( 'NONE',  ( 209.4486294747436261, 36.74096400909239435, 13.09663628362915055 ) ) ;
#66806=ORIENTED_EDGE ( 'NONE', *, *, #69037, .T. ) ;
#66828=AXIS2_PLACEMENT_3D ( 'NONE', #87858, #37225, #9253 ) ;
#66836=ADVANCED_FACE ( 'NONE', ( #57175 ), #92654, .F. ) ;
#66837=FACE_OUTER_BOUND ( 'NONE', #41234, .T. ) ;
#66838=AXIS2_PLACEMENT_3D ( 'NONE', #41192, #3846, #48785 ) ;
#66840=CARTESIAN_POINT ( 'NONE',  ( 0.000000000000000000, 3.000000000000000000, -9.000000000000001776 ) ) ;
#66843=CARTESIAN_POINT ( 'NONE',  ( 199.8090428944973382, 41.61473866538664623, 10.14950798386179009 ) ) ;
#66869=CARTESIAN_POINT ( 'NONE',  ( 156.4892692376083971, 15.19211566834788485, 9.995848581180753811 ) ) ;
#66887=ORIENTED_EDGE ( 'NONE', *, *, #82549, .T. ) ;
#66900=VERTEX_POINT ( 'NONE', #65217 ) ;
#66901=VECTOR ( 'NONE', #74134, 1000.000000000000000 ) ;
#66904=CIRCLE ( 'NONE', #39629, 2.046895004029262832 ) ;
#66921=EDGE_LOOP ( 'NONE', ( #12390, #71838, #72939, #33722 ) ) ;
#66922=PLANE ( 'NONE',  #30675 ) ;
#66925=ORIENTED_EDGE ( 'NONE', *, *, #64104, .T. ) ;
#66941=CARTESIAN_POINT ( 'NONE',  ( 175.2296996224750103, 275.0000000000000568, 0.000000000000000000 ) ) ;
#66944=EDGE_CURVE ( 'NONE', #48610, #33225, #93586, .T. ) ;
#66949=CARTESIAN_POINT ( 'NONE',  ( 164.2231345125756263, 300.2961574867697436, -7.500000000000000000 ) ) ;
#66953=DIRECTION ( 'NONE',  ( -0.000000000000000000, 1.000000000000000000, -0.000000000000000000 ) ) ;
#66957=FACE_OUTER_BOUND ( 'NONE', #46030, .T. ) ;
#66971=CIRCLE ( 'NONE', #26132, 25.00000000000000000 ) ;
#66979=DIRECTION ( 'NONE',  ( 0.000000000000000000, -1.000000000000000000, 0.000000000000000000 ) ) ;
#66993=AXIS2_PLACEMENT_3D ( 'NONE', #3689, #2751, #76117 ) ;
#67010=CIRCLE ( 'NONE', #56411, 24.50000000000000355 ) ;
#67012=ORIENTED_EDGE ( 'NONE', *, *, #27047, .F. ) ;
#67034=ORIENTED_EDGE ( 'NONE', *, *, #27704, .T. ) ;
#67036=VECTOR ( 'NONE', #42120, 1000.000000000000000 ) ;
#67044=DIRECTION ( 'NONE',  ( 0.000000000000000000, 0.000000000000000000, 1.000000000000000000 ) ) ;
#67046=CIRCLE ( 'NONE', #91217, 5.568361562975243650 ) ;
#67050=ORIENTED_EDGE ( 'NONE', *, *, #4713, .T. ) ;
#67051=CARTESIAN_POINT ( 'NONE',  ( 196.4635112535681856, 24.42475431280786680, 11.30725198228063988 ) ) ;
#67068=DIRECTION ( 'NONE',  ( 0.000000000000000000, 0.000000000000000000, 1.000000000000000000 ) ) ;
#67070=CIRCLE ( 'NONE', #57970, 0.5000000000000004441 ) ;
#67079=DIRECTION ( 'NONE',  ( -0.3994899938748465162, 0.000000000000000000, -0.9167375550253601402 ) ) ;
#67083=ADVANCED_FACE ( 'NONE', ( #8799 ), #14997, .T. ) ;
#67085=LINE ( 'NONE', #8828, #53182 ) ;
#67088=DIRECTION ( 'NONE',  ( 0.000000000000000000, 1.000000000000000000, 0.000000000000000000 ) ) ;
#67112=CARTESIAN_POINT ( 'NONE',  ( 138.6539576904058606, 275.5000000000000568, -10.49999999999999822 ) ) ;
#67113=AXIS2_PLACEMENT_3D ( 'NONE', #43404, #72299, #42944 ) ;
#67130=CIRCLE ( 'NONE', #65672, 9.550761578869391144 ) ;
#67138=AXIS2_PLACEMENT_3D ( 'NONE', #10330, #26423, #82767 ) ;
#67142=ORIENTED_EDGE ( 'NONE', *, *, #24310, .T. ) ;
#67159=EDGE_CURVE ( 'NONE', #84959, #63082, #11128, .T. ) ;
#67161=CARTESIAN_POINT ( 'NONE',  ( 152.0128028882535887, 20.82798718771466540, 9.301361753755822193 ) ) ;
#67170=CARTESIAN_POINT ( 'NONE',  ( 207.5984058588019536, 35.65225752631543088, 15.03172026579641951 ) ) ;
#67174=ORIENTED_EDGE ( 'NONE', *, *, #47800, .T. ) ;
#67176=CARTESIAN_POINT ( 'NONE',  ( 198.8856906601489811, 17.32477107587094167, -10.54429824094598800 ) ) ;
#67186=TOROIDAL_SURFACE ( 'NONE', #91343, 4.499999999999993783, 0.5000000000000000000 ) ;
#67200=CARTESIAN_POINT ( 'NONE',  ( 208.4306832106271088, 0.04196010845015941959, 7.500000000000013323 ) ) ;
#67202=CIRCLE ( 'NONE', #26364, 4.499999999999990230 ) ;
#67212=VECTOR ( 'NONE', #90421, 1000.000000000000000 ) ;
#67219=TOROIDAL_SURFACE ( 'NONE', #32402, 1.000000000000000000, 0.5000000000000000000 ) ;
#67229=EDGE_CURVE ( 'NONE', #50020, #13665, #91277, .T. ) ;
#67233=ORIENTED_EDGE ( 'NONE', *, *, #78401, .F. ) ;
#67237=DIRECTION ( 'NONE',  ( 0.000000000000000000, 1.000000000000000000, 0.000000000000000000 ) ) ;
#67245=ORIENTED_EDGE ( 'NONE', *, *, #86598, .F. ) ;
#67252=CARTESIAN_POINT ( 'NONE',  ( 189.9243309297870610, 250.0000000000000568, 24.72542485937348644 ) ) ;
#67260=ORIENTED_EDGE ( 'NONE', *, *, #11852, .T. ) ;
#67264=CIRCLE ( 'NONE', #46083, 2.999999999999993783 ) ;
#67270=EDGE_LOOP ( 'NONE', ( #74410, #66372, #376, #33343 ) ) ;
#67277=DIRECTION ( 'NONE',  ( -0.000000000000000000, -1.000000000000000000, -0.000000000000000000 ) ) ;
#67289=ORIENTED_EDGE ( 'NONE', *, *, #9862, .T. ) ;
#67290=CYLINDRICAL_SURFACE ( 'NONE', #39766, 24.00000000000001066 ) ;
#67300=CARTESIAN_POINT ( 'NONE',  ( 207.7761861081325208, 35.69891260691532153, 14.41714557868260371 ) ) ;
#67319=LINE ( 'NONE', #52157, #60769 ) ;
#67324=CARTESIAN_POINT ( 'NONE',  ( 200.4644824113734387, 214.9910457053126720, -2.942835885954282471 ) ) ;
#67325=FACE_OUTER_BOUND ( 'NONE', #74064, .T. ) ;
#67333=ADVANCED_FACE ( 'NONE', ( #65686 ), #62682, .T. ) ;
#67336=CARTESIAN_POINT ( 'NONE',  ( 199.4392256788250677, 65.82574266882504332, 7.741079165001067963 ) ) ;
#67344=AXIS2_PLACEMENT_3D ( 'NONE', #8443, #37322, #66230 ) ;
#67352=CARTESIAN_POINT ( 'NONE',  ( 164.8901442405950206, 2.982772324107380690, 9.000000000000000000 ) ) ;
#67353=CYLINDRICAL_SURFACE ( 'NONE', #14820, 11.60392986742922439 ) ;
#67369=VERTEX_POINT ( 'NONE', #81239 ) ;
#67372=ORIENTED_EDGE ( 'NONE', *, *, #86489, .T. ) ;
#67382=VERTEX_POINT ( 'NONE', #8348 ) ;
#67389=EDGE_CURVE ( 'NONE', #10282, #80534, #45236, .T. ) ;
#67393=EDGE_CURVE ( 'NONE', #23662, #13726, #55122, .T. ) ;
#67395=ORIENTED_EDGE ( 'NONE', *, *, #89572, .F. ) ;
#67402=VERTEX_POINT ( 'NONE', #1251 ) ;
#67403=CARTESIAN_POINT ( 'NONE',  ( 159.2635086430408080, 16.43186977800937498, 9.166206881811428175 ) ) ;
#67407=ORIENTED_EDGE ( 'NONE', *, *, #27704, .F. ) ;
#67421=CIRCLE ( 'NONE', #6927, 0.4999999999999923395 ) ;
#67424=PLANE ( 'NONE',  #91118 ) ;
#67429=ADVANCED_FACE ( 'NONE', ( #80314 ), #50974, .F. ) ;
#67430=DIRECTION ( 'NONE',  ( -0.7453559924999194619, 0.000000000000000000, -0.6666666666666782870 ) ) ;
#67431=CARTESIAN_POINT ( 'NONE',  ( 206.9189553108847406, 30.70889394204682432, 14.49999999999999822 ) ) ;
#67434=CARTESIAN_POINT ( 'NONE',  ( 195.7161433444922807, 19.55326545191306309, 12.92152971952034513 ) ) ;
#67436=CARTESIAN_POINT ( 'NONE',  ( 155.6265766802774806, 17.98195150565546996, -10.85854113850068892 ) ) ;
#67438=DIRECTION ( 'NONE',  ( 0.000000000000000000, 0.000000000000000000, -1.000000000000000000 ) ) ;
#67474=CARTESIAN_POINT ( 'NONE',  ( 199.7589824058529473, 41.15052235409930859, 10.49999999999999822 ) ) ;
#67486=ORIENTED_EDGE ( 'NONE', *, *, #64191, .T. ) ;
#67488=ORIENTED_EDGE ( 'NONE', *, *, #66150, .F. ) ;
#67504=VERTEX_POINT ( 'NONE', #38618 ) ;
#67511=CARTESIAN_POINT ( 'NONE',  ( 197.6806146935310551, 68.83995197827617574, -9.477423483297931384 ) ) ;
#67517=CARTESIAN_POINT ( 'NONE',  ( 156.4851178187871312, 0.000000000000000000, 7.000000000000000000 ) ) ;
#67536=DIRECTION ( 'NONE',  ( 0.000000000000000000, 1.000000000000000000, 0.000000000000000000 ) ) ;
#67546=CARTESIAN_POINT ( 'NONE',  ( 164.2231345125756263, 275.0000000000000568, -7.500000000000000000 ) ) ;
#67551=CARTESIAN_POINT ( 'NONE',  ( 164.2231345125756263, 300.2961574867697436, -4.888549259831427740 ) ) ;
#67554=DIRECTION ( 'NONE',  ( 0.2916739763039189470, 0.000000000000000000, 0.9565177946839572565 ) ) ;
#67561=CARTESIAN_POINT ( 'NONE',  ( 193.9153122143737562, 214.9910457053126720, 17.21343741151142481 ) ) ;
#67564=DIRECTION ( 'NONE',  ( 0.000000000000000000, 1.000000000000000000, 0.000000000000000000 ) ) ;
#67573=EDGE_CURVE ( 'NONE', #17873, #5311, #45927, .T. ) ;
#67581=CARTESIAN_POINT ( 'NONE',  ( 201.2104617360081704, 41.21457449016151031, 10.00000000000000000 ) ) ;
#67593=AXIS2_PLACEMENT_3D ( 'NONE', #26482, #32182, #68641 ) ;
#67596=ADVANCED_FACE ( 'NONE', ( #32466 ), #58069, .F. ) ;
#67602=DIRECTION ( 'NONE',  ( 0.000000000000000000, 0.000000000000000000, 1.000000000000000000 ) ) ;
#67632=FACE_OUTER_BOUND ( 'NONE', #70547, .T. ) ;
#67636=ORIENTED_EDGE ( 'NONE', *, *, #18958, .T. ) ;
#67637=ORIENTED_EDGE ( 'NONE', *, *, #31148, .T. ) ;
#67638=CARTESIAN_POINT ( 'NONE',  ( 195.5762488419090346, 41.38929653454901114, 14.52727654096534060 ) ) ;
#67653=DIRECTION ( 'NONE',  ( -0.000000000000000000, -1.000000000000000000, -0.000000000000000000 ) ) ;
#67667=CARTESIAN_POINT ( 'NONE',  ( 160.5350683151633291, 275.0000000000000568, 20.22542485937379908 ) ) ;
#67677=DIRECTION ( 'NONE',  ( -0.9953184226294286008, 0.000000000000000000, 0.09665007798479081924 ) ) ;
#67687=ORIENTED_EDGE ( 'NONE', *, *, #44800, .F. ) ;
#67688=DIRECTION ( 'NONE',  ( 0.000000000000000000, 1.000000000000000000, 0.000000000000000000 ) ) ;
#67691=LINE ( 'NONE', #24585, #20167 ) ;
#67702=DIRECTION ( 'NONE',  ( 0.9531768234071980039, -0.3024135303179465994, -0.000000000000000000 ) ) ;
#67704=CARTESIAN_POINT ( 'NONE',  ( 196.1388477366602956, 72.64613238536348661, 11.79151705418648177 ) ) ;
#67705=EDGE_CURVE ( 'NONE', #70776, #19395, #87789, .T. ) ;
#67721=EDGE_CURVE ( 'NONE', #83547, #67504, #17788, .T. ) ;
#67723=EDGE_CURVE ( 'NONE', #27549, #56772, #82234, .T. ) ;
#67727=AXIS2_PLACEMENT_3D ( 'NONE', #34835, #77936, #40494 ) ;
#67733=FACE_OUTER_BOUND ( 'NONE', #36371, .T. ) ;
#67744=EDGE_LOOP ( 'NONE', ( #14982, #22322, #32694, #31519, #64522, #64836, #24114 ) ) ;
#67745=CARTESIAN_POINT ( 'NONE',  ( 195.4349574838196020, 27.23211070204046180, 14.00000000000008882 ) ) ;
#67754=CARTESIAN_POINT ( 'NONE',  ( 198.6003787446688591, 25.18134682881806796, 11.03083405179678778 ) ) ;
#67764=CARTESIAN_POINT ( 'NONE',  ( 159.4851178187871312, 15.00000000000000000, 10.00000000000000000 ) ) ;
#67766=CARTESIAN_POINT ( 'NONE',  ( 194.3836820389603304, 26.49645583160156193, 14.46137890893106892 ) ) ;
#67773=CARTESIAN_POINT ( 'NONE',  ( 155.0231696494687981, 19.71747416577793643, 13.29925684039281286 ) ) ;
#67775=FACE_BOUND ( 'NONE', #34640, .T. ) ;
#67778=CARTESIAN_POINT ( 'NONE',  ( 175.2296996224750103, 154.6894116713782807, -24.16304133878946558 ) ) ;
#67790=ORIENTED_EDGE ( 'NONE', *, *, #9225, .F. ) ;
#67806=CARTESIAN_POINT ( 'NONE',  ( 212.7238915819278589, 32.98517505407394168, 12.09245862095555601 ) ) ;
#67809=DIRECTION ( 'NONE',  ( -0.000000000000000000, -0.000000000000000000, 1.000000000000000000 ) ) ;
#67824=ORIENTED_EDGE ( 'NONE', *, *, #66944, .F. ) ;
#67832=CARTESIAN_POINT ( 'NONE',  ( 196.7071296363290855, 19.50333209967908132, -12.79999999999999361 ) ) ;
#67837=ORIENTED_EDGE ( 'NONE', *, *, #75080, .T. ) ;
#67848=ORIENTED_EDGE ( 'NONE', *, *, #84552, .F. ) ;
#67853=EDGE_CURVE ( 'NONE', #59112, #50020, #32471, .T. ) ;
#67864=VECTOR ( 'NONE', #36212, 1000.000000000000000 ) ;
#67879=FACE_OUTER_BOUND ( 'NONE', #13027, .T. ) ;
#67885=DIRECTION ( 'NONE',  ( 0.9531768234071978929, -0.3024135303179465439, 0.000000000000000000 ) ) ;
#67886=DIRECTION ( 'NONE',  ( 0.3262578496237564796, 0.000000000000000000, 0.9452808130703185263 ) ) ;
#67889=DIRECTION ( 'NONE',  ( 0.000000000000000000, 1.000000000000000000, 0.000000000000000000 ) ) ;
#67891=CARTESIAN_POINT ( 'NONE',  ( 156.1688672180497690, 17.06233518523552917, -10.31625060074404487 ) ) ;
#67910=EDGE_CURVE ( 'NONE', #75307, #26750, #48993, .T. ) ;
#67912=EDGE_CURVE ( 'NONE', #68073, #22603, #76226, .T. ) ;
#67929=AXIS2_PLACEMENT_3D ( 'NONE', #86745, #21429, #35652 ) ;
#67944=EDGE_LOOP ( 'NONE', ( #62761, #6231, #78786 ) ) ;
#67946=EDGE_LOOP ( 'NONE', ( #5888, #35959, #50605, #86560 ) ) ;
#67960=VERTEX_POINT ( 'NONE', #47102 ) ;
#67965=ORIENTED_EDGE ( 'NONE', *, *, #29049, .T. ) ;
#67971=FACE_OUTER_BOUND ( 'NONE', #27218, .T. ) ;
#67975=EDGE_CURVE ( 'NONE', #29329, #56700, #53580, .T. ) ;
#67978=CARTESIAN_POINT ( 'NONE',  ( 208.6208076322478746, 32.98517505407394168, 12.09245862095555601 ) ) ;
#67990=CIRCLE ( 'NONE', #48305, 4.025000000000000355 ) ;
#68000=CARTESIAN_POINT ( 'NONE',  ( 209.8744251295252354, 28.03846817292548366, 10.50000000000000000 ) ) ;
#68008=CARTESIAN_POINT ( 'NONE',  ( 179.7289557593406357, 276.0000000000000568, -24.91818181818184641 ) ) ;
#68016=CARTESIAN_POINT ( 'NONE',  ( 160.5350683151633291, 215.0000000000000568, 20.22542485937379908 ) ) ;
#68018=EDGE_CURVE ( 'NONE', #16726, #11326, #39144, .T. ) ;
#68020=ADVANCED_FACE ( 'NONE', ( #18721, #47584 ), #39065, .F. ) ;
#68021=CARTESIAN_POINT ( 'NONE',  ( 219.8344101925596021, 35.72494958537217968, -7.000000000000000000 ) ) ;
#68034=EDGE_LOOP ( 'NONE', ( #48854, #87851, #11703, #9827, #74971 ) ) ;
#68048=CARTESIAN_POINT ( 'NONE',  ( 140.6539576904058606, 275.0000000000000568, -12.50000000000000000 ) ) ;
#68058=CARTESIAN_POINT ( 'NONE',  ( 184.3556211049944409, 2.982772324107381579, 9.000000000000000000 ) ) ;
#68061=VECTOR ( 'NONE', #20806, 1000.000000000000000 ) ;
#68064=VERTEX_POINT ( 'NONE', #3104 ) ;
#68073=VERTEX_POINT ( 'NONE', #39522 ) ;
#68078=DIRECTION ( 'NONE',  ( 0.000000000000000000, 0.000000000000000000, 1.000000000000000000 ) ) ;
#68081=CARTESIAN_POINT ( 'NONE',  ( 153.3309649087729838, 129.0860594806759423, 12.69538652463440442 ) ) ;
#68090=CARTESIAN_POINT ( 'NONE',  ( 185.2519943799831879, 3.000000000000000444, -9.000000000000001776 ) ) ;
#68093=ORIENTED_EDGE ( 'NONE', *, *, #5615, .T. ) ;
#68094=ADVANCED_FACE ( 'NONE', ( #12079 ), #67186, .T. ) ;
#68095=FACE_OUTER_BOUND ( 'NONE', #36012, .T. ) ;
#68109=DIRECTION ( 'NONE',  ( 0.000000000000000000, 0.000000000000000000, 1.000000000000000000 ) ) ;
#68110=CARTESIAN_POINT ( 'NONE',  ( 154.4590814691992193, 20.78850955393007638, -13.92316269559726472 ) ) ;
#68118=( NAMED_UNIT ( * ) SI_UNIT ( $, .STERADIAN. ) SOLID_ANGLE_UNIT ( ) );
#68122=EDGE_CURVE ( 'NONE', #30954, #93112, #24409, .T. ) ;
#68123=CYLINDRICAL_SURFACE ( 'NONE', #74754, 2.999999999999997335 ) ;
#68125=AXIS2_PLACEMENT_3D ( 'NONE', #86529, #85615, #62938 ) ;
#68126=CARTESIAN_POINT ( 'NONE',  ( 195.8725848201698341, 20.33787691583836121, 12.24547402278110475 ) ) ;
#68131=AXIS2_PLACEMENT_3D ( 'NONE', #12004, #62702, #11538 ) ;
#68134=EDGE_CURVE ( 'NONE', #45831, #63777, #57072, .T. ) ;
#68135=DIRECTION ( 'NONE',  ( 0.000000000000000000, 0.000000000000000000, 1.000000000000000000 ) ) ;
#68145=EDGE_CURVE ( 'NONE', #43024, #87978, #6702, .T. ) ;
#68149=ORIENTED_EDGE ( 'NONE', *, *, #2808, .F. ) ;
#68150=CARTESIAN_POINT ( 'NONE',  ( 197.1933712184921603, 24.89666632552609826, 12.64285714285712992 ) ) ;
#68152=CARTESIAN_POINT ( 'NONE',  ( 175.2296996224750103, 249.5000000000000568, 0.000000000000000000 ) ) ;
#68164=CARTESIAN_POINT ( 'NONE',  ( 175.2296996224749250, 275.0000000000000568, -24.99999999999999289 ) ) ;
#68166=CARTESIAN_POINT ( 'NONE',  ( 156.8306017167579114, 275.6568570078858329, 16.89650703334504911 ) ) ;
#68169=CARTESIAN_POINT ( 'NONE',  ( 154.1407330040854333, 128.0000000000000568, -13.42592592592592737 ) ) ;
#68179=ORIENTED_EDGE ( 'NONE', *, *, #34788, .T. ) ;
#68189=ORIENTED_EDGE ( 'NONE', *, *, #38083, .F. ) ;
#68190=ORIENTED_EDGE ( 'NONE', *, *, #40288, .T. ) ;
#68191=DIRECTION ( 'NONE',  ( 0.000000000000000000, 0.000000000000000000, 1.000000000000000000 ) ) ;
#68192=VECTOR ( 'NONE', #72592, 1000.000000000000000 ) ;
#68197=CARTESIAN_POINT ( 'NONE',  ( 151.7489156927950376, 20.88249531811356263, -8.613363710899797354 ) ) ;
#68209=ORIENTED_EDGE ( 'NONE', *, *, #15663, .T. ) ;
#68210=CARTESIAN_POINT ( 'NONE',  ( 175.2296996224750103, 249.5000000000000568, 25.00000000000000355 ) ) ;
#68218=CARTESIAN_POINT ( 'NONE',  ( 201.0876323342543515, 25.81167821795958162, 10.49999999999999822 ) ) ;
#68231=CARTESIAN_POINT ( 'NONE',  ( 196.0143093133015384, 24.42324672360810212, 11.99999999999998934 ) ) ;
#68235=B_SPLINE_CURVE_WITH_KNOTS ( 'NONE', 3,
 ( #90674, #39092, #40485, #19215, #53797, #47129, #46667, #91150 ),
 .UNSPECIFIED., .F., .F.,
 ( 4, 2, 2, 4 ),
 ( 0.000000000000000000, 0.004220890787215657823, 0.006331336180823474158, 0.008441781574431289625 ),
 .UNSPECIFIED. ) ;
#68239=CARTESIAN_POINT ( 'NONE',  ( 154.1407330040854333, 128.0000000000000568, -13.42592592592592737 ) ) ;
#68243=DIRECTION ( 'NONE',  ( 0.000000000000000000, 1.000000000000000000, 0.000000000000000000 ) ) ;
#68244=CARTESIAN_POINT ( 'NONE',  ( 219.8344101925596021, 36.73669859915801794, 10.00000000000000000 ) ) ;
#68257=VECTOR ( 'NONE', #79481, 1000.000000000000000 ) ;
#68258=EDGE_CURVE ( 'NONE', #44986, #74736, #2156, .T. ) ;
#68270=DIRECTION ( 'NONE',  ( 0.000000000000000000, 0.000000000000000000, 1.000000000000000000 ) ) ;
#68288=ORIENTED_EDGE ( 'NONE', *, *, #26658, .T. ) ;
#68290=VERTEX_POINT ( 'NONE', #77904 ) ;
#68296=CARTESIAN_POINT ( 'NONE',  ( 140.6539576904058606, 250.5000000000000568, 12.50000000000000000 ) ) ;
#68312=VERTEX_POINT ( 'NONE', #7320 ) ;
#68320=CARTESIAN_POINT ( 'NONE',  ( 157.1544330182169631, 16.98551211945807893, 7.440913067426849992 ) ) ;
#68325=VERTEX_POINT ( 'NONE', #41884 ) ;
#68338=CARTESIAN_POINT ( 'NONE',  ( 193.9402003287077605, 214.5000000000000568, 16.58062614384823874 ) ) ;
#68342=DIRECTION ( 'NONE',  ( -0.000000000000000000, -1.000000000000000000, -0.000000000000000000 ) ) ;
#68345=EDGE_CURVE ( 'NONE', #92829, #33827, #70795, .T. ) ;
#68348=CYLINDRICAL_SURFACE ( 'NONE', #50412, 1.500000000000001332 ) ;
#68353=CARTESIAN_POINT ( 'NONE',  ( 156.4851178187871312, 15.00000000000000178, -10.00000000000000000 ) ) ;
#68366=ADVANCED_FACE ( 'NONE', ( #27707 ), #80674, .T. ) ;
#68369=ORIENTED_EDGE ( 'NONE', *, *, #67853, .T. ) ;
#68372=DIRECTION ( 'NONE',  ( -0.000000000000000000, -1.000000000000000000, -0.000000000000000000 ) ) ;
#68374=ORIENTED_EDGE ( 'NONE', *, *, #8991, .F. ) ;
#68389=EDGE_CURVE ( 'NONE', #4490, #63422, #11200, .T. ) ;
#68392=AXIS2_PLACEMENT_3D ( 'NONE', #86841, #36655, #690 ) ;
#68399=AXIS2_PLACEMENT_3D ( 'NONE', #41797, #84879, #6779 ) ;
#68404=CIRCLE ( 'NONE', #59280, 24.00000000000000000 ) ;
#68408=EDGE_LOOP ( 'NONE', ( #9462, #64510, #82246, #53410 ) ) ;
#68431=ORIENTED_EDGE ( 'NONE', *, *, #21626, .F. ) ;
#68443=CARTESIAN_POINT ( 'NONE',  ( 197.2116943569230898, 214.9331615741067765, -12.42446933126075592 ) ) ;
#68452=AXIS2_PLACEMENT_3D ( 'NONE', #7782, #50411, #78832 ) ;
#68461=AXIS2_PLACEMENT_3D ( 'NONE', #40571, #34443, #90757 ) ;
#68468=DIRECTION ( 'NONE',  ( 0.000000000000000000, -1.000000000000000000, 0.000000000000000000 ) ) ;
#68489=CIRCLE ( 'NONE', #21588, 7.500000000000013323 ) ;
#68498=ADVANCED_FACE ( 'NONE', ( #65117 ), #22451, .T. ) ;
#68504=DIRECTION ( 'NONE',  ( 1.000000000000000000, 0.000000000000000000, 1.224646799147353207E-16 ) ) ;
#68516=CARTESIAN_POINT ( 'NONE',  ( 208.6208076322478746, 32.98517505407394168, 14.49999999999999822 ) ) ;
#68525=AXIS2_PLACEMENT_3D ( 'NONE', #22457, #74508, #67430 ) ;
#68527=DIRECTION ( 'NONE',  ( -0.000000000000000000, -0.000000000000000000, 1.000000000000000000 ) ) ;
#68528=CARTESIAN_POINT ( 'NONE',  ( 154.7659666677360235, 19.56018909072649237, -12.94946946942526189 ) ) ;
#68532=ORIENTED_EDGE ( 'NONE', *, *, #57514, .T. ) ;
#68542=ORIENTED_EDGE ( 'NONE', *, *, #18738, .F. ) ;
#68547=DIRECTION ( 'NONE',  ( 0.000000000000000000, 0.000000000000000000, -1.000000000000000000 ) ) ;
#68549=CIRCLE ( 'NONE', #3519, 0.5000000000000004441 ) ;
#68551=B_SPLINE_CURVE_WITH_KNOTS ( 'NONE', 3,
 ( #49592, #21179, #93144, #6986, #58119, #43419, #42477, #50529, #57642, #92201, #28299, #7435, #86487, #56245 ),
 .UNSPECIFIED., .F., .F.,
 ( 4, 2, 2, 2, 2, 2, 4 ),
 ( 0.000000000000000000, 0.0003894434397089267179, 0.0007788868794178534357, 0.001168330319126780316, 0.001557773758835706871, 0.002336660638253565837, 0.003115547517671425019 ),
 .UNSPECIFIED. ) ;
#68562=ADVANCED_FACE ( 'NONE', ( #23393 ), #15741, .T. ) ;
#68563=CARTESIAN_POINT ( 'NONE',  ( 194.6714370800177676, 41.21621202809333084, 14.07240042052004725 ) ) ;
#68565=EDGE_LOOP ( 'NONE', ( #53360, #72419, #75288, #18680, #38135, #37340 ) ) ;
#68566=CARTESIAN_POINT ( 'NONE',  ( 197.3380612925966489, 18.22700036951276914, 11.15593255764728831 ) ) ;
#68577=AXIS2_PLACEMENT_3D ( 'NONE', #42941, #14076, #58559 ) ;
#68592=AXIS2_PLACEMENT_3D ( 'NONE', #51439, #80327, #67068 ) ;
#68594=DIRECTION ( 'NONE',  ( 0.6056179655966479336, -0.7957555401921982963, 0.000000000000000000 ) ) ;
#68606=FACE_OUTER_BOUND ( 'NONE', #92870, .T. ) ;
#68611=AXIS2_PLACEMENT_3D ( 'NONE', #50772, #43654, #65936 ) ;
#68613=VECTOR ( 'NONE', #53372, 1000.000000000000000 ) ;
#68618=DIRECTION ( 'NONE',  ( 1.000000000000000000, 0.000000000000000000, 0.000000000000000000 ) ) ;
#68621=CARTESIAN_POINT ( 'NONE',  ( 216.5288609127277084, 293.9636489450776935, -40.00000000000000711 ) ) ;
#68630=ORIENTED_EDGE ( 'NONE', *, *, #39673, .T. ) ;
#68637=ORIENTED_EDGE ( 'NONE', *, *, #37224, .F. ) ;
#68641=DIRECTION ( 'NONE',  ( 1.000000000000000000, 0.000000000000000000, 0.000000000000000000 ) ) ;
#68658=ORIENTED_EDGE ( 'NONE', *, *, #15525, .F. ) ;
#68661=CARTESIAN_POINT ( 'NONE',  ( 169.8384340989974817, 275.5000000000000568, -24.41176470588234437 ) ) ;
#68666=CARTESIAN_POINT ( 'NONE',  ( 151.0524635986548674, 20.99320456764979070, -6.527652849435627402 ) ) ;
#68670=EDGE_CURVE ( 'NONE', #22603, #39182, #30033, .T. ) ;
#68680=CARTESIAN_POINT ( 'NONE',  ( 201.2509219215139922, 65.09645894978945080, 2.617322427804800622 ) ) ;
#68684=CIRCLE ( 'NONE', #38444, 0.4999999999999926170 ) ;
#68691=CIRCLE ( 'NONE', #44477, 24.50000000000000355 ) ;
#68697=TOROIDAL_SURFACE ( 'NONE', #27893, 1.000000000000000000, 0.5000000000000000000 ) ;
#68703=CARTESIAN_POINT ( 'NONE',  ( 186.2362647323748206, 276.0000000000000568, 22.80382896336985965 ) ) ;
#68712=CARTESIAN_POINT ( 'NONE',  ( 153.3309649087729838, 129.0860594806759423, -12.69538652463440442 ) ) ;
#68714=CARTESIAN_POINT ( 'NONE',  ( 186.6539576904058890, 293.9636489450775230, 11.60392986742922439 ) ) ;
#68717=CARTESIAN_POINT ( 'NONE',  ( 195.4781563537916327, 39.36132622696000283, 15.49999999999999645 ) ) ;
#68727=ORIENTED_EDGE ( 'NONE', *, *, #50389, .T. ) ;
#68728=DIRECTION ( 'NONE',  ( 1.233581138472395244E-14, 0.000000000000000000, 1.000000000000000000 ) ) ;
#68731=DIRECTION ( 'NONE',  ( -0.9693563597868444237, -0.2456588035076248677, 4.923761215728623624E-16 ) ) ;
#68736=( BOUNDED_CURVE ( )  B_SPLINE_CURVE ( 3, ( #17668, #9611, #46521, #75422 ),
 .UNSPECIFIED., .F., .F. ) 
 B_SPLINE_CURVE_WITH_KNOTS ( ( 4, 4 ),
 ( 4.712388980384689674, 6.283185307179586232 ),
 .UNSPECIFIED. ) 
 CURVE ( )  GEOMETRIC_REPRESENTATION_ITEM ( )  RATIONAL_B_SPLINE_CURVE ( ( 1.000000000000000000, 0.8047378541243649375, 0.8047378541243649375, 1.000000000000000000 ) ) 
 REPRESENTATION_ITEM ( '' )  );
#68742=( BOUNDED_CURVE ( )  B_SPLINE_CURVE ( 3, ( #69797, #91066, #56555, #70746 ),
 .UNSPECIFIED., .F., .F. ) 
 B_SPLINE_CURVE_WITH_KNOTS ( ( 4, 4 ),
 ( 1.570796326794894560, 2.004620063563923527 ),
 .UNSPECIFIED. ) 
 CURVE ( )  GEOMETRIC_REPRESENTATION_ITEM ( )  RATIONAL_B_SPLINE_CURVE ( ( 1.000000000000000000, 0.9843778111405746545, 0.9843778111405746545, 1.000000000000000000 ) ) 
 REPRESENTATION_ITEM ( '' )  );
#68745=CARTESIAN_POINT ( 'NONE',  ( 185.2519943799831879, 3.000000000000000444, -9.000000000000001776 ) ) ;
#68763=ORIENTED_EDGE ( 'NONE', *, *, #26148, .T. ) ;
#68792=ORIENTED_EDGE ( 'NONE', *, *, #22499, .T. ) ;
#68793=DIRECTION ( 'NONE',  ( 0.000000000000000000, 0.000000000000000000, 1.000000000000000000 ) ) ;
#68796=EDGE_CURVE ( 'NONE', #24735, #48324, #75398, .T. ) ;
#68799=ORIENTED_EDGE ( 'NONE', *, *, #49105, .F. ) ;
#68806=DIRECTION ( 'NONE',  ( 0.000000000000000000, 0.000000000000000000, 1.000000000000000000 ) ) ;
#68817=CARTESIAN_POINT ( 'NONE',  ( 199.6150009768959990, 275.5000000000000568, -2.367926910627516257 ) ) ;
#68819=AXIS2_PLACEMENT_3D ( 'NONE', #92229, #25962, #71419 ) ;
#68823=CARTESIAN_POINT ( 'NONE',  ( 186.6539576904058890, 276.0000000000000568, -11.60392986742922439 ) ) ;
#68824=CARTESIAN_POINT ( 'NONE',  ( 195.5396684847816573, 20.94006894122355433, 14.59130073475925116 ) ) ;
#68830=CARTESIAN_POINT ( 'NONE',  ( 209.2651480440030980, 38.13450996287912886, 14.02415587114431617 ) ) ;
#68832=CIRCLE ( 'NONE', #71895, 1.999999999999996003 ) ;
#68833=CARTESIAN_POINT ( 'NONE',  ( 156.1711712139736505, 21.00000000000000000, 14.59590564729795226 ) ) ;
#68836=CARTESIAN_POINT ( 'NONE',  ( 158.5846220834698670, 17.78059845260474248, -9.675371801486436496 ) ) ;
#68845=VERTEX_POINT ( 'NONE', #66489 ) ;
#68879=ORIENTED_EDGE ( 'NONE', *, *, #11367, .F. ) ;
#68882=ORIENTED_EDGE ( 'NONE', *, *, #18976, .T. ) ;
#68887=ADVANCED_FACE ( 'NONE', ( #8698 ), #45136, .F. ) ;
#68899=EDGE_LOOP ( 'NONE', ( #86134, #13344, #48209, #21718 ) ) ;
#68901=CIRCLE ( 'NONE', #40135, 5.568361562975243650 ) ;
#68906=EDGE_LOOP ( 'NONE', ( #26942, #44661 ) ) ;
#68909=ORIENTED_EDGE ( 'NONE', *, *, #86488, .F. ) ;
#68934=CARTESIAN_POINT ( 'NONE',  ( 184.7149167944524493, 8.542400036368780647, 10.00000000000000178 ) ) ;
#68942=CARTESIAN_POINT ( 'NONE',  ( 195.5424455875674425, 40.24675177650068036, 14.87863167422141153 ) ) ;
#68948=CARTESIAN_POINT ( 'NONE',  ( 183.0442525570908288, 264.6571197653884155, -7.500000000000000000 ) ) ;
#68978=CARTESIAN_POINT ( 'NONE',  ( 200.6103193995254230, 249.5000000000000568, -2.464576988612307229 ) ) ;
#68989=VERTEX_POINT ( 'NONE', #59859 ) ;
#68999=CARTESIAN_POINT ( 'NONE',  ( 196.4324178900849347, 72.07371985372441259, 11.29105239310641018 ) ) ;
#69000=PLANE ( 'NONE',  #31188 ) ;
#69004=VERTEX_POINT ( 'NONE', #696 ) ;
#69018=DIRECTION ( 'NONE',  ( -0.01818181818181330636, 0.000000000000000000, 0.9998346970812744816 ) ) ;
#69020=FACE_OUTER_BOUND ( 'NONE', #13957, .T. ) ;
#69029=CARTESIAN_POINT ( 'NONE',  ( 194.9193168125297575, 41.63678119477545181, 13.72372309788986300 ) ) ;
#69032=ORIENTED_EDGE ( 'NONE', *, *, #55137, .T. ) ;
#69033=ORIENTED_EDGE ( 'NONE', *, *, #73101, .T. ) ;
#69034=CARTESIAN_POINT ( 'NONE',  ( 197.0984808611917458, 19.93437704977205982, 12.12215979493358908 ) ) ;
#69037=EDGE_CURVE ( 'NONE', #84462, #85293, #18782, .T. ) ;
#69062=CARTESIAN_POINT ( 'NONE',  ( 209.7513585654922679, 305.7026273589066818, 13.99999999999999112 ) ) ;
#69064=CARTESIAN_POINT ( 'NONE',  ( 160.5350683151633291, 275.5000000000000568, 20.22542485937379908 ) ) ;
#69071=DIRECTION ( 'NONE',  ( 0.000000000000000000, -0.000000000000000000, 1.000000000000000000 ) ) ;
#69082=ORIENTED_EDGE ( 'NONE', *, *, #41751, .T. ) ;
#69085=CARTESIAN_POINT ( 'NONE',  ( 208.4306832106271088, 0.04196010845015910040, -7.500000000000013323 ) ) ;
#69090=EDGE_CURVE ( 'NONE', #17873, #59473, #71733, .T. ) ;
#69103=VERTEX_POINT ( 'NONE', #31888 ) ;
#69107=CARTESIAN_POINT ( 'NONE',  ( 197.2964169323986425, 25.88250311104176049, 12.12231587770837393 ) ) ;
#69108=CARTESIAN_POINT ( 'NONE',  ( 195.6164516548605548, 25.75475877429676785, 14.47166412665907842 ) ) ;
#69125=ORIENTED_EDGE ( 'NONE', *, *, #38392, .T. ) ;
#69126=CYLINDRICAL_SURFACE ( 'NONE', #57473, 0.5000000000000004441 ) ;
#69131=CARTESIAN_POINT ( 'NONE',  ( 199.5806965732583933, 26.46139589673911985, 10.63455718553152352 ) ) ;
#69141=VERTEX_POINT ( 'NONE', #70577 ) ;
#69142=DIRECTION ( 'NONE',  ( 1.000000000000000000, -0.000000000000000000, 0.000000000000000000 ) ) ;
#69150=DIRECTION ( 'NONE',  ( -0.000000000000000000, -1.000000000000000000, -0.000000000000000000 ) ) ;
#69163=CYLINDRICAL_SURFACE ( 'NONE', #45939, 5.999999999999998224 ) ;
#69165=DIRECTION ( 'NONE',  ( -0.9531768234073174639, 0.3024135303175699563, -3.864692125754213305E-13 ) ) ;
#69175=DIRECTION ( 'NONE',  ( -0.000000000000000000, -1.000000000000000000, -0.000000000000000000 ) ) ;
#69177=CARTESIAN_POINT ( 'NONE',  ( 157.4851178187871312, 17.34719063663031946, 6.999999999999999112 ) ) ;
#69178=CARTESIAN_POINT ( 'NONE',  ( 175.2296996224750103, 215.0000000000000568, 0.000000000000000000 ) ) ;
#69189=DIRECTION ( 'NONE',  ( -0.000000000000000000, -0.000000000000000000, -1.000000000000000000 ) ) ;
#69192=DIRECTION ( 'NONE',  ( 0.000000000000000000, 1.000000000000000000, 0.000000000000000000 ) ) ;
#69195=ADVANCED_FACE ( 'NONE', ( #39425 ), #3468, .T. ) ;
#69204=FACE_OUTER_BOUND ( 'NONE', #36117, .T. ) ;
#69205=CARTESIAN_POINT ( 'NONE',  ( 185.7024372569428294, 214.9312412210030061, 22.95886720168237005 ) ) ;
#69219=ORIENTED_EDGE ( 'NONE', *, *, #28532, .T. ) ;
#69221=ORIENTED_EDGE ( 'NONE', *, *, #12664, .T. ) ;
#69226=LINE ( 'NONE', #11460, #83945 ) ;
#69231=ORIENTED_EDGE ( 'NONE', *, *, #87554, .T. ) ;
#69251=ORIENTED_EDGE ( 'NONE', *, *, #19481, .T. ) ;
#69256=VERTEX_POINT ( 'NONE', #38967 ) ;
#69263=CARTESIAN_POINT ( 'NONE',  ( 197.2116943569230045, 250.0000000000000568, -12.92446933126075592 ) ) ;
#69268=CARTESIAN_POINT ( 'NONE',  ( 208.7500163748177897, 30.13141828311449189, 14.27675564571656253 ) ) ;
#69279=DIRECTION ( 'NONE',  ( 0.000000000000000000, 0.000000000000000000, 1.000000000000000000 ) ) ;
#69282=DIRECTION ( 'NONE',  ( -0.000000000000000000, -1.000000000000000000, -0.000000000000000000 ) ) ;
#69284=VERTEX_POINT ( 'NONE', #18146 ) ;
#69285=CARTESIAN_POINT ( 'NONE',  ( 156.3984609948128366, 15.95758591462681864, -7.138650918358526276 ) ) ;
#69287=CARTESIAN_POINT ( 'NONE',  ( 156.8041522122653930, 275.5000000000000568, 16.89672165344857646 ) ) ;
#69290=CARTESIAN_POINT ( 'NONE',  ( 157.2528655986806427, 19.19772955881777676, -10.67418916507680748 ) ) ;
#69298=ADVANCED_FACE ( 'NONE', ( #75903 ), #41462, .F. ) ;
#69300=VERTEX_POINT ( 'NONE', #31431 ) ;
#69305=ORIENTED_EDGE ( 'NONE', *, *, #13732, .F. ) ;
#69307=CARTESIAN_POINT ( 'NONE',  ( 152.4536156746142410, 275.5000000000000568, 12.00000000000000000 ) ) ;
#69319=ADVANCED_FACE ( 'NONE', ( #46540 ), #61261, .T. ) ;
#69322=LINE ( 'NONE', #4921, #42426 ) ;
#69335=ORIENTED_EDGE ( 'NONE', *, *, #72851, .T. ) ;
#69344=AXIS2_PLACEMENT_3D ( 'NONE', #65405, #57359, #29399 ) ;
#69370=DIRECTION ( 'NONE',  ( -0.3994899938748465162, 0.000000000000000000, -0.9167375550253601402 ) ) ;
#69382=CARTESIAN_POINT ( 'NONE',  ( 154.0637704119390321, 19.72112694978656222, -13.30738029212319695 ) ) ;
#69392=CARTESIAN_POINT ( 'NONE',  ( 196.0143093133015384, 73.40565171261609123, 11.99999999999998757 ) ) ;
#69396=CARTESIAN_POINT ( 'NONE',  ( 197.0547923074542780, 42.37849028824485487, 12.19783058971606593 ) ) ;
#69403=ADVANCED_FACE ( 'NONE', ( #67879 ), #18611, .T. ) ;
#69416=CARTESIAN_POINT ( 'NONE',  ( 196.8803347170859865, 24.42324672360809856, 12.49999999999999289 ) ) ;
#69429=EDGE_CURVE ( 'NONE', #77857, #17873, #39896, .T. ) ;
#69435=FACE_OUTER_BOUND ( 'NONE', #38123, .T. ) ;
#69445=ORIENTED_EDGE ( 'NONE', *, *, #9361, .F. ) ;
#69446=ORIENTED_EDGE ( 'NONE', *, *, #21097, .T. ) ;
#69455=PLANE ( 'NONE',  #74693 ) ;
#69456=CARTESIAN_POINT ( 'NONE',  ( 159.4851178187871312, 15.00000000000000000, -9.000000000000001776 ) ) ;
#69460=ORIENTED_EDGE ( 'NONE', *, *, #56503, .F. ) ;
#69476=CARTESIAN_POINT ( 'NONE',  ( 222.8344101925596306, 2.184664232470858947E-16, -8.757359312880716118 ) ) ;
#69487=CARTESIAN_POINT ( 'NONE',  ( 197.1033433601519107, 72.78980819445995110, -12.11496968317325873 ) ) ;
#69489=VERTEX_POINT ( 'NONE', #92318 ) ;
#69490=ORIENTED_EDGE ( 'NONE', *, *, #24839, .F. ) ;
#69491=CARTESIAN_POINT ( 'NONE',  ( 197.3663942936549347, 19.61288093082368533, 11.77299963048777620 ) ) ;
#69493=EDGE_CURVE ( 'NONE', #53411, #84479, #61817, .T. ) ;
#69506=CARTESIAN_POINT ( 'NONE',  ( 189.9243309297870610, 275.0000000000000568, 20.22542485937349355 ) ) ;
#69507=CARTESIAN_POINT ( 'NONE',  ( 195.5238343228637916, 40.22264805511078833, 13.82193646908953610 ) ) ;
#69519=CARTESIAN_POINT ( 'NONE',  ( 209.9972545312790544, 27.55378999303206200, 10.50000000000000000 ) ) ;
#69521=B_SPLINE_CURVE_WITH_KNOTS ( 'NONE', 3,
 ( #54594, #17231, #62187, #25711 ),
 .UNSPECIFIED., .F., .F.,
 ( 4, 4 ),
 ( 0.000000000000000000, 9.632970524402617444E-05 ),
 .UNSPECIFIED. ) ;
#69531=CARTESIAN_POINT ( 'NONE',  ( 196.1569681665548330, 42.06793861907576826, 13.67794394913816447 ) ) ;
#69538=B_SPLINE_CURVE_WITH_KNOTS ( 'NONE', 3,
 ( #33681, #40289, #55937, #69205, #77719, #70626 ),
 .UNSPECIFIED., .F., .F.,
 ( 4, 2, 4 ),
 ( 0.0002823611672359634833, 0.0005641097415182887501, 0.0008458583158006138542 ),
 .UNSPECIFIED. ) ;
#69541=CARTESIAN_POINT ( 'NONE',  ( 175.2296996224750103, 133.0000000000000000, -24.00000000000001066 ) ) ;
#69543=DIRECTION ( 'NONE',  ( 0.000000000000000000, 0.000000000000000000, -1.000000000000000000 ) ) ;
#69553=EDGE_CURVE ( 'NONE', #31710, #5311, #79078, .T. ) ;
#69560=ADVANCED_FACE ( 'NONE', ( #75442 ), #67424, .F. ) ;
#69563=ORIENTED_EDGE ( 'NONE', *, *, #82280, .T. ) ;
#69567=DIRECTION ( 'NONE',  ( 0.000000000000000000, 0.000000000000000000, 1.000000000000000000 ) ) ;
#69568=CARTESIAN_POINT ( 'NONE',  ( 195.0811277873548306, 27.06158795357637104, 15.19607843539318104 ) ) ;
#69588=CARTESIAN_POINT ( 'NONE',  ( 200.2296996224750103, 68.12454877777268791, 0.000000000000000000 ) ) ;
#69604=DIRECTION ( 'NONE',  ( 1.000000000000000000, 0.000000000000000000, -0.000000000000000000 ) ) ;
#69609=AXIS2_PLACEMENT_3D ( 'NONE', #5159, #48210, #71429 ) ;
#69616=VECTOR ( 'NONE', #48551, 1000.000000000000000 ) ;
#69628=CARTESIAN_POINT ( 'NONE',  ( 156.4851178187871312, 0.000000000000000000, 7.000000000000000000 ) ) ;
#69630=DIRECTION ( 'NONE',  ( -0.3024135303175699008, -0.9531768234073173529, 0.000000000000000000 ) ) ;
#69638=CARTESIAN_POINT ( 'NONE',  ( 153.1745786719506270, 129.2309077672098283, -12.62609896151546351 ) ) ;
#69643=CARTESIAN_POINT ( 'NONE',  ( 164.2231345125756263, 250.0000000000000568, 22.80382896337009058 ) ) ;
#69653=DIRECTION ( 'NONE',  ( 0.000000000000000000, 0.000000000000000000, -1.000000000000000000 ) ) ;
#69669=LINE ( 'NONE', #54994, #32975 ) ;
#69673=AXIS2_PLACEMENT_3D ( 'NONE', #13909, #50338, #50815 ) ;
#69684=EDGE_LOOP ( 'NONE', ( #59926, #21444, #74825, #65100 ) ) ;
#69686=ORIENTED_EDGE ( 'NONE', *, *, #43760, .T. ) ;
#69691=FACE_OUTER_BOUND ( 'NONE', #71469, .T. ) ;
#69696=ORIENTED_EDGE ( 'NONE', *, *, #42665, .F. ) ;
#69708=EDGE_LOOP ( 'NONE', ( #56078, #56671, #13267, #90871 ) ) ;
#69715=ORIENTED_EDGE ( 'NONE', *, *, #70808, .F. ) ;
#69716=DIRECTION ( 'NONE',  ( -0.000000000000000000, -1.000000000000000000, -0.000000000000000000 ) ) ;
#69720=ORIENTED_EDGE ( 'NONE', *, *, #42294, .F. ) ;
#69732=CARTESIAN_POINT ( 'NONE',  ( 208.2607500777332064, 30.15285273545742228, 15.07857486252943069 ) ) ;
#69734=EDGE_CURVE ( 'NONE', #1176, #39726, #50334, .T. ) ;
#69744=DIRECTION ( 'NONE',  ( 1.000000000000000000, 0.000000000000000000, 0.000000000000000000 ) ) ;
#69745=DIRECTION ( 'NONE',  ( -0.3024135303179443235, -0.9531768234071985590, 0.000000000000000000 ) ) ;
#69747=VECTOR ( 'NONE', #36372, 1000.000000000000000 ) ;
#69752=ORIENTED_EDGE ( 'NONE', *, *, #75074, .F. ) ;
#69753=CARTESIAN_POINT ( 'NONE',  ( 203.5977283565847813, 62.01285785379745619, 6.999999999999999112 ) ) ;
#69755=CARTESIAN_POINT ( 'NONE',  ( 206.0205385567603571, 30.15663536185482485, 14.00000000000000000 ) ) ;
#69768=EDGE_CURVE ( 'NONE', #17873, #64817, #24647, .T. ) ;
#69769=VERTEX_POINT ( 'NONE', #6643 ) ;
#69772=CARTESIAN_POINT ( 'NONE',  ( 157.4851178187871312, 1.000000000000000888, -7.000000000000000888 ) ) ;
#69790=CARTESIAN_POINT ( 'NONE',  ( 165.0427047786672290, 275.5000000000000568, 23.37680765314704701 ) ) ;
#69797=CARTESIAN_POINT ( 'NONE',  ( 201.2104617360081704, 60.19600395700749829, 10.00000000000000000 ) ) ;
#69805=ORIENTED_EDGE ( 'NONE', *, *, #47697, .F. ) ;
#69835=VERTEX_POINT ( 'NONE', #87533 ) ;
#69842=DIRECTION ( 'NONE',  ( 0.6056179655966478226, -0.7957555401921982963, 0.000000000000000000 ) ) ;
#69848=DIRECTION ( 'NONE',  ( 8.659560562354797273E-17, -0.7071067811865584529, 0.7071067811865364705 ) ) ;
#69855=CARTESIAN_POINT ( 'NONE',  ( 196.9534188175200029, 25.84350552936208700, 12.42857142857141817 ) ) ;
#69864=DIRECTION ( 'NONE',  ( 1.000000000000000000, 0.000000000000000000, 0.000000000000000000 ) ) ;
#69868=CARTESIAN_POINT ( 'NONE',  ( 189.9243309297870610, 215.0000000000000568, 20.22542485937349355 ) ) ;
#69878=CIRCLE ( 'NONE', #272, 0.5000000000000004441 ) ;
#69882=CARTESIAN_POINT ( 'NONE',  ( 208.6208076322478746, 32.98517505407394168, 10.00000000000000000 ) ) ;
#69886=CARTESIAN_POINT ( 'NONE',  ( 150.6539576904058606, 293.9636489450775230, 9.103929867429224387 ) ) ;
#69904=DIRECTION ( 'NONE',  ( -0.8435586647355782786, 0.000000000000000000, -0.5370370370370447510 ) ) ;
#69913=EDGE_CURVE ( 'NONE', #74736, #2640, #52740, .T. ) ;
#69925=DIRECTION ( 'NONE',  ( -0.000000000000000000, -1.000000000000000000, -0.000000000000000000 ) ) ;
#69930=ORIENTED_EDGE ( 'NONE', *, *, #71404, .F. ) ;
#69939=EDGE_LOOP ( 'NONE', ( #89851, #11569, #80625, #89457 ) ) ;
#69946=EDGE_CURVE ( 'NONE', #19714, #52231, #86619, .T. ) ;
#69949=VECTOR ( 'NONE', #46683, 1000.000000000000000 ) ;
#69957=CARTESIAN_POINT ( 'NONE',  ( 207.6679626695819820, 29.67996584739399069, 14.87498546835752222 ) ) ;
#69959=FACE_OUTER_BOUND ( 'NONE', #22746, .T. ) ;
#69960=AXIS2_PLACEMENT_3D ( 'NONE', #51132, #85714, #20859 ) ;
#69962=VERTEX_POINT ( 'NONE', #58690 ) ;
#69964=CARTESIAN_POINT ( 'NONE',  ( 197.7323754217920282, 18.47808631421187542, 11.36704352365794790 ) ) ;
#69967=EDGE_CURVE ( 'NONE', #59928, #57748, #50597, .T. ) ;
#69980=DIRECTION ( 'NONE',  ( -1.000000000000000000, 0.000000000000000000, 0.000000000000000000 ) ) ;
#69993=CARTESIAN_POINT ( 'NONE',  ( 195.0811277904324754, 27.48493576247232895, 15.19607843137254477 ) ) ;
#70005=CARTESIAN_POINT ( 'NONE',  ( 195.8476942551502020, 41.45913785700680165, 14.14010213890159484 ) ) ;
#70010=AXIS2_PLACEMENT_3D ( 'NONE', #63953, #36438, #58240 ) ;
#70015=ORIENTED_EDGE ( 'NONE', *, *, #66150, .T. ) ;
#70016=DIRECTION ( 'NONE',  ( -0.000000000000000000, -1.000000000000000000, -0.000000000000000000 ) ) ;
#70019=LINE ( 'NONE', #39235, #85186 ) ;
#70025=AXIS2_PLACEMENT_3D ( 'NONE', #38554, #8734, #16778 ) ;
#70030=VERTEX_POINT ( 'NONE', #57765 ) ;
#70031=LINE ( 'NONE', #88634, #43985 ) ;
#70035=AXIS2_PLACEMENT_3D ( 'NONE', #10107, #11035, #54131 ) ;
#70036=ADVANCED_FACE ( 'NONE', ( #78603 ), #51554, .F. ) ;
#70044=DIRECTION ( 'NONE',  ( -0.000000000000000000, -0.000000000000000000, -1.000000000000000000 ) ) ;
#70045=TOROIDAL_SURFACE ( 'NONE', #35297, 24.50000000000000355, 0.5000000000000000000 ) ;
#70046=DIRECTION ( 'NONE',  ( 1.000000000000000000, 0.000000000000000000, -0.000000000000000000 ) ) ;
#70047=LINE ( 'NONE', #91799, #37055 ) ;
#70058=VECTOR ( 'NONE', #44954, 1000.000000000000000 ) ;
#70059=ORIENTED_EDGE ( 'NONE', *, *, #76674, .F. ) ;
#70067=EDGE_CURVE ( 'NONE', #18551, #74338, #71987, .T. ) ;
#70069=ORIENTED_EDGE ( 'NONE', *, *, #43842, .F. ) ;
#70070=LINE ( 'NONE', #54903, #3032 ) ;
#70085=CARTESIAN_POINT ( 'NONE',  ( 154.7659666677360235, 19.56018909072649237, -12.94946946942526189 ) ) ;
#70087=AXIS2_PLACEMENT_3D ( 'NONE', #14563, #50530, #27841 ) ;
#70097=AXIS2_PLACEMENT_3D ( 'NONE', #14773, #85780, #65911 ) ;
#70103=AXIS2_PLACEMENT_3D ( 'NONE', #79330, #28658, #27730 ) ;
#70111=AXIS2_PLACEMENT_3D ( 'NONE', #40249, #40711, #48772 ) ;
#70112=ADVANCED_FACE ( 'NONE', ( #65822 ), #26200, .T. ) ;
#70127=VECTOR ( 'NONE', #74678, 1000.000000000000000 ) ;
#70128=DIRECTION ( 'NONE',  ( -1.000000000000000000, 0.000000000000000000, 0.000000000000000000 ) ) ;
#70130=LINE ( 'NONE', #62562, #74395 ) ;
#70140=ORIENTED_EDGE ( 'NONE', *, *, #36317, .F. ) ;
#70143=CIRCLE ( 'NONE', #29316, 0.5000000000000004441 ) ;
#70144=DIRECTION ( 'NONE',  ( 0.000000000000000000, 0.000000000000000000, 1.000000000000000000 ) ) ;
#70157=EDGE_CURVE ( 'NONE', #12291, #41724, #85139, .T. ) ;
#70168=TOROIDAL_SURFACE ( 'NONE', #617, 24.16304133878946558, 4.003189038634632269 ) ;
#70174=ORIENTED_EDGE ( 'NONE', *, *, #58173, .T. ) ;
#70200=VERTEX_POINT ( 'NONE', #43082 ) ;
#70209=DIRECTION ( 'NONE',  ( 0.000000000000000000, 0.000000000000000000, 1.000000000000000000 ) ) ;
#70224=LINE ( 'NONE', #11020, #18563 ) ;
#70232=EDGE_CURVE ( 'NONE', #34264, #70640, #22233, .T. ) ;
#70235=CARTESIAN_POINT ( 'NONE',  ( 175.2296996224750103, 158.6892791692949629, 0.000000000000000000 ) ) ;
#70236=PLANE ( 'NONE',  #27733 ) ;
#70246=LINE ( 'NONE', #41794, #24050 ) ;
#70260=ORIENTED_EDGE ( 'NONE', *, *, #17026, .T. ) ;
#70265=VERTEX_POINT ( 'NONE', #57308 ) ;
#70267=CARTESIAN_POINT ( 'NONE',  ( 189.9243309297870610, 215.0000000000000568, 20.22542485937349355 ) ) ;
#70288=ADVANCED_FACE ( 'NONE', ( #85691 ), #29190, .T. ) ;
#70290=LINE ( 'NONE', #92975, #62186 ) ;
#70318=VERTEX_POINT ( 'NONE', #14222 ) ;
#70336=CARTESIAN_POINT ( 'NONE',  ( 152.9200301536558584, 20.54241773159133899, -11.30461213543805599 ) ) ;
#70349=DIRECTION ( 'NONE',  ( -0.2456588035076220367, 0.9693563597868450898, 0.000000000000000000 ) ) ;
#70354=DIRECTION ( 'NONE',  ( 0.000000000000000000, -1.000000000000000000, 0.000000000000000000 ) ) ;
#70361=CARTESIAN_POINT ( 'NONE',  ( 196.9658976021800356, 41.89417665433578009, 12.94436659007928547 ) ) ;
#70362=CARTESIAN_POINT ( 'NONE',  ( 197.3133474189782248, 24.42324672360810212, 12.74999999999999112 ) ) ;
#70375=DIRECTION ( 'NONE',  ( -1.000000000000000000, 0.000000000000000000, 0.000000000000000000 ) ) ;
#70395=CARTESIAN_POINT ( 'NONE',  ( 201.1937845308156341, 300.0127519931331790, -5.237596670121819287 ) ) ;
#70399=EDGE_CURVE ( 'NONE', #64853, #34296, #60955, .T. ) ;
#70407=ORIENTED_EDGE ( 'NONE', *, *, #54121, .T. ) ;
#70408=ORIENTED_EDGE ( 'NONE', *, *, #41382, .F. ) ;
#70419=DIRECTION ( 'NONE',  ( -0.000000000000000000, -1.000000000000000000, -0.000000000000000000 ) ) ;
#70423=EDGE_LOOP ( 'NONE', ( #4684, #12191, #68630, #8981 ) ) ;
#70436=ORIENTED_EDGE ( 'NONE', *, *, #62500, .F. ) ;
#70446=CARTESIAN_POINT ( 'NONE',  ( 194.4755092218382799, 40.71494654549765357, 14.33893281099658346 ) ) ;
#70448=VERTEX_POINT ( 'NONE', #17462 ) ;
#70450=DIRECTION ( 'NONE',  ( 0.000000000000000000, 0.000000000000000000, 1.000000000000000000 ) ) ;
#70477=DIRECTION ( 'NONE',  ( 1.000000000000000000, 0.000000000000000000, 0.000000000000000000 ) ) ;
#70479=CARTESIAN_POINT ( 'NONE',  ( 175.2296996224750103, 149.6461846693799487, 0.000000000000000000 ) ) ;
#70491=CARTESIAN_POINT ( 'NONE',  ( 195.5093152655051938, 40.06852958779855811, 14.92626378859575809 ) ) ;
#70500=ORIENTED_EDGE ( 'NONE', *, *, #74108, .T. ) ;
#70501=CARTESIAN_POINT ( 'NONE',  ( 157.4851178187871312, 1.000000000000000888, -7.000000000000000888 ) ) ;
#70503=CARTESIAN_POINT ( 'NONE',  ( 208.0345994753939181, 28.60382334453963082, 12.94649967097967647 ) ) ;
#70513=VERTEX_POINT ( 'NONE', #73364 ) ;
#70514=CARTESIAN_POINT ( 'NONE',  ( 194.8940620914166573, 40.53306711095739701, 13.77184909798794621 ) ) ;
#70517=CARTESIAN_POINT ( 'NONE',  ( 197.7129307445490269, 68.09401877024910732, -12.80442219784224811 ) ) ;
#70518=ADVANCED_FACE ( 'NONE', ( #87996 ), #53428, .T. ) ;
#70520=ORIENTED_EDGE ( 'NONE', *, *, #69090, .T. ) ;
#70531=ORIENTED_EDGE ( 'NONE', *, *, #82892, .T. ) ;
#70538=ORIENTED_EDGE ( 'NONE', *, *, #55137, .F. ) ;
#70547=EDGE_LOOP ( 'NONE', ( #58897, #72051, #79973, #69930 ) ) ;
#70562=EDGE_LOOP ( 'NONE', ( #29982, #87042, #24278, #27694 ) ) ;
#70564=CARTESIAN_POINT ( 'NONE',  ( 200.2349812190172713, 66.43136063442170780, 7.741079165001067963 ) ) ;
#70571=DIRECTION ( 'NONE',  ( 0.000000000000000000, 1.000000000000000000, 0.000000000000000000 ) ) ;
#70577=CARTESIAN_POINT ( 'NONE',  ( 193.9646936176702070, 21.00000000000000000, 15.00000000000000000 ) ) ;
#70596=CARTESIAN_POINT ( 'NONE',  ( 201.2104617360081704, 250.0000000000000568, 15.00000000000000000 ) ) ;
#70609=ORIENTED_EDGE ( 'NONE', *, *, #14384, .F. ) ;
#70612=CARTESIAN_POINT ( 'NONE',  ( 140.6539576904058606, 275.0000000000000568, 10.50000000000000000 ) ) ;
#70624=DIRECTION ( 'NONE',  ( 1.000000000000000000, 0.000000000000000000, 0.000000000000000000 ) ) ;
#70626=CARTESIAN_POINT ( 'NONE',  ( 185.8264795993290477, 214.9910457053126720, 23.09031830825835385 ) ) ;
#70640=VERTEX_POINT ( 'NONE', #9873 ) ;
#70654=DIRECTION ( 'NONE',  ( 0.000000000000000000, 0.000000000000000000, 1.000000000000000000 ) ) ;
#70659=ORIENTED_EDGE ( 'NONE', *, *, #21995, .T. ) ;
#70666=ORIENTED_EDGE ( 'NONE', *, *, #89671, .T. ) ;
#70671=EDGE_LOOP ( 'NONE', ( #10873, #21814, #10530, #32586, #66699 ) ) ;
#70691=EDGE_CURVE ( 'NONE', #53738, #53411, #16062, .T. ) ;
#70694=CARTESIAN_POINT ( 'NONE',  ( 161.2244399300530233, 8.542400036368780647, 9.000000000000001776 ) ) ;
#70695=DIRECTION ( 'NONE',  ( 0.000000000000000000, 0.000000000000000000, 1.000000000000000000 ) ) ;
#70708=CARTESIAN_POINT ( 'NONE',  ( 175.2296996224750103, 247.0000000000001137, 8.550761578869359170 ) ) ;
#70718=ORIENTED_EDGE ( 'NONE', *, *, #14576, .F. ) ;
#70746=CARTESIAN_POINT ( 'NONE',  ( 199.1087447750284980, 64.61450673763175701, 10.46317447812566570 ) ) ;
#70753=EDGE_CURVE ( 'NONE', #2466, #20445, #33780, .T. ) ;
#70755=EDGE_LOOP ( 'NONE', ( #33257, #42629, #90182, #30570 ) ) ;
#70758=VERTEX_POINT ( 'NONE', #75217 ) ;
#70776=VERTEX_POINT ( 'NONE', #66716 ) ;
#70790=DIRECTION ( 'NONE',  ( 0.000000000000000000, 0.000000000000000000, 1.000000000000000000 ) ) ;
#70795=LINE ( 'NONE', #63715, #85282 ) ;
#70802=DIRECTION ( 'NONE',  ( 0.000000000000000000, 1.000000000000000000, 0.000000000000000000 ) ) ;
#70805=VECTOR ( 'NONE', #60610, 1000.000000000000114 ) ;
#70808=EDGE_CURVE ( 'NONE', #1443, #33827, #13171, .T. ) ;
#70810=DIRECTION ( 'NONE',  ( 0.000000000000000000, -0.000000000000000000, 1.000000000000000000 ) ) ;
#70813=CARTESIAN_POINT ( 'NONE',  ( 165.2494399300530290, 8.542400036368780647, 10.00000000000000000 ) ) ;
#70846=AXIS2_PLACEMENT_3D ( 'NONE', #18745, #84987, #49025 ) ;
#70850=CARTESIAN_POINT ( 'NONE',  ( 154.9065949031809453, 18.65395765032405961, 9.525636664968139655 ) ) ;
#70861=ORIENTED_EDGE ( 'NONE', *, *, #82755, .F. ) ;
#70871=CARTESIAN_POINT ( 'NONE',  ( 153.6987871352711181, 19.48326534539917887, -11.45812909362560639 ) ) ;
#70872=CARTESIAN_POINT ( 'NONE',  ( 153.4133700136260927, 129.9709486557056834, -11.65454253063697898 ) ) ;
#70885=ADVANCED_FACE ( 'NONE', ( #10331 ), #65730, .T. ) ;
#70890=ORIENTED_EDGE ( 'NONE', *, *, #83847, .F. ) ;
#70891=DIRECTION ( 'NONE',  ( -0.000000000000000000, 0.000000000000000000, -1.000000000000000000 ) ) ;
#70892=CARTESIAN_POINT ( 'NONE',  ( 180.5131398354828320, 250.5000000000000568, -23.92352941176473635 ) ) ;
#70898=CARTESIAN_POINT ( 'NONE',  ( 154.3452702497934013, 20.31595811206259938, 11.82731014213360510 ) ) ;
#70899=CARTESIAN_POINT ( 'NONE',  ( 197.2116943569230045, 250.0000000000000568, -12.92446933126075592 ) ) ;
#70901=ORIENTED_EDGE ( 'NONE', *, *, #59380, .F. ) ;
#70902=EDGE_LOOP ( 'NONE', ( #28449, #26601, #24127, #33730 ) ) ;
#70903=CARTESIAN_POINT ( 'NONE',  ( 140.6539576904058606, 249.5000000000000568, -12.50000000000000000 ) ) ;
#70910=AXIS2_PLACEMENT_3D ( 'NONE', #42258, #35169, #85816 ) ;
#70918=DIRECTION ( 'NONE',  ( -0.000000000000000000, -1.000000000000000000, -0.000000000000000000 ) ) ;
#70919=EDGE_CURVE ( 'NONE', #4814, #93104, #39756, .T. ) ;
#70920=ADVANCED_FACE ( 'NONE', ( #77078 ), #61942, .F. ) ;
#70921=DIRECTION ( 'NONE',  ( 0.000000000000000000, 0.000000000000000000, 1.000000000000000000 ) ) ;
#70948=CARTESIAN_POINT ( 'NONE',  ( 195.3159225978357085, 40.29405723410430795, 14.88612872638837636 ) ) ;
#70954=EDGE_CURVE ( 'NONE', #3752, #50728, #52957, .T. ) ;
#70958=CARTESIAN_POINT ( 'NONE',  ( 152.0139507567534736, 20.82771571514191677, 9.304222368691537071 ) ) ;
#70960=CARTESIAN_POINT ( 'NONE',  ( 196.3496553477289979, 276.0000000000000568, -12.41762739670150850 ) ) ;
#70983=CARTESIAN_POINT ( 'NONE',  ( 198.6884013828325521, 64.61450673763175701, -9.555809373750793867 ) ) ;
#70984=FACE_OUTER_BOUND ( 'NONE', #61295, .T. ) ;
#70985=DIRECTION ( 'NONE',  ( -0.000000000000000000, -0.000000000000000000, -1.000000000000000000 ) ) ;
#70994=ORIENTED_EDGE ( 'NONE', *, *, #88732, .F. ) ;
#71004=LINE ( 'NONE', #28847, #68061 ) ;
#71018=ORIENTED_EDGE ( 'NONE', *, *, #69429, .T. ) ;
#71019=ORIENTED_EDGE ( 'NONE', *, *, #16970, .T. ) ;
#71035=FACE_OUTER_BOUND ( 'NONE', #28505, .T. ) ;
#71036=ADVANCED_FACE ( 'NONE', ( #25478 ), #5121, .T. ) ;
#71037=DIRECTION ( 'NONE',  ( 0.000000000000000000, 0.000000000000000000, 1.000000000000000000 ) ) ;
#71047=VECTOR ( 'NONE', #59672, 1000.000000000000000 ) ;
#71058=CARTESIAN_POINT ( 'NONE',  ( 154.4030696693785956, 128.9756020784251120, 12.16842021443607180 ) ) ;
#71060=CARTESIAN_POINT ( 'NONE',  ( 175.2296996224750103, 160.0000000000000568, 0.000000000000000000 ) ) ;
#71072=CARTESIAN_POINT ( 'NONE',  ( 199.0061125298537377, 250.5000000000000568, -12.72542485937401580 ) ) ;
#71086=CARTESIAN_POINT ( 'NONE',  ( 185.1905923765118587, 275.0000000000000568, 21.83530662808691147 ) ) ;
#71106=CIRCLE ( 'NONE', #19724, 4.499999999999993783 ) ;
#71109=ORIENTED_EDGE ( 'NONE', *, *, #25741, .T. ) ;
#71112=AXIS2_PLACEMENT_3D ( 'NONE', #70596, #93284, #485 ) ;
#71117=DIRECTION ( 'NONE',  ( 0.000000000000000000, 0.000000000000000000, 1.000000000000000000 ) ) ;
#71123=EDGE_LOOP ( 'NONE', ( #19272, #67142 ) ) ;
#71130=ORIENTED_EDGE ( 'NONE', *, *, #36693, .T. ) ;
#71131=PLANE ( 'NONE',  #18640 ) ;
#71142=CARTESIAN_POINT ( 'NONE',  ( 164.2231345125756263, 250.5000000000000568, 22.80382896337008702 ) ) ;
#71152=EDGE_LOOP ( 'NONE', ( #59709, #70531, #32991, #34083 ) ) ;
#71157=EDGE_CURVE ( 'NONE', #70, #46709, #93332, .T. ) ;
#71160=FACE_OUTER_BOUND ( 'NONE', #25072, .T. ) ;
#71161=CARTESIAN_POINT ( 'NONE',  ( 184.1778392089217107, 3.000000000000000000, 10.00000000000000178 ) ) ;
#71165=EDGE_CURVE ( 'NONE', #557, #72022, #56434, .T. ) ;
#71170=DIRECTION ( 'NONE',  ( -0.000000000000000000, -1.000000000000000000, -0.000000000000000000 ) ) ;
#71175=DIRECTION ( 'NONE',  ( 0.000000000000000000, -1.000000000000000000, 0.000000000000000000 ) ) ;
#71185=AXIS2_PLACEMENT_3D ( 'NONE', #33329, #40404, #56059 ) ;
#71188=VECTOR ( 'NONE', #68372, 1000.000000000000000 ) ;
#71192=ORIENTED_EDGE ( 'NONE', *, *, #89368, .T. ) ;
#71202=ORIENTED_EDGE ( 'NONE', *, *, #89067, .T. ) ;
#71216=DIRECTION ( 'NONE',  ( 1.000000000000000000, 0.000000000000000000, 0.000000000000000000 ) ) ;
#71226=VERTEX_POINT ( 'NONE', #75672 ) ;
#71244=VERTEX_POINT ( 'NONE', #34466 ) ;
#71253=ORIENTED_EDGE ( 'NONE', *, *, #54587, .T. ) ;
#71254=EDGE_CURVE ( 'NONE', #21613, #25416, #63372, .T. ) ;
#71258=AXIS2_PLACEMENT_3D ( 'NONE', #24238, #2485, #2934 ) ;
#71262=PLANE ( 'NONE',  #44177 ) ;
#71281=DIRECTION ( 'NONE',  ( -0.000000000000000000, -0.000000000000000000, -1.000000000000000000 ) ) ;
#71290=EDGE_CURVE ( 'NONE', #28813, #34201, #11051, .T. ) ;
#71301=LINE ( 'NONE', #42389, #4448 ) ;
#71318=AXIS2_PLACEMENT_3D ( 'NONE', #93200, #77601, #56297 ) ;
#71329=EDGE_LOOP ( 'NONE', ( #6281, #44054, #68369, #3651, #44978 ) ) ;
#71330=EDGE_LOOP ( 'NONE', ( #84245, #61273, #86327, #60268 ) ) ;
#71341=CARTESIAN_POINT ( 'NONE',  ( 197.7051530045995094, 41.80213891112347824, 12.00000000000000000 ) ) ;
#71353=ORIENTED_EDGE ( 'NONE', *, *, #48163, .T. ) ;
#71357=ORIENTED_EDGE ( 'NONE', *, *, #6382, .F. ) ;
#71360=ADVANCED_FACE ( 'NONE', ( #85107 ), #20257, .T. ) ;
#71368=CARTESIAN_POINT ( 'NONE',  ( 180.2296971224742776, 215.0000000000000568, -25.00500000000002387 ) ) ;
#71371=CARTESIAN_POINT ( 'NONE',  ( 165.0461196878273711, 214.7033826592484616, 22.86486864458202817 ) ) ;
#71372=ORIENTED_EDGE ( 'NONE', *, *, #21877, .F. ) ;
#71373=DIRECTION ( 'NONE',  ( -0.000000000000000000, -1.000000000000000000, -0.000000000000000000 ) ) ;
#71382=AXIS2_PLACEMENT_3D ( 'NONE', #59011, #1701, #68806 ) ;
#71386=AXIS2_PLACEMENT_3D ( 'NONE', #29476, #60214, #89053 ) ;
#71389=CARTESIAN_POINT ( 'NONE',  ( 196.8088576720463436, 292.7107012191569311, -7.905027250450429754 ) ) ;
#71392=AXIS2_PLACEMENT_3D ( 'NONE', #86748, #42730, #71645 ) ;
#71404=EDGE_CURVE ( 'NONE', #29329, #24735, #30122, .T. ) ;
#71419=DIRECTION ( 'NONE',  ( 0.000000000000000000, 0.000000000000000000, 1.000000000000000000 ) ) ;
#71428=VERTEX_POINT ( 'NONE', #64777 ) ;
#71429=DIRECTION ( 'NONE',  ( 0.7957555401921969640, 0.6056179655966498210, 0.000000000000000000 ) ) ;
#71440=ORIENTED_EDGE ( 'NONE', *, *, #8954, .T. ) ;
#71441=CARTESIAN_POINT ( 'NONE',  ( 194.2991910711363346, 39.77461757278994980, 14.57244569840369053 ) ) ;
#71446=VERTEX_POINT ( 'NONE', #42960 ) ;
#71453=CARTESIAN_POINT ( 'NONE',  ( 199.6702811234769683, 65.52214591209386185, -9.100946541886337116 ) ) ;
#71456=CARTESIAN_POINT ( 'NONE',  ( 201.2104617360081704, 41.21457449016152452, 9.000000000000000000 ) ) ;
#71459=VERTEX_POINT ( 'NONE', #49133 ) ;
#71464=ADVANCED_FACE ( 'NONE', ( #64320 ), #42005, .T. ) ;
#71466=CIRCLE ( 'NONE', #69960, 10.55076157886938937 ) ;
#71469=EDGE_LOOP ( 'NONE', ( #31280, #77584, #63229, #72869 ) ) ;
#71493=ORIENTED_EDGE ( 'NONE', *, *, #52972, .F. ) ;
#71494=ORIENTED_EDGE ( 'NONE', *, *, #66418, .T. ) ;
#71509=CARTESIAN_POINT ( 'NONE',  ( 199.8839601301601476, 66.89258700487513920, -4.790067391029595001 ) ) ;
#71510=DIRECTION ( 'NONE',  ( 0.000000000000000000, 1.000000000000000000, 0.000000000000000000 ) ) ;
#71520=DIRECTION ( 'NONE',  ( 0.000000000000000000, -1.000000000000000000, -0.000000000000000000 ) ) ;
#71526=VECTOR ( 'NONE', #13143, 1000.000000000000000 ) ;
#71534=CIRCLE ( 'NONE', #27723, 24.00000000000000711 ) ;
#71535=FACE_OUTER_BOUND ( 'NONE', #71329, .T. ) ;
#71537=CARTESIAN_POINT ( 'NONE',  ( 197.8646367605500700, 70.82932363588079738, -10.83694520234208269 ) ) ;
#71547=DIRECTION ( 'NONE',  ( 0.000000000000000000, 1.000000000000000000, 0.000000000000000000 ) ) ;
#71556=AXIS2_PLACEMENT_3D ( 'NONE', #70612, #77229, #32741 ) ;
#71563=DIRECTION ( 'NONE',  ( -0.000000000000000000, 1.000000000000000000, -0.000000000000000000 ) ) ;
#71564=CYLINDRICAL_SURFACE ( 'NONE', #69344, 0.5000000000000004441 ) ;
#71569=EDGE_CURVE ( 'NONE', #28384, #33195, #63838, .T. ) ;
#71586=AXIS2_PLACEMENT_3D ( 'NONE', #48414, #61715, #25707 ) ;
#71592=DIRECTION ( 'NONE',  ( 0.000000000000000000, 1.000000000000000000, 0.000000000000000000 ) ) ;
#71606=ORIENTED_EDGE ( 'NONE', *, *, #34585, .F. ) ;
#71607=CARTESIAN_POINT ( 'NONE',  ( 195.5480150185777291, 26.67257684198393974, 13.83492282920820493 ) ) ;
#71618=FACE_BOUND ( 'NONE', #45508, .T. ) ;
#71619=CIRCLE ( 'NONE', #76119, 4.999999999999976907 ) ;
#71628=AXIS2_PLACEMENT_3D ( 'NONE', #55813, #11317, #90358 ) ;
#71635=CARTESIAN_POINT ( 'NONE',  ( 153.6948129392865781, 20.34864080145124987, 12.70029817130066441 ) ) ;
#71640=DIRECTION ( 'NONE',  ( 0.000000000000000000, 0.000000000000000000, 1.000000000000000000 ) ) ;
#71645=DIRECTION ( 'NONE',  ( -0.9953184226294286008, 0.000000000000000000, 0.09665007798479169354 ) ) ;
#71646=DIRECTION ( 'NONE',  ( -0.000000000000000000, 0.000000000000000000, -1.000000000000000000 ) ) ;
#71653=AXIS2_PLACEMENT_3D ( 'NONE', #5942, #86384, #71758 ) ;
#71657=ORIENTED_EDGE ( 'NONE', *, *, #13861, .T. ) ;
#71658=AXIS2_PLACEMENT_3D ( 'NONE', #25461, #54805, #82751 ) ;
#71661=LINE ( 'NONE', #57907, #77552 ) ;
#71667=AXIS2_PLACEMENT_3D ( 'NONE', #86391, #34360, #56138 ) ;
#71678=AXIS2_PLACEMENT_3D ( 'NONE', #21599, #43374, #72269 ) ;
#71679=EDGE_CURVE ( 'NONE', #42461, #31710, #14133, .T. ) ;
#71682=DIRECTION ( 'NONE',  ( 0.000000000000000000, 0.000000000000000000, 1.000000000000000000 ) ) ;
#71699=EDGE_LOOP ( 'NONE', ( #11954, #23131, #52211, #50794, #85870 ) ) ;
#71702=ORIENTED_EDGE ( 'NONE', *, *, #11258, .F. ) ;
#71729=ORIENTED_EDGE ( 'NONE', *, *, #44269, .T. ) ;
#71733=CIRCLE ( 'NONE', #86835, 0.5000000000000129896 ) ;
#71739=DIRECTION ( 'NONE',  ( 0.000000000000000000, -0.000000000000000000, 1.000000000000000000 ) ) ;
#71748=AXIS2_PLACEMENT_3D ( 'NONE', #43163, #71117, #78223 ) ;
#71758=DIRECTION ( 'NONE',  ( -0.8435586647355751699, 0.000000000000000000, -0.5370370370370497470 ) ) ;
#71761=CIRCLE ( 'NONE', #38461, 4.103083949679980691 ) ;
#71766=FACE_OUTER_BOUND ( 'NONE', #78746, .T. ) ;
#71792=EDGE_CURVE ( 'NONE', #84462, #25231, #7892, .T. ) ;
#71811=CIRCLE ( 'NONE', #760, 25.00000000000000355 ) ;
#71813=ADVANCED_FACE ( 'NONE', ( #72315 ), #21653, .T. ) ;
#71819=LINE ( 'NONE', #20676, #628 ) ;
#71822=AXIS2_PLACEMENT_3D ( 'NONE', #88427, #404, #1791 ) ;
#71825=EDGE_LOOP ( 'NONE', ( #61244, #80508, #85673, #30336 ) ) ;
#71832=AXIS2_PLACEMENT_3D ( 'NONE', #6958, #93572, #28729 ) ;
#71838=ORIENTED_EDGE ( 'NONE', *, *, #71165, .T. ) ;
#71839=CARTESIAN_POINT ( 'NONE',  ( 156.0793278192250284, 19.94580804510101402, 11.55434249967772331 ) ) ;
#71845=CARTESIAN_POINT ( 'NONE',  ( 175.2296996224750103, 247.0000000000001137, -8.550761578869359170 ) ) ;
#71848=CARTESIAN_POINT ( 'NONE',  ( 183.0442525570908288, 300.2961574867697436, 7.500000000000000000 ) ) ;
#71850=VERTEX_POINT ( 'NONE', #28300 ) ;
#71851=CARTESIAN_POINT ( 'NONE',  ( 165.2494399300530290, 8.542400036368780647, 10.00000000000000000 ) ) ;
#71865=DIRECTION ( 'NONE',  ( -0.000000000000000000, 1.000000000000000000, -0.000000000000000000 ) ) ;
#71866=CARTESIAN_POINT ( 'NONE',  ( 201.2104617360081704, 250.0000000000000568, 15.00000000000000000 ) ) ;
#71893=CARTESIAN_POINT ( 'NONE',  ( 208.4306832106270519, 1.063508326895939771, 7.500000000000014211 ) ) ;
#71895=AXIS2_PLACEMENT_3D ( 'NONE', #3686, #33479, #62382 ) ;
#71908=ORIENTED_EDGE ( 'NONE', *, *, #20685, .F. ) ;
#71927=ORIENTED_EDGE ( 'NONE', *, *, #84467, .T. ) ;
#71933=CARTESIAN_POINT ( 'NONE',  ( 196.1375241020610076, 72.62792297770094763, -11.78658572562475904 ) ) ;
#71934=CARTESIAN_POINT ( 'NONE',  ( 206.6195589736935005, 30.30844190587212594, 15.00000000000000000 ) ) ;
#71937=ORIENTED_EDGE ( 'NONE', *, *, #8361, .T. ) ;
#71945=ORIENTED_EDGE ( 'NONE', *, *, #32453, .F. ) ;
#71955=CARTESIAN_POINT ( 'NONE',  ( 161.2244399300530233, 8.542400036368780647, -9.000000000000001776 ) ) ;
#71966=AXIS2_PLACEMENT_3D ( 'NONE', #15443, #29667, #58547 ) ;
#71970=EDGE_LOOP ( 'NONE', ( #16907, #26273 ) ) ;
#71971=CARTESIAN_POINT ( 'NONE',  ( 209.6287663260175975, 29.00782453271232697, 12.09245862095555601 ) ) ;
#71982=B_SPLINE_CURVE_WITH_KNOTS ( 'NONE', 3,
 ( #67200, #10805, #24553, #66724, #9881, #46321 ),
 .UNSPECIFIED., .F., .F.,
 ( 4, 2, 4 ),
 ( 0.002739916521960775609, 0.004109700271224535871, 0.005479484020488295699 ),
 .UNSPECIFIED. ) ;
#71986=CARTESIAN_POINT ( 'NONE',  ( 197.5277731218624524, 69.98851376389092138, -11.59179972303952866 ) ) ;
#71987=LINE ( 'NONE', #14683, #67036 ) ;
#71997=DIRECTION ( 'NONE',  ( 0.000000000000000000, 0.000000000000000000, 1.000000000000000000 ) ) ;
#71999=FACE_OUTER_BOUND ( 'NONE', #27902, .T. ) ;
#72006=EDGE_CURVE ( 'NONE', #54877, #83549, #57994, .T. ) ;
#72008=ADVANCED_FACE ( 'NONE', ( #45720 ), #74630, .T. ) ;
#72012=CARTESIAN_POINT ( 'NONE',  ( 199.5538737146232506, 67.40778408939276289, -8.432808456659151020 ) ) ;
#72022=VERTEX_POINT ( 'NONE', #1264 ) ;
#72023=FACE_OUTER_BOUND ( 'NONE', #19612, .T. ) ;
#72025=CARTESIAN_POINT ( 'NONE',  ( 160.5350683151633291, 276.0000000000000568, 24.72542485937379197 ) ) ;
#72039=DIRECTION ( 'NONE',  ( 0.000000000000000000, 0.000000000000000000, 1.000000000000000000 ) ) ;
#72051=ORIENTED_EDGE ( 'NONE', *, *, #64191, .F. ) ;
#72064=DIRECTION ( 'NONE',  ( -0.000000000000000000, -1.000000000000000000, -0.000000000000000000 ) ) ;
#72078=CARTESIAN_POINT ( 'NONE',  ( 195.9076712334997694, 25.46858585516271845, 12.18710226207752712 ) ) ;
#72094=EDGE_CURVE ( 'NONE', #4814, #48695, #59477, .T. ) ;
#72108=EDGE_CURVE ( 'NONE', #84479, #5104, #83085, .T. ) ;
#72110=CARTESIAN_POINT ( 'NONE',  ( 209.9779462868543760, 37.90836112277824554, 13.95111757441427258 ) ) ;
#72115=DIRECTION ( 'NONE',  ( 0.000000000000000000, 1.000000000000000000, 0.000000000000000000 ) ) ;
#72128=CARTESIAN_POINT ( 'NONE',  ( 197.3235832258322375, 41.90495390785805796, 12.40447841451800848 ) ) ;
#72130=ORIENTED_EDGE ( 'NONE', *, *, #81029, .F. ) ;
#72185=ORIENTED_EDGE ( 'NONE', *, *, #46507, .T. ) ;
#72188=ORIENTED_EDGE ( 'NONE', *, *, #55616, .F. ) ;
#72197=CARTESIAN_POINT ( 'NONE',  ( 0.000000000000000000, 3.000000000000000000, -9.000000000000001776 ) ) ;
#72202=DIRECTION ( 'NONE',  ( 0.000000000000000000, 0.000000000000000000, 1.000000000000000000 ) ) ;
#72209=FACE_OUTER_BOUND ( 'NONE', #83422, .T. ) ;
#72224=EDGE_CURVE ( 'NONE', #26503, #23662, #91675, .T. ) ;
#72232=DIRECTION ( 'NONE',  ( 0.000000000000000000, 0.000000000000000000, 1.000000000000000000 ) ) ;
#72269=DIRECTION ( 'NONE',  ( 0.000000000000000000, -0.000000000000000000, 1.000000000000000000 ) ) ;
#72283=ORIENTED_EDGE ( 'NONE', *, *, #26014, .F. ) ;
#72289=VECTOR ( 'NONE', #45428, 1000.000000000000000 ) ;
#72292=CARTESIAN_POINT ( 'NONE',  ( 209.8744251295252354, 28.03846817292548366, 12.09245862095555601 ) ) ;
#72293=CARTESIAN_POINT ( 'NONE',  ( 158.6539576904058606, 293.9636489450775230, 0.000000000000000000 ) ) ;
#72295=DIRECTION ( 'NONE',  ( 0.000000000000000000, 0.000000000000000000, 1.000000000000000000 ) ) ;
#72299=DIRECTION ( 'NONE',  ( -0.000000000000000000, -1.000000000000000000, -0.000000000000000000 ) ) ;
#72314=DIRECTION ( 'NONE',  ( -0.9565177946839410472, -1.517921082078008940E-15, 0.2916739763039721267 ) ) ;
#72315=FACE_OUTER_BOUND ( 'NONE', #73290, .T. ) ;
#72327=ADVANCED_FACE ( 'NONE', ( #45250 ), #9271, .T. ) ;
#72329=CARTESIAN_POINT ( 'NONE',  ( 152.4536156746142410, 129.7208004331680797, -12.50000000000000000 ) ) ;
#72331=CARTESIAN_POINT ( 'NONE',  ( 199.0061125298537377, 276.0000000000000568, -7.725424859374024678 ) ) ;
#72338=CARTESIAN_POINT ( 'NONE',  ( 197.1983186874051341, 40.91381848194614435, 12.13059964849341021 ) ) ;
#72343=( BOUNDED_SURFACE ( )  B_SPLINE_SURFACE ( 3, 2, ( 
 ( #37391, #16553, #9432 ),
 ( #36944, #30772, #44497 ),
 ( #17019, #73402, #15167 ),
 ( #66300, #30301, #2364 ) ),
 .UNSPECIFIED., .F., .F., .F. ) 
 B_SPLINE_SURFACE_WITH_KNOTS ( ( 4, 4 ),
 ( 3, 3 ),
 ( 1.570796326794896558, 2.004620063563922638 ),
 ( 0.000000000000000000, 1.000000000000000000 ),
 .UNSPECIFIED. ) 
 GEOMETRIC_REPRESENTATION_ITEM ( )  RATIONAL_B_SPLINE_SURFACE ( (
 ( 1.000000000000000000, 0.7071067811865475727, 1.000000000000000000),
 ( 1.000000000000000000, 0.7478056585118711963, 1.000000000000000000),
 ( 1.000000000000000000, 0.7849082635113622253, 1.000000000000000000),
 ( 1.000000000000000000, 0.8168508380123946644, 1.000000000000000000) ) ) 
 REPRESENTATION_ITEM ( '' )  SURFACE ( )  );
#72351=( BOUNDED_CURVE ( )  B_SPLINE_CURVE ( 3, ( #77849, #33817, #27180, #12998 ),
 .UNSPECIFIED., .F., .F. ) 
 B_SPLINE_CURVE_WITH_KNOTS ( ( 4, 4 ),
 ( 4.712388980384689674, 6.283185307179586232 ),
 .UNSPECIFIED. ) 
 CURVE ( )  GEOMETRIC_REPRESENTATION_ITEM ( )  RATIONAL_B_SPLINE_CURVE ( ( 1.000000000000000000, 0.8047378541243649375, 0.8047378541243649375, 1.000000000000000000 ) ) 
 REPRESENTATION_ITEM ( '' )  );
#72356=ORIENTED_EDGE ( 'NONE', *, *, #84148, .T. ) ;
#72357=CARTESIAN_POINT ( 'NONE',  ( 197.2510236111309609, 71.96844395090404589, 11.91691450877446279 ) ) ;
#72359=CARTESIAN_POINT ( 'NONE',  ( 140.6539576904058606, 275.0000000000000568, -10.49999999999999822 ) ) ;
#72370=CARTESIAN_POINT ( 'NONE',  ( 195.0647618973419242, 40.86965449270967099, 13.52197506507135571 ) ) ;
#72382=DIRECTION ( 'NONE',  ( -1.000000000000000000, 0.000000000000000000, 0.000000000000000000 ) ) ;
#72383=DIRECTION ( 'NONE',  ( 0.000000000000000000, 1.000000000000000000, 0.000000000000000000 ) ) ;
#72387=ORIENTED_EDGE ( 'NONE', *, *, #39617, .T. ) ;
#72394=ORIENTED_EDGE ( 'NONE', *, *, #56360, .F. ) ;
#72403=CARTESIAN_POINT ( 'NONE',  ( 164.2231345125756263, 300.2961574867697436, 4.888549259831427740 ) ) ;
#72419=ORIENTED_EDGE ( 'NONE', *, *, #19910, .T. ) ;
#72420=ORIENTED_EDGE ( 'NONE', *, *, #65268, .T. ) ;
#72435=FACE_OUTER_BOUND ( 'NONE', #25061, .T. ) ;
#72446=CARTESIAN_POINT ( 'NONE',  ( 200.3424981856614693, 61.71662552184319139, 9.000000000000000000 ) ) ;
#72454=PLANE ( 'NONE',  #45389 ) ;
#72456=ADVANCED_FACE ( 'NONE', ( #2203 ), #76158, .T. ) ;
#72467=AXIS2_PLACEMENT_3D ( 'NONE', #15844, #9650, #31902 ) ;
#72469=ORIENTED_EDGE ( 'NONE', *, *, #30878, .T. ) ;
#72485=CARTESIAN_POINT ( 'NONE',  ( 154.7659666677267865, 20.47222690886501439, 12.53936336329526391 ) ) ;
#72496=ORIENTED_EDGE ( 'NONE', *, *, #52934, .T. ) ;
#72510=CARTESIAN_POINT ( 'NONE',  ( 153.2628468892384603, 20.37991841447902175, -11.93555113919331134 ) ) ;
#72522=VERTEX_POINT ( 'NONE', #44340 ) ;
#72523=CARTESIAN_POINT ( 'NONE',  ( 196.0517256323039135, 25.50333437355849142, 11.93519303445567736 ) ) ;
#72528=VECTOR ( 'NONE', #30390, 1000.000000000000000 ) ;
#72549=DIRECTION ( 'NONE',  ( 0.000000000000000000, 0.000000000000000000, 1.000000000000000000 ) ) ;
#72555=CARTESIAN_POINT ( 'NONE',  ( 151.4851178187871312, 15.00000000000000000, 0.000000000000000000 ) ) ;
#72560=CARTESIAN_POINT ( 'NONE',  ( 154.1407330040854333, 249.5000000000000568, -13.42592592592592915 ) ) ;
#72561=CARTESIAN_POINT ( 'NONE',  ( 197.3748232817349049, 275.0000000000000568, -12.45182892472559821 ) ) ;
#72571=ORIENTED_EDGE ( 'NONE', *, *, #68134, .T. ) ;
#72588=CARTESIAN_POINT ( 'NONE',  ( 153.5041831715941782, 19.57420759269780319, 11.76949543550875354 ) ) ;
#72590=AXIS2_PLACEMENT_3D ( 'NONE', #25163, #62087, #68728 ) ;
#72592=DIRECTION ( 'NONE',  ( 0.000000000000000000, -1.000000000000000000, -0.000000000000000000 ) ) ;
#72608=ORIENTED_EDGE ( 'NONE', *, *, #44755, .F. ) ;
#72611=ORIENTED_EDGE ( 'NONE', *, *, #67910, .F. ) ;
#72625=ADVANCED_FACE ( 'NONE', ( #83111 ), #75364, .F. ) ;
#72628=EDGE_CURVE ( 'NONE', #36747, #59112, #52408, .T. ) ;
#72630=ORIENTED_EDGE ( 'NONE', *, *, #24839, .T. ) ;
#72637=ORIENTED_EDGE ( 'NONE', *, *, #23802, .T. ) ;
#72640=VERTEX_POINT ( 'NONE', #19200 ) ;
#72649=CARTESIAN_POINT ( 'NONE',  ( 199.4565688755349981, 40.19734553069211103, 10.50000000000000888 ) ) ;
#72654=DIRECTION ( 'NONE',  ( 0.000000000000000000, 1.000000000000000000, 0.000000000000000000 ) ) ;
#72662=CARTESIAN_POINT ( 'NONE',  ( 154.4590814691937624, 20.78850955392830357, 13.92316269558947539 ) ) ;
#72666=CARTESIAN_POINT ( 'NONE',  ( 196.8803347170859865, 73.40565171261609123, 12.49999999999999289 ) ) ;
#72685=CARTESIAN_POINT ( 'NONE',  ( 209.8616357346608936, 36.89613957940315458, 12.09245862095555779 ) ) ;
#72724=DIRECTION ( 'NONE',  ( 0.000000000000000000, 1.000000000000000000, 0.000000000000000000 ) ) ;
#72727=AXIS2_PLACEMENT_3D ( 'NONE', #21942, #7713, #8634 ) ;
#72740=ORIENTED_EDGE ( 'NONE', *, *, #40929, .F. ) ;
#72741=CARTESIAN_POINT ( 'NONE',  ( 175.2296996224749250, 275.0000000000000568, -24.99999999999999289 ) ) ;
#72747=DIRECTION ( 'NONE',  ( 0.000000000000000000, 1.000000000000000000, 0.000000000000000000 ) ) ;
#72748=LINE ( 'NONE', #65679, #56238 ) ;
#72750=VERTEX_POINT ( 'NONE', #32482 ) ;
#72753=ORIENTED_EDGE ( 'NONE', *, *, #23679, .F. ) ;
#72768=DIRECTION ( 'NONE',  ( -0.7957555401921980742, -0.6056179655966482667, 0.000000000000000000 ) ) ;
#72781=CARTESIAN_POINT ( 'NONE',  ( 200.4644824113734671, 250.5000000000000568, -2.942835885954290021 ) ) ;
#72783=LINE ( 'NONE', #7908, #91363 ) ;
#72787=VECTOR ( 'NONE', #15062, 1000.000000000000000 ) ;
#72793=CARTESIAN_POINT ( 'NONE',  ( 153.6987871352777404, 19.48326534539592458, 11.45812909364015297 ) ) ;
#72806=ORIENTED_EDGE ( 'NONE', *, *, #15662, .F. ) ;
#72807=CARTESIAN_POINT ( 'NONE',  ( 154.9842916688209868, 275.0000000000000568, -12.88888888888890882 ) ) ;
#72820=CARTESIAN_POINT ( 'NONE',  ( 196.1981356858130425, 40.87848184507377880, 13.11514447343857981 ) ) ;
#72851=EDGE_CURVE ( 'NONE', #26459, #91019, #41319, .T. ) ;
#72854=TOROIDAL_SURFACE ( 'NONE', #53172, 4.499999999999990230, 0.5000000000000000000 ) ;
#72856=AXIS2_PLACEMENT_3D ( 'NONE', #9524, #73016, #8599 ) ;
#72866=AXIS2_PLACEMENT_3D ( 'NONE', #63852, #42491, #21667 ) ;
#72869=ORIENTED_EDGE ( 'NONE', *, *, #68018, .F. ) ;
#72919=EDGE_CURVE ( 'NONE', #75628, #84462, #44374, .T. ) ;
#72922=CIRCLE ( 'NONE', #86480, 7.500000000000013323 ) ;
#72923=ORIENTED_EDGE ( 'NONE', *, *, #57669, .F. ) ;
#72927=DIRECTION ( 'NONE',  ( -0.000000000000000000, -0.000000000000000000, -1.000000000000000000 ) ) ;
#72930=CIRCLE ( 'NONE', #85009, 0.5000000000000048850 ) ;
#72932=AXIS2_PLACEMENT_3D ( 'NONE', #45498, #18049, #53084 ) ;
#72939=ORIENTED_EDGE ( 'NONE', *, *, #41688, .F. ) ;
#72943=CARTESIAN_POINT ( 'NONE',  ( 189.4188515237862589, 293.9636489450775798, 13.99999999999999112 ) ) ;
#72944=EDGE_CURVE ( 'NONE', #26361, #76874, #28650, .T. ) ;
#72959=EDGE_CURVE ( 'NONE', #26750, #14772, #28193, .T. ) ;
#72969=CARTESIAN_POINT ( 'NONE',  ( 197.2116943569230330, 275.5000000000000568, -12.92446933126074882 ) ) ;
#72982=CARTESIAN_POINT ( 'NONE',  ( 194.7771416239231996, 25.43510842100042169, 13.92549921621965936 ) ) ;
#73000=AXIS2_PLACEMENT_3D ( 'NONE', #54962, #12842, #49271 ) ;
#73003=ORIENTED_EDGE ( 'NONE', *, *, #78211, .T. ) ;
#73010=CARTESIAN_POINT ( 'NONE',  ( 154.9842916688210153, 275.0000000000000568, 12.88888888888891593 ) ) ;
#73016=DIRECTION ( 'NONE',  ( 1.000000000000000000, 0.000000000000000000, -0.000000000000000000 ) ) ;
#73019=CARTESIAN_POINT ( 'NONE',  ( 199.7107580773175073, 25.46274433093360301, 10.17758690952041256 ) ) ;
#73022=CARTESIAN_POINT ( 'NONE',  ( 195.1858027385590049, 26.47779181510070146, 15.05860297072264231 ) ) ;
#73031=EDGE_CURVE ( 'NONE', #82490, #69835, #35756, .T. ) ;
#73037=CARTESIAN_POINT ( 'NONE',  ( 197.7051530045995094, 41.80213891112347824, 12.00000000000000000 ) ) ;
#73049=AXIS2_PLACEMENT_3D ( 'NONE', #62901, #48177, #91738 ) ;
#73051=FACE_OUTER_BOUND ( 'NONE', #19065, .T. ) ;
#73054=CARTESIAN_POINT ( 'NONE',  ( 208.6208076322478746, 32.98517505407394168, 14.26380412667038655 ) ) ;
#73066=TOROIDAL_SURFACE ( 'NONE', #15612, 1.000000000000000000, 0.5000000000000000000 ) ;
#73074=ORIENTED_EDGE ( 'NONE', *, *, #16074, .T. ) ;
#73076=CIRCLE ( 'NONE', #85165, 1.000000000000000888 ) ;
#73087=VECTOR ( 'NONE', #3137, 1000.000000000000000 ) ;
#73101=EDGE_CURVE ( 'NONE', #45666, #33195, #59545, .T. ) ;
#73104=ORIENTED_EDGE ( 'NONE', *, *, #38171, .F. ) ;
#73108=ORIENTED_EDGE ( 'NONE', *, *, #63351, .F. ) ;
#73122=DIRECTION ( 'NONE',  ( 1.000000000000000000, 0.000000000000000000, 0.000000000000000000 ) ) ;
#73129=DIRECTION ( 'NONE',  ( -1.000000000000000000, -0.000000000000000000, -0.000000000000000000 ) ) ;
#73136=CARTESIAN_POINT ( 'NONE',  ( 155.3967522965721173, 18.12362412296635128, -8.741384835540280562 ) ) ;
#73142=CARTESIAN_POINT ( 'NONE',  ( 180.2294467949672878, 214.9970011440365454, -24.94063848305471609 ) ) ;
#73146=CIRCLE ( 'NONE', #61056, 2.842139515347646750 ) ;
#73147=CIRCLE ( 'NONE', #20366, 2.999999999999997780 ) ;
#73152=AXIS2_PLACEMENT_3D ( 'NONE', #42004, #70918, #20722 ) ;
#73159=ADVANCED_FACE ( 'NONE', ( #5480 ), #64669, .F. ) ;
#73161=VERTEX_POINT ( 'NONE', #21072 ) ;
#73162=EDGE_CURVE ( 'NONE', #52528, #80622, #93497, .T. ) ;
#73166=AXIS2_PLACEMENT_3D ( 'NONE', #10724, #4565, #32529 ) ;
#73200=CARTESIAN_POINT ( 'NONE',  ( 161.2244399300530233, 8.542400036368780647, 10.00000000000000000 ) ) ;
#73201=AXIS2_PLACEMENT_3D ( 'NONE', #11140, #4981, #75542 ) ;
#73209=CIRCLE ( 'NONE', #27867, 25.00000000000000355 ) ;
#73219=ORIENTED_EDGE ( 'NONE', *, *, #87889, .T. ) ;
#73221=VECTOR ( 'NONE', #37824, 1000.000000000000000 ) ;
#73222=VECTOR ( 'NONE', #66558, 1000.000000000000000 ) ;
#73224=EDGE_CURVE ( 'NONE', #1470, #41734, #28669, .T. ) ;
#73229=DIRECTION ( 'NONE',  ( 0.2456588035076310295, -0.9693563597868428694, 0.000000000000000000 ) ) ;
#73230=DIRECTION ( 'NONE',  ( -1.000000000000000000, 0.000000000000000000, 0.000000000000000000 ) ) ;
#73233=AXIS2_PLACEMENT_3D ( 'NONE', #53351, #75601, #12137 ) ;
#73236=ORIENTED_EDGE ( 'NONE', *, *, #18737, .F. ) ;
#73237=CARTESIAN_POINT ( 'NONE',  ( 196.2220355002111489, 24.40165861654593016, 11.64020769021003332 ) ) ;
#73250=EDGE_CURVE ( 'NONE', #14834, #83547, #49943, .T. ) ;
#73259=DIRECTION ( 'NONE',  ( -0.8435586647355767242, 0.000000000000000000, -0.5370370370370473045 ) ) ;
#73260=DIRECTION ( 'NONE',  ( 0.000000000000000000, 0.000000000000000000, -1.000000000000000000 ) ) ;
#73265=CARTESIAN_POINT ( 'NONE',  ( 170.7304434856092143, 250.0000000000000568, -24.91818181818181088 ) ) ;
#73267=CARTESIAN_POINT ( 'NONE',  ( 153.9133111279453203, 20.47222690886559704, 13.06183683676577267 ) ) ;
#73273=DIRECTION ( 'NONE',  ( 0.000000000000000000, 0.000000000000000000, 1.000000000000000000 ) ) ;
#73290=EDGE_LOOP ( 'NONE', ( #5200, #50243, #6624, #30403 ) ) ;
#73291=CARTESIAN_POINT ( 'NONE',  ( 198.1232845152093205, 70.21759135774367167, 10.41992497367912662 ) ) ;
#73303=ORIENTED_EDGE ( 'NONE', *, *, #16325, .F. ) ;
#73318=ORIENTED_EDGE ( 'NONE', *, *, #11195, .F. ) ;
#73344=CARTESIAN_POINT ( 'NONE',  ( 198.5844002719293258, 69.20872177009273685, -9.718513320358827201 ) ) ;
#73349=ORIENTED_EDGE ( 'NONE', *, *, #28796, .F. ) ;
#73350=CARTESIAN_POINT ( 'NONE',  ( 196.3596534549891999, 42.20329003140924584, 13.36271651522391757 ) ) ;
#73363=CARTESIAN_POINT ( 'NONE',  ( 197.2116943569230898, 214.9331615741067765, -12.42446933126075592 ) ) ;
#73364=CARTESIAN_POINT ( 'NONE',  ( 199.4392256788250677, 65.82574266882504332, -7.741079165001071516 ) ) ;
#73366=AXIS2_PLACEMENT_3D ( 'NONE', #47684, #76585, #10765 ) ;
#73377=DIRECTION ( 'NONE',  ( -1.000000000000000000, 0.000000000000000000, 0.000000000000000000 ) ) ;
#73401=ORIENTED_EDGE ( 'NONE', *, *, #65309, .T. ) ;
#73402=CARTESIAN_POINT ( 'NONE',  ( 201.5895683925353694, 64.65149228630519929, -9.583120145142274282 ) ) ;
#73405=CARTESIAN_POINT ( 'NONE',  ( 0.000000000000000000, 3.000000000000000000, 9.000000000000001776 ) ) ;
#73414=ORIENTED_EDGE ( 'NONE', *, *, #11080, .T. ) ;
#73418=CARTESIAN_POINT ( 'NONE',  ( 196.3505989544111969, 71.51162351314616217, 11.47879840082592473 ) ) ;
#73421=CARTESIAN_POINT ( 'NONE',  ( 140.6539576904058606, 250.0000000000000568, -10.49999999999999822 ) ) ;
#73430=ORIENTED_EDGE ( 'NONE', *, *, #73993, .T. ) ;
#73437=ORIENTED_EDGE ( 'NONE', *, *, #53943, .F. ) ;
#73445=CARTESIAN_POINT ( 'NONE',  ( 151.4851178187871312, 20.00000000000000000, 10.00000000000000000 ) ) ;
#73473=VERTEX_POINT ( 'NONE', #230 ) ;
#73478=EDGE_CURVE ( 'NONE', #25873, #86239, #84604, .T. ) ;
#73481=CARTESIAN_POINT ( 'NONE',  ( 194.9270631639382430, 25.19695901056785914, 13.71261800098177730 ) ) ;
#73487=FACE_OUTER_BOUND ( 'NONE', #12424, .T. ) ;
#73489=VECTOR ( 'NONE', #59100, 1000.000000000000000 ) ;
#73490=CARTESIAN_POINT ( 'NONE',  ( 201.0876323342543799, 25.81167821795959938, 9.999999999999998224 ) ) ;
#73493=CARTESIAN_POINT ( 'NONE',  ( 195.4994389829729755, 25.60173194700487542, 14.63396631094618172 ) ) ;
#73494=DIRECTION ( 'NONE',  ( 1.000000000000000000, -0.000000000000000000, -0.000000000000000000 ) ) ;
#73506=FACE_OUTER_BOUND ( 'NONE', #70671, .T. ) ;
#73509=CARTESIAN_POINT ( 'NONE',  ( 193.5162140859150668, 249.5000000000000568, 17.51463615629763027 ) ) ;
#73522=DIRECTION ( 'NONE',  ( -0.000000000000000000, -1.000000000000000000, -0.000000000000000000 ) ) ;
#73562=VERTEX_POINT ( 'NONE', #72666 ) ;
#73569=ORIENTED_EDGE ( 'NONE', *, *, #76892, .T. ) ;
#73574=ORIENTED_EDGE ( 'NONE', *, *, #54065, .T. ) ;
#73584=CARTESIAN_POINT ( 'NONE',  ( 152.4536156746142410, 250.5000000000000568, -12.49999999999999289 ) ) ;
#73598=DIRECTION ( 'NONE',  ( -1.000000000000000000, 0.000000000000000000, 2.940294503956655304E-16 ) ) ;
#73600=DIRECTION ( 'NONE',  ( 0.000000000000000000, 1.000000000000000000, 0.000000000000000000 ) ) ;
#73602=CARTESIAN_POINT ( 'NONE',  ( 152.4536156746142410, 250.5000000000000568, -11.99999999999999289 ) ) ;
#73606=CARTESIAN_POINT ( 'NONE',  ( 180.2296971224742776, 215.0000000000000568, -25.00500000000002387 ) ) ;
#73619=CARTESIAN_POINT ( 'NONE',  ( 209.8616357346608652, 36.89613957940318301, 12.90102856104451767 ) ) ;
#73622=CARTESIAN_POINT ( 'NONE',  ( 175.2296996224750103, 250.0000000000000568, 0.000000000000000000 ) ) ;
#73637=ADVANCED_FACE ( 'NONE', ( #74512 ), #24119, .F. ) ;
#73641=CARTESIAN_POINT ( 'NONE',  ( 169.8384340989974817, 275.0000000000000568, -24.41176470588234437 ) ) ;
#73675=ORIENTED_EDGE ( 'NONE', *, *, #31692, .F. ) ;
#73676=CARTESIAN_POINT ( 'NONE',  ( 170.7304434856092143, 275.5000000000000568, -24.91818181818181088 ) ) ;
#73681=EDGE_CURVE ( 'NONE', #93112, #34264, #1763, .T. ) ;
#73683=DIRECTION ( 'NONE',  ( -1.000000000000000000, 0.000000000000000000, 0.000000000000000000 ) ) ;
#73688=ORIENTED_EDGE ( 'NONE', *, *, #88205, .T. ) ;
#73689=DIRECTION ( 'NONE',  ( 0.4988042400434494761, -0.06911816301596634959, -0.8639542867860402486 ) ) ;
#73694=EDGE_CURVE ( 'NONE', #39232, #49322, #34744, .T. ) ;
#73712=FACE_OUTER_BOUND ( 'NONE', #75473, .T. ) ;
#73720=DIRECTION ( 'NONE',  ( 0.000000000000000000, 0.000000000000000000, 1.000000000000000000 ) ) ;
#73743=CARTESIAN_POINT ( 'NONE',  ( 199.5543596254793499, 67.40697023589044079, 8.432225012702247113 ) ) ;
#73770=ORIENTED_EDGE ( 'NONE', *, *, #48476, .T. ) ;
#73794=EDGE_CURVE ( 'NONE', #22798, #90280, #90938, .T. ) ;
#73796=EDGE_CURVE ( 'NONE', #68989, #14859, #17309, .T. ) ;
#73797=CYLINDRICAL_SURFACE ( 'NONE', #12573, 9.103929867429224387 ) ;
#73803=CARTESIAN_POINT ( 'NONE',  ( 196.6739207415263593, 42.33397377253083960, 12.85244989408970184 ) ) ;
#73809=AXIS2_PLACEMENT_3D ( 'NONE', #91895, #5294, #32754 ) ;
#73818=CARTESIAN_POINT ( 'NONE',  ( 210.3152560301384142, 38.32590481451376263, 10.50000000000000000 ) ) ;
#73826=CARTESIAN_POINT ( 'NONE',  ( 154.0331653244526819, 19.37068896744924018, 11.96806464917981216 ) ) ;
#73831=FACE_OUTER_BOUND ( 'NONE', #55142, .T. ) ;
#73841=CARTESIAN_POINT ( 'NONE',  ( 164.2231345125756263, 264.6571197653884155, 7.500000000000000000 ) ) ;
#73850=VERTEX_POINT ( 'NONE', #22460 ) ;
#73851=CARTESIAN_POINT ( 'NONE',  ( 175.2296996224750103, 128.0000000000000568, 0.000000000000000000 ) ) ;
#73854=DIRECTION ( 'NONE',  ( -0.000000000000000000, -0.000000000000000000, 1.000000000000000000 ) ) ;
#73863=ORIENTED_EDGE ( 'NONE', *, *, #2023, .F. ) ;
#73867=CARTESIAN_POINT ( 'NONE',  ( 221.8344101925596306, 1.000000000000000222, -7.000000000000000888 ) ) ;
#73869=AXIS2_PLACEMENT_3D ( 'NONE', #57085, #233, #28654 ) ;
#73871=CARTESIAN_POINT ( 'NONE',  ( 154.9842916688209868, 128.0000000000000568, -12.88888888888889461 ) ) ;
#73884=EDGE_CURVE ( 'NONE', #31000, #16833, #51334, .T. ) ;
#73894=CARTESIAN_POINT ( 'NONE',  ( 164.7123623445222904, 3.000000000000000000, 10.00000000000000178 ) ) ;
#73906=EDGE_LOOP ( 'NONE', ( #77019, #49772, #55852 ) ) ;
#73907=CARTESIAN_POINT ( 'NONE',  ( 194.7211398848818362, 27.16984437419170462, 14.02118807791477018 ) ) ;
#73926=CARTESIAN_POINT ( 'NONE',  ( 157.7238125175282448, 18.72892514816167164, 11.10081581328679867 ) ) ;
#73928=CIRCLE ( 'NONE', #33110, 1.000000000000000888 ) ;
#73929=CARTESIAN_POINT ( 'NONE',  ( 194.2991783531507508, 27.07972378075054465, 14.57245942894549096 ) ) ;
#73934=EDGE_CURVE ( 'NONE', #47807, #17649, #60330, .T. ) ;
#73936=DIRECTION ( 'NONE',  ( 0.000000000000000000, 0.000000000000000000, 1.000000000000000000 ) ) ;
#73938=CARTESIAN_POINT ( 'NONE',  ( 201.0876323342543515, 25.81167821795959938, 10.49999999999999822 ) ) ;
#73942=CARTESIAN_POINT ( 'NONE',  ( 221.8344101925596021, 1.000000000000000222, -8.171572875253810153 ) ) ;
#73952=CARTESIAN_POINT ( 'NONE',  ( 154.1407330040854333, 128.0000000000000568, 13.42592592592592737 ) ) ;
#73955=FACE_OUTER_BOUND ( 'NONE', #5072, .T. ) ;
#73968=CARTESIAN_POINT ( 'NONE',  ( 158.5846220834750397, 17.31716537717085203, 10.56280983457213907 ) ) ;
#73971=LINE ( 'NONE', #38448, #53033 ) ;
#73985=VERTEX_POINT ( 'NONE', #8259 ) ;
#73993=EDGE_CURVE ( 'NONE', #14152, #35152, #87642, .T. ) ;
#73996=CIRCLE ( 'NONE', #16549, 4.003189038634634045 ) ;
#74009=ORIENTED_EDGE ( 'NONE', *, *, #65011, .T. ) ;
#74020=EDGE_CURVE ( 'NONE', #76130, #44950, #67990, .T. ) ;
#74021=VERTEX_POINT ( 'NONE', #66048 ) ;
#74044=CARTESIAN_POINT ( 'NONE',  ( 175.2296996224750103, 20.99999999999998934, 24.00000000000000355 ) ) ;
#74047=CARTESIAN_POINT ( 'NONE',  ( 152.4536156746142410, 250.0000000000000568, 14.50000000000000000 ) ) ;
#74049=DIRECTION ( 'NONE',  ( -0.000000000000000000, -0.000000000000000000, -1.000000000000000000 ) ) ;
#74064=EDGE_LOOP ( 'NONE', ( #71945, #41972, #49335, #35367 ) ) ;
#74072=DIRECTION ( 'NONE',  ( 0.000000000000000000, 1.000000000000000000, 0.000000000000000000 ) ) ;
#74086=EDGE_CURVE ( 'NONE', #86133, #66468, #58924, .T. ) ;
#74102=ORIENTED_EDGE ( 'NONE', *, *, #41537, .F. ) ;
#74108=EDGE_CURVE ( 'NONE', #40624, #74338, #27174, .T. ) ;
#74111=CARTESIAN_POINT ( 'NONE',  ( 201.2104617360081704, 60.19600395700749829, 7.000000000000000000 ) ) ;
#74124=EDGE_LOOP ( 'NONE', ( #84131, #75390, #89821, #46553, #4105, #20680 ) ) ;
#74127=EDGE_CURVE ( 'NONE', #34178, #44986, #69521, .T. ) ;
#74134=DIRECTION ( 'NONE',  ( -1.000000000000000000, 0.000000000000000000, -0.000000000000000000 ) ) ;
#74135=FACE_OUTER_BOUND ( 'NONE', #14883, .T. ) ;
#74141=CARTESIAN_POINT ( 'NONE',  ( 197.9931848602547007, 41.98013133710430367, 9.866139269262600209 ) ) ;
#74144=ADVANCED_FACE ( 'NONE', ( #75913 ), #17699, .F. ) ;
#74155=CARTESIAN_POINT ( 'NONE',  ( 185.4166944662832179, 250.5000000000000568, 23.37680765314684450 ) ) ;
#74164=CARTESIAN_POINT ( 'NONE',  ( 219.8344101925596021, 3.000000000000000000, -10.00000000000000000 ) ) ;
#74165=CARTESIAN_POINT ( 'NONE',  ( 164.2231345125756263, 291.1800221208779931, -7.499999999999996447 ) ) ;
#74173=DIRECTION ( 'NONE',  ( -0.000000000000000000, -1.000000000000000000, -0.000000000000000000 ) ) ;
#74183=CARTESIAN_POINT ( 'NONE',  ( 189.9243309297870610, 249.5000000000000568, 20.22542485937349355 ) ) ;
#74198=CARTESIAN_POINT ( 'NONE',  ( 154.1415209985679269, 20.37991841447902175, 11.45812909362559040 ) ) ;
#74200=DIRECTION ( 'NONE',  ( 0.000000000000000000, 1.000000000000000000, 0.000000000000000000 ) ) ;
#74210=ORIENTED_EDGE ( 'NONE', *, *, #12108, .T. ) ;
#74225=ORIENTED_EDGE ( 'NONE', *, *, #81096, .T. ) ;
#74243=CARTESIAN_POINT ( 'NONE',  ( 207.4345711710209343, 35.56792554197559042, 12.00000000000000000 ) ) ;
#74251=CARTESIAN_POINT ( 'NONE',  ( 139.1539576904058606, 250.0000000000000568, 10.50000000000000000 ) ) ;
#74257=CARTESIAN_POINT ( 'NONE',  ( 200.6868442215943844, 15.43634792868608940, -10.00000000000000355 ) ) ;
#74260=EDGE_CURVE ( 'NONE', #15778, #92724, #54135, .T. ) ;
#74271=CARTESIAN_POINT ( 'NONE',  ( 184.7149167944524493, 8.542400036368780647, 25.74970488511327815 ) ) ;
#74280=CARTESIAN_POINT ( 'NONE',  ( 199.0061125298537377, 250.5000000000000568, -7.725424859374024678 ) ) ;
#74307=DIRECTION ( 'NONE',  ( 0.000000000000000000, 0.000000000000000000, 1.000000000000000000 ) ) ;
#74310=LINE ( 'NONE', #73405, #70058 ) ;
#74314=EDGE_CURVE ( 'NONE', #70030, #13153, #74998, .T. ) ;
#74324=CARTESIAN_POINT ( 'NONE',  ( 159.6810783670777880, 8.542400036368780647, -9.000000000000001776 ) ) ;
#74338=VERTEX_POINT ( 'NONE', #76856 ) ;
#74346=ORIENTED_EDGE ( 'NONE', *, *, #57468, .T. ) ;
#74354=DIRECTION ( 'NONE',  ( 0.5370370370370571855, -0.000000000000000000, 0.8435586647355706180 ) ) ;
#74366=CARTESIAN_POINT ( 'NONE',  ( 194.2870706637142177, 27.48493576247232539, 14.58823529411773734 ) ) ;
#74384=CARTESIAN_POINT ( 'NONE',  ( 184.7149167944524493, 8.542400036368780647, -9.000000000000001776 ) ) ;
#74386=CARTESIAN_POINT ( 'NONE',  ( 200.4551663813218170, 64.49084098419280053, 0.000000000000000000 ) ) ;
#74387=CIRCLE ( 'NONE', #23022, 25.00000000000000355 ) ;
#74395=VECTOR ( 'NONE', #34135, 1000.000000000000000 ) ;
#74397=CARTESIAN_POINT ( 'NONE',  ( 200.5094052070897419, 25.16710152838790293, 9.999999999999998224 ) ) ;
#74400=CARTESIAN_POINT ( 'NONE',  ( 197.4836817735085219, 42.27872732282709478, 11.66666666666667140 ) ) ;
#74410=ORIENTED_EDGE ( 'NONE', *, *, #15525, .T. ) ;
#74427=CARTESIAN_POINT ( 'NONE',  ( 159.4851178187817879, 15.24064981607338432, 10.00000000000000178 ) ) ;
#74430=FACE_OUTER_BOUND ( 'NONE', #35363, .T. ) ;
#74444=ORIENTED_EDGE ( 'NONE', *, *, #43842, .T. ) ;
#74466=AXIS2_PLACEMENT_3D ( 'NONE', #43486, #43030, #72382 ) ;
#74471=ORIENTED_EDGE ( 'NONE', *, *, #53345, .T. ) ;
#74484=ORIENTED_EDGE ( 'NONE', *, *, #23802, .F. ) ;
#74499=CIRCLE ( 'NONE', #32190, 24.49999999999999645 ) ;
#74508=DIRECTION ( 'NONE',  ( 0.6522365350567651543, -0.2069344830099842103, -0.7292226148979034095 ) ) ;
#74509=CARTESIAN_POINT ( 'NONE',  ( 193.9646936176698375, 19.99999999999999645, 15.00000000000039080 ) ) ;
#74512=FACE_OUTER_BOUND ( 'NONE', #53655, .T. ) ;
#74519=DIRECTION ( 'NONE',  ( 0.000000000000000000, 0.000000000000000000, 1.000000000000000000 ) ) ;
#74527=ADVANCED_FACE ( 'NONE', ( #33290 ), #83465, .T. ) ;
#74529=AXIS2_PLACEMENT_3D ( 'NONE', #41891, #35752, #5937 ) ;
#74531=ORIENTED_EDGE ( 'NONE', *, *, #23350, .T. ) ;
#74532=TOROIDAL_SURFACE ( 'NONE', #21620, 1.000000000000000000, 0.5000000000000000000 ) ;
#74536=FACE_OUTER_BOUND ( 'NONE', #87017, .T. ) ;
#74538=AXIS2_PLACEMENT_3D ( 'NONE', #46902, #61161, #61616 ) ;
#74540=CARTESIAN_POINT ( 'NONE',  ( 209.8744251295252354, 28.03846817292548366, 15.00000000000000000 ) ) ;
#74544=VECTOR ( 'NONE', #91536, 1000.000000000000000 ) ;
#74555=VECTOR ( 'NONE', #80885, 1000.000000000000000 ) ;
#74557=EDGE_CURVE ( 'NONE', #62353, #55580, #32830, .T. ) ;
#74562=AXIS2_PLACEMENT_3D ( 'NONE', #64895, #93262, #27959 ) ;
#74572=VECTOR ( 'NONE', #49745, 1000.000000000000000 ) ;
#74574=EDGE_LOOP ( 'NONE', ( #5627, #7486, #67637, #50765 ) ) ;
#74581=B_SPLINE_CURVE_WITH_KNOTS ( 'NONE', 3,
 ( #71893, #59055, #35886, #21679, #22143, #93627 ),
 .UNSPECIFIED., .F., .F.,
 ( 4, 2, 4 ),
 ( 0.002740393443096640798, 0.004110592855002227590, 0.005480792266907814382 ),
 .UNSPECIFIED. ) ;
#74592=ORIENTED_EDGE ( 'NONE', *, *, #42126, .F. ) ;
#74598=VERTEX_POINT ( 'NONE', #24797 ) ;
#74603=AXIS2_PLACEMENT_3D ( 'NONE', #53191, #88243, #8256 ) ;
#74608=CARTESIAN_POINT ( 'NONE',  ( 196.7679187601920034, 69.63253546436693853, -10.95639144170524837 ) ) ;
#74627=CIRCLE ( 'NONE', #67138, 24.00000000000001066 ) ;
#74630=CYLINDRICAL_SURFACE ( 'NONE', #29258, 3.000000000000000000 ) ;
#74632=AXIS2_PLACEMENT_3D ( 'NONE', #38201, #66189, #1306 ) ;
#74640=CARTESIAN_POINT ( 'NONE',  ( 175.2296996224749250, 250.5000000000000568, -24.99999999999999289 ) ) ;
#74646=CARTESIAN_POINT ( 'NONE',  ( 169.8384340989974532, 214.5000000000000568, -24.41176470588233727 ) ) ;
#74648=EDGE_CURVE ( 'NONE', #27540, #89945, #76395, .T. ) ;
#74654=VECTOR ( 'NONE', #28282, 1000.000000000000000 ) ;
#74672=EDGE_CURVE ( 'NONE', #17168, #10872, #4881, .T. ) ;
#74678=DIRECTION ( 'NONE',  ( -1.000000000000000000, -0.000000000000000000, -0.000000000000000000 ) ) ;
#74684=CIRCLE ( 'NONE', #32373, 4.499999999999990230 ) ;
#74688=ORIENTED_EDGE ( 'NONE', *, *, #742, .F. ) ;
#74693=AXIS2_PLACEMENT_3D ( 'NONE', #39147, #62363, #5066 ) ;
#74702=CARTESIAN_POINT ( 'NONE',  ( 202.9738562182569694, 293.9636489450776367, -59.00000000000003553 ) ) ;
#74714=CIRCLE ( 'NONE', #6737, 2.500000000000002220 ) ;
#74720=DIRECTION ( 'NONE',  ( 0.9998346970812742596, 0.000000000000000000, 0.01818181818181330636 ) ) ;
#74724=CARTESIAN_POINT ( 'NONE',  ( 208.4306832106271088, 0.04196010845015910040, -7.500000000000013323 ) ) ;
#74735=ORIENTED_EDGE ( 'NONE', *, *, #55276, .F. ) ;
#74736=VERTEX_POINT ( 'NONE', #55079 ) ;
#74737=CARTESIAN_POINT ( 'NONE',  ( 195.1441566087187311, 40.16915684026574951, 15.11344275051338748 ) ) ;
#74754=AXIS2_PLACEMENT_3D ( 'NONE', #40146, #76160, #41068 ) ;
#74762=FACE_OUTER_BOUND ( 'NONE', #40367, .T. ) ;
#74764=VECTOR ( 'NONE', #59527, 1000.000000000000000 ) ;
#74766=TOROIDAL_SURFACE ( 'NONE', #12807, 4.499999999999990230, 0.5000000000000000000 ) ;
#74773=VECTOR ( 'NONE', #24514, 1000.000000000000000 ) ;
#74782=CARTESIAN_POINT ( 'NONE',  ( 157.4851178187871312, 69.18068689461284748, -7.000000000000000888 ) ) ;
#74794=CARTESIAN_POINT ( 'NONE',  ( 219.8344101925596021, 35.72494958537217968, 7.000000000000000000 ) ) ;
#74804=ADVANCED_FACE ( 'NONE', ( #60790 ), #83948, .F. ) ;
#74806=EDGE_LOOP ( 'NONE', ( #37992, #56528, #23610, #81307, #85416, #39031, #82750 ) ) ;
#74809=DIRECTION ( 'NONE',  ( -0.000000000000000000, -1.000000000000000000, -0.000000000000000000 ) ) ;
#74810=EDGE_CURVE ( 'NONE', #35587, #67369, #93163, .T. ) ;
#74812=DIRECTION ( 'NONE',  ( -0.000000000000000000, -1.000000000000000000, -0.000000000000000000 ) ) ;
#74823=( BOUNDED_CURVE ( )  B_SPLINE_CURVE ( 3, ( #84666, #90814, #25515, #84203 ),
 .UNSPECIFIED., .F., .F. ) 
 B_SPLINE_CURVE_WITH_KNOTS ( ( 4, 4 ),
 ( 1.570796326794894560, 2.004620063563922638 ),
 .UNSPECIFIED. ) 
 CURVE ( )  GEOMETRIC_REPRESENTATION_ITEM ( )  RATIONAL_B_SPLINE_CURVE ( ( 1.000000000000000000, 0.9843778111405747655, 0.9843778111405747655, 1.000000000000000000 ) ) 
 REPRESENTATION_ITEM ( '' )  );
#74824=PRODUCT_DEFINITION ( 'UNKNOWN', '', #2384, #34327 ) ;
#74825=ORIENTED_EDGE ( 'NONE', *, *, #41751, .F. ) ;
#74828=( BOUNDED_CURVE ( )  B_SPLINE_CURVE ( 3, ( #13966, #72649, #65576, #58910 ),
 .UNSPECIFIED., .F., .F. ) 
 B_SPLINE_CURVE_WITH_KNOTS ( ( 4, 4 ),
 ( 1.570796326794902775, 2.411864997362830110 ),
 .UNSPECIFIED. ) 
 CURVE ( )  GEOMETRIC_REPRESENTATION_ITEM ( )  RATIONAL_B_SPLINE_CURVE ( ( 1.000000000000000000, 0.9419139527835183046, 0.9419139527835183046, 1.000000000000000000 ) ) 
 REPRESENTATION_ITEM ( '' )  );
#74835=ORIENTED_EDGE ( 'NONE', *, *, #37224, .T. ) ;
#74841=LINE ( 'NONE', #2407, #89939 ) ;
#74853=VERTEX_POINT ( 'NONE', #53682 ) ;
#74854=FACE_OUTER_BOUND ( 'NONE', #82232, .T. ) ;
#74877=DIRECTION ( 'NONE',  ( -0.000000000000000000, 0.000000000000000000, -1.000000000000000000 ) ) ;
#74886=CARTESIAN_POINT ( 'NONE',  ( 194.7272697301369533, 20.94006893973816119, -14.00764870559285136 ) ) ;
#74889=FACE_OUTER_BOUND ( 'NONE', #76913, .T. ) ;
#74890=DIRECTION ( 'NONE',  ( 0.000000000000000000, 0.000000000000000000, 1.000000000000000000 ) ) ;
#74899=VERTEX_POINT ( 'NONE', #57433 ) ;
#74916=CARTESIAN_POINT ( 'NONE',  ( 165.4265872613447641, 2.973978534295030229, 8.999830714574057922 ) ) ;
#74917=CARTESIAN_POINT ( 'NONE',  ( 222.8344101925596306, 35.72494958537217968, 7.000000000000000000 ) ) ;
#74943=CARTESIAN_POINT ( 'NONE',  ( 195.1051073005702960, 20.04979238141099174, -15.17562376660917067 ) ) ;
#74948=VERTEX_POINT ( 'NONE', #34705 ) ;
#74959=ORIENTED_EDGE ( 'NONE', *, *, #49120, .T. ) ;
#74966=ORIENTED_EDGE ( 'NONE', *, *, #90748, .F. ) ;
#74970=EDGE_LOOP ( 'NONE', ( #68882, #69720, #24398, #39963 ) ) ;
#74971=ORIENTED_EDGE ( 'NONE', *, *, #71679, .F. ) ;
#74986=AXIS2_PLACEMENT_3D ( 'NONE', #36748, #80769, #79398 ) ;
#74994=CARTESIAN_POINT ( 'NONE',  ( 184.7149167944524493, 8.542400036368780647, 9.000000000000001776 ) ) ;
#74995=DIRECTION ( 'NONE',  ( 0.6056179655966479336, -0.7957555401921982963, 0.000000000000000000 ) ) ;
#74998=LINE ( 'NONE', #11038, #83108 ) ;
#75017=DIRECTION ( 'NONE',  ( 0.000000000000000000, 0.000000000000000000, 1.000000000000000000 ) ) ;
#75020=FACE_OUTER_BOUND ( 'NONE', #89222, .T. ) ;
#75038=CARTESIAN_POINT ( 'NONE',  ( 207.4410801934303379, 29.85817334154656422, 14.41714557868295898 ) ) ;
#75048=AXIS2_PLACEMENT_3D ( 'NONE', #55373, #85638, #41605 ) ;
#75051=ORIENTED_EDGE ( 'NONE', *, *, #1761, .T. ) ;
#75053=VERTEX_POINT ( 'NONE', #63618 ) ;
#75072=EDGE_LOOP ( 'NONE', ( #17882, #9922, #28140, #25553 ) ) ;
#75074=EDGE_CURVE ( 'NONE', #30244, #13595, #81904, .T. ) ;
#75079=CARTESIAN_POINT ( 'NONE',  ( 184.7149167944524493, 8.542400036368780647, 25.74970488511327815 ) ) ;
#75080=EDGE_CURVE ( 'NONE', #24375, #610, #60431, .T. ) ;
#75086=DIRECTION ( 'NONE',  ( -0.5505044217881672752, 0.8348322475753291450, 0.000000000000000000 ) ) ;
#75088=ADVANCED_FACE ( 'NONE', ( #28088 ), #48419, .T. ) ;
#75115=DIRECTION ( 'NONE',  ( -1.000000000000000000, 0.000000000000000000, 0.000000000000000000 ) ) ;
#75118=DIRECTION ( 'NONE',  ( 0.000000000000000000, 0.000000000000000000, 1.000000000000000000 ) ) ;
#75142=ORIENTED_EDGE ( 'NONE', *, *, #51451, .T. ) ;
#75145=CARTESIAN_POINT ( 'NONE',  ( 203.6865049563636774, 300.2141583696141538, -4.993328456907190294 ) ) ;
#75164=CARTESIAN_POINT ( 'NONE',  ( 140.6539576904058606, 275.0000000000000568, 11.50000000000000000 ) ) ;
#75165=FACE_OUTER_BOUND ( 'NONE', #26599, .T. ) ;
#75178=ORIENTED_EDGE ( 'NONE', *, *, #6569, .T. ) ;
#75183=PLANE ( 'NONE',  #79454 ) ;
#75187=CARTESIAN_POINT ( 'NONE',  ( 196.1227023549103592, 250.0000000000000568, -11.81026827902096521 ) ) ;
#75188=CARTESIAN_POINT ( 'NONE',  ( 197.5461146819721137, 68.31320778628679591, 9.184551779176434394 ) ) ;
#75196=CYLINDRICAL_SURFACE ( 'NONE', #10990, 24.00000000000001066 ) ;
#75200=CARTESIAN_POINT ( 'NONE',  ( 195.1832308150864037, 40.36708659705613655, 15.06199699808708381 ) ) ;
#75217=CARTESIAN_POINT ( 'NONE',  ( 183.0442525570908288, 291.1800221208779931, 7.500000000000000000 ) ) ;
#75229=CARTESIAN_POINT ( 'NONE',  ( 179.7289557593406357, 275.5000000000000568, -24.91818181818184641 ) ) ;
#75231=DIRECTION ( 'NONE',  ( 0.000000000000000000, 1.000000000000000000, 0.000000000000000000 ) ) ;
#75240=DIRECTION ( 'NONE',  ( 0.000000000000000000, 1.000000000000000000, 0.000000000000000000 ) ) ;
#75262=ORIENTED_EDGE ( 'NONE', *, *, #13973, .F. ) ;
#75267=ADVANCED_FACE ( 'NONE', ( #93389 ), #27606, .T. ) ;
#75269=CARTESIAN_POINT ( 'NONE',  ( 157.1811212665062101, 275.9651295423822717, 16.89756555088535350 ) ) ;
#75288=ORIENTED_EDGE ( 'NONE', *, *, #58215, .T. ) ;
#75289=ORIENTED_EDGE ( 'NONE', *, *, #76892, .F. ) ;
#75290=VECTOR ( 'NONE', #62810, 1000.000000000000000 ) ;
#75291=DIRECTION ( 'NONE',  ( 0.000000000000000000, 0.000000000000000000, -1.000000000000000000 ) ) ;
#75296=CARTESIAN_POINT ( 'NONE',  ( 202.8019728163925492, 61.40723988820079171, 7.000000000000000000 ) ) ;
#75307=VERTEX_POINT ( 'NONE', #11357 ) ;
#75308=CARTESIAN_POINT ( 'NONE',  ( 194.7373591563044783, 27.48493576247233250, 14.00000000000007461 ) ) ;
#75318=DIRECTION ( 'NONE',  ( 0.000000000000000000, 1.000000000000000000, 0.000000000000000000 ) ) ;
#75324=EDGE_CURVE ( 'NONE', #90952, #85642, #63565, .T. ) ;
#75328=EDGE_CURVE ( 'NONE', #84307, #65773, #70070, .T. ) ;
#75332=CARTESIAN_POINT ( 'NONE',  ( 210.6909600361163371, -5.082197683525803883E-17, 7.166288341785294058 ) ) ;
#75341=CARTESIAN_POINT ( 'NONE',  ( 197.4352353745718744, 215.0000000000000568, -12.47235818614446146 ) ) ;
#75344=FACE_OUTER_BOUND ( 'NONE', #33099, .T. ) ;
#75355=VERTEX_POINT ( 'NONE', #10410 ) ;
#75356=CARTESIAN_POINT ( 'NONE',  ( 216.5288609127277084, 293.9636489450776935, 13.99999999999999112 ) ) ;
#75359=CARTESIAN_POINT ( 'NONE',  ( 195.7122344542522399, 26.11845659094913685, 14.66853270682850940 ) ) ;
#75364=( BOUNDED_SURFACE ( )  B_SPLINE_SURFACE ( 3, 2, ( 
 ( #47115, #62295, #48530 ),
 ( #4065, #54241, #76500 ),
 ( #90660, #62789, #26303 ),
 ( #60896, #82652, #25820 ),
 ( #10680, #32000, #18739 ),
 ( #4997, #83576, #55198 ),
 ( #47598, #91624, #89745 ),
 ( #26777, #19662, #54700 ),
 ( #24906, #33396, #84053 ),
 ( #76964, #11624, #40470 ) ),
 .UNSPECIFIED., .F., .F., .F. ) 
 B_SPLINE_SURFACE_WITH_KNOTS ( ( 4, 2, 2, 2, 4 ),
 ( 3, 3 ),
 ( -2.168404344971008868E-19, 0.002513556688247616140, 0.005027113376495232280, 0.007540670064742848420, 0.01005422675299046456 ),
 ( 0.000000000000000000, 1.000000000000000000 ),
 .UNSPECIFIED. ) 
 GEOMETRIC_REPRESENTATION_ITEM ( )  RATIONAL_B_SPLINE_SURFACE ( (
 ( 1.000000000000000000, 0.8168508380123963297, 1.000000000000000000),
 ( 1.000000000000000000, 0.8469576315469661276, 1.000000000000000000),
 ( 1.000000000000000000, 0.8738409315860931059, 1.000000000000000000),
 ( 1.000000000000000000, 0.9200669567820307648, 1.000000000000000000),
 ( 1.000000000000000000, 0.9394145480633124823, 1.000000000000000000),
 ( 1.000000000000000000, 0.9701920524516296496, 1.000000000000000000),
 ( 1.000000000000000000, 0.9815163856011694943, 1.000000000000000000),
 ( 1.000000000000000000, 0.9964122006648195029, 1.000000000000000000),
 ( 1.000000000000000000, 1.000002041055502389, 1.000000000000000000),
 ( 1.000000000000000000, 1.000000000000000000, 1.000000000000000000) ) ) 
 REPRESENTATION_ITEM ( '' )  SURFACE ( )  );
#75370=( BOUNDED_CURVE ( )  B_SPLINE_CURVE ( 3, ( #88367, #24914, #23517, #53791 ),
 .UNSPECIFIED., .F., .F. ) 
 B_SPLINE_CURVE_WITH_KNOTS ( ( 4, 4 ),
 ( 4.712388980384689674, 6.283185307179586232 ),
 .UNSPECIFIED. ) 
 CURVE ( )  GEOMETRIC_REPRESENTATION_ITEM ( )  RATIONAL_B_SPLINE_CURVE ( ( 1.000000000000000000, 0.8047378541243649375, 0.8047378541243649375, 1.000000000000000000 ) ) 
 REPRESENTATION_ITEM ( '' )  );
#75375=CARTESIAN_POINT ( 'NONE',  ( 207.0561972617101674, 35.35788477359429294, 14.49999999999999822 ) ) ;
#75390=ORIENTED_EDGE ( 'NONE', *, *, #31774, .T. ) ;
#75392=VERTEX_POINT ( 'NONE', #40670 ) ;
#75398=B_SPLINE_CURVE_WITH_KNOTS ( 'NONE', 3,
 ( #81141, #2080, #36661, #58915, #58460, #16285, #87761, #57993, #86847, #66038 ),
 .UNSPECIFIED., .F., .F.,
 ( 4, 2, 2, 2, 4 ),
 ( 8.886119947416682612E-17, 0.0005219798220732356541, 0.001043959644146382404, 0.001565939466219529261, 0.002087919288292675903 ),
 .UNSPECIFIED. ) ;
#75409=CARTESIAN_POINT ( 'NONE',  ( 153.6987871352777404, 19.48326534539592458, 11.45812909364015297 ) ) ;
#75414=ORIENTED_EDGE ( 'NONE', *, *, #63294, .F. ) ;
#75422=CARTESIAN_POINT ( 'NONE',  ( 140.6539576904058606, 131.0000000000000568, -11.50000000000000000 ) ) ;
#75428=CIRCLE ( 'NONE', #34609, 8.550761578869359170 ) ;
#75438=DIRECTION ( 'NONE',  ( -0.01818181818181330636, 0.000000000000000000, 0.9998346970812744816 ) ) ;
#75442=FACE_OUTER_BOUND ( 'NONE', #10751, .T. ) ;
#75445=ADVANCED_FACE ( 'NONE', ( #47311 ), #13, .T. ) ;
#75448=CYLINDRICAL_SURFACE ( 'NONE', #86688, 0.5000000000000004441 ) ;
#75454=CARTESIAN_POINT ( 'NONE',  ( 158.5846220834750113, 17.31716537717171889, -10.56280983457258316 ) ) ;
#75468=ORIENTED_EDGE ( 'NONE', *, *, #56056, .T. ) ;
#75473=EDGE_LOOP ( 'NONE', ( #60265, #73219, #32073 ) ) ;
#75489=CIRCLE ( 'NONE', #34675, 3.000000000000002665 ) ;
#75491=DIRECTION ( 'NONE',  ( 0.000000000000000000, 0.000000000000000000, 1.000000000000000000 ) ) ;
#75497=EDGE_CURVE ( 'NONE', #55526, #83549, #18936, .T. ) ;
#75500=ADVANCED_FACE ( 'NONE', ( #39274 ), #24183, .F. ) ;
#75506=VERTEX_POINT ( 'NONE', #33132 ) ;
#75508=ORIENTED_EDGE ( 'NONE', *, *, #56743, .F. ) ;
#75532=ADVANCED_FACE ( 'NONE', ( #77162 ), #69126, .F. ) ;
#75536=CARTESIAN_POINT ( 'NONE',  ( 175.2296996224750103, 138.1603916158177583, 0.000000000000000000 ) ) ;
#75542=DIRECTION ( 'NONE',  ( 0.000000000000000000, 0.000000000000000000, 1.000000000000000000 ) ) ;
#75548=AXIS2_PLACEMENT_3D ( 'NONE', #85264, #48795, #50206 ) ;
#75551=CARTESIAN_POINT ( 'NONE',  ( 153.3221070565148807, 19.65277508768675574, -12.04734487801197140 ) ) ;
#75558=CARTESIAN_POINT ( 'NONE',  ( 198.4468466364687060, 24.69666864892464275, 10.58981561310753250 ) ) ;
#75566=CARTESIAN_POINT ( 'NONE',  ( 140.6539576904058606, 275.5000000000000568, 12.50000000000000000 ) ) ;
#75571=CARTESIAN_POINT ( 'NONE',  ( 201.0876323342543515, 25.81167821795958162, 10.49999999999999822 ) ) ;
#75601=DIRECTION ( 'NONE',  ( 0.000000000000000000, -1.000000000000000000, 0.000000000000000000 ) ) ;
#75605=ADVANCED_FACE ( 'NONE', ( #90397 ), #83181, .T. ) ;
#75612=ORIENTED_EDGE ( 'NONE', *, *, #88205, .F. ) ;
#75613=LINE ( 'NONE', #3175, #10793 ) ;
#75620=VECTOR ( 'NONE', #14602, 1000.000000000000000 ) ;
#75624=DIRECTION ( 'NONE',  ( -0.000000000000000000, 0.000000000000000000, -1.000000000000000000 ) ) ;
#75628=VERTEX_POINT ( 'NONE', #11819 ) ;
#75637=ORIENTED_EDGE ( 'NONE', *, *, #46981, .F. ) ;
#75645=DIRECTION ( 'NONE',  ( -0.000000000000000000, -1.000000000000000000, -0.000000000000000000 ) ) ;
#75654=DIRECTION ( 'NONE',  ( 0.000000000000000000, 0.000000000000000000, -1.000000000000000000 ) ) ;
#75672=CARTESIAN_POINT ( 'NONE',  ( 140.6539576904058606, 275.0000000000000568, 11.50000000000000000 ) ) ;
#75684=FACE_OUTER_BOUND ( 'NONE', #9721, .T. ) ;
#75686=CIRCLE ( 'NONE', #10655, 5.568361562975243650 ) ;
#75687=CARTESIAN_POINT ( 'NONE',  ( 160.5350683151633291, 249.5000000000000568, 20.22542485937379908 ) ) ;
#75691=TOROIDAL_SURFACE ( 'NONE', #62110, 4.500000000000002665, 0.5000000000000000000 ) ;
#75694=DIRECTION ( 'NONE',  ( 0.9531768234071980039, -0.3024135303179465994, -1.750957418710600124E-16 ) ) ;
#75697=CARTESIAN_POINT ( 'NONE',  ( 199.6150009768959990, 249.5000000000000568, -2.367926910627510484 ) ) ;
#75701=EDGE_CURVE ( 'NONE', #24951, #59134, #39302, .T. ) ;
#75705=EDGE_CURVE ( 'NONE', #73562, #21018, #62095, .T. ) ;
#75709=CARTESIAN_POINT ( 'NONE',  ( 152.4536156746142410, 250.5000000000000568, -14.50000000000000000 ) ) ;
#75711=DIRECTION ( 'NONE',  ( 0.000000000000000000, 0.000000000000000000, 1.000000000000000000 ) ) ;
#75719=VERTEX_POINT ( 'NONE', #4717 ) ;
#75723=CARTESIAN_POINT ( 'NONE',  ( 199.2296996224750103, 66.10105075020101140, -4.735552035431046215E-14 ) ) ;
#75724=EDGE_CURVE ( 'NONE', #79261, #41691, #51393, .T. ) ;
#75730=CARTESIAN_POINT ( 'NONE',  ( 199.4392256788250677, 65.82574266882504332, -7.741079165001071516 ) ) ;
#75731=CARTESIAN_POINT ( 'NONE',  ( 196.0953433360011786, 25.50289778183998379, 14.17534932438595341 ) ) ;
#75739=ORIENTED_EDGE ( 'NONE', *, *, #7520, .F. ) ;
#75749=VERTEX_POINT ( 'NONE', #68661 ) ;
#75751=ORIENTED_EDGE ( 'NONE', *, *, #67229, .F. ) ;
#75752=CARTESIAN_POINT ( 'NONE',  ( 196.8803347170859865, 73.40565171261609123, 12.49999999999999289 ) ) ;
#75753=AXIS2_PLACEMENT_3D ( 'NONE', #73054, #8185, #22850 ) ;
#75763=TOROIDAL_SURFACE ( 'NONE', #34950, 1.000000000000000000, 0.5000000000000000000 ) ;
#75770=ORIENTED_EDGE ( 'NONE', *, *, #12869, .F. ) ;
#75771=CARTESIAN_POINT ( 'NONE',  ( 183.0442525570908288, 291.1800221208779931, -7.499999999999996447 ) ) ;
#75789=DIRECTION ( 'NONE',  ( -1.000000000000000000, 0.000000000000000000, 0.000000000000000000 ) ) ;
#75791=CARTESIAN_POINT ( 'NONE',  ( 208.6610849207568208, 0.04196010845019451652, 7.500000000000014211 ) ) ;
#75800=DIRECTION ( 'NONE',  ( 0.000000000000000000, 9.656854691831248164E-17, 1.000000000000000000 ) ) ;
#75802=DIRECTION ( 'NONE',  ( 0.000000000000000000, 0.000000000000000000, -1.000000000000000000 ) ) ;
#75817=CIRCLE ( 'NONE', #24386, 5.603083949679982467 ) ;
#75819=DIRECTION ( 'NONE',  ( -0.000000000000000000, -1.000000000000000000, -0.000000000000000000 ) ) ;
#75830=CARTESIAN_POINT ( 'NONE',  ( 165.0685442354929080, 2.974099043298211065, 8.999832278985701706 ) ) ;
#75848=ORIENTED_EDGE ( 'NONE', *, *, #73101, .F. ) ;
#75852=ADVANCED_FACE ( 'NONE', ( #50624 ), #52904, .F. ) ;
#75859=ORIENTED_EDGE ( 'NONE', *, *, #32453, .T. ) ;
#75879=DIRECTION ( 'NONE',  ( 0.000000000000000000, 0.000000000000000000, 1.000000000000000000 ) ) ;
#75887=AXIS2_PLACEMENT_3D ( 'NONE', #70899, #63352, #27338 ) ;
#75892=AXIS2_PLACEMENT_3D ( 'NONE', #58817, #23284, #22352 ) ;
#75903=FACE_OUTER_BOUND ( 'NONE', #57241, .T. ) ;
#75906=EDGE_CURVE ( 'NONE', #82379, #3784, #36290, .T. ) ;
#75909=DIRECTION ( 'NONE',  ( -0.000000000000000000, -1.000000000000000000, -0.000000000000000000 ) ) ;
#75910=CYLINDRICAL_SURFACE ( 'NONE', #92728, 1.999999999999988454 ) ;
#75913=FACE_OUTER_BOUND ( 'NONE', #78258, .T. ) ;
#75915=CARTESIAN_POINT ( 'NONE',  ( 201.5895683924992170, 64.65149228633973166, 9.583120145149372604 ) ) ;
#75917=DIRECTION ( 'NONE',  ( -0.000000000000000000, -1.000000000000000000, -0.000000000000000000 ) ) ;
#75920=CARTESIAN_POINT ( 'NONE',  ( 155.8109286537086859, 19.19772955881914456, -9.232252220101429430 ) ) ;
#75925=( BOUNDED_CURVE ( )  B_SPLINE_CURVE ( 3, ( #82428, #73926, #38858, #67764 ),
 .UNSPECIFIED., .F., .F. ) 
 B_SPLINE_CURVE_WITH_KNOTS ( ( 4, 4 ),
 ( 5.134959379131569968, 6.283185307179586232 ),
 .UNSPECIFIED. ) 
 CURVE ( )  GEOMETRIC_REPRESENTATION_ITEM ( )  RATIONAL_B_SPLINE_CURVE ( ( 1.000000000000000000, 0.8931162488198151062, 0.8931162488198151062, 1.000000000000000000 ) ) 
 REPRESENTATION_ITEM ( '' )  );
#75929=ORIENTED_EDGE ( 'NONE', *, *, #45139, .T. ) ;
#75967=EDGE_CURVE ( 'NONE', #28861, #56456, #42089, .T. ) ;
#75969=EDGE_LOOP ( 'NONE', ( #63206, #4899, #5850, #56096, #85160, #18468 ) ) ;
#75972=ORIENTED_EDGE ( 'NONE', *, *, #55295, .T. ) ;
#75975=EDGE_CURVE ( 'NONE', #7049, #91480, #71004, .T. ) ;
#75996=VERTEX_POINT ( 'NONE', #49217 ) ;
#76004=CARTESIAN_POINT ( 'NONE',  ( 152.6002739434380260, 20.65727164547434569, -10.65122728699565080 ) ) ;
#76009=DIRECTION ( 'NONE',  ( 0.000000000000000000, 0.000000000000000000, 1.000000000000000000 ) ) ;
#76017=CARTESIAN_POINT ( 'NONE',  ( 154.0376014794581465, 19.37029994958559698, -11.97447443758434993 ) ) ;
#76018=AXIS2_PLACEMENT_3D ( 'NONE', #5359, #33748, #12933 ) ;
#76026=EDGE_CURVE ( 'NONE', #82136, #42552, #81626, .T. ) ;
#76036=LINE ( 'NONE', #62796, #60837 ) ;
#76042=CARTESIAN_POINT ( 'NONE',  ( 160.6539576904058606, 293.9636489450775230, 0.000000000000000000 ) ) ;
#76051=DIRECTION ( 'NONE',  ( 0.000000000000000000, 0.000000000000000000, 1.000000000000000000 ) ) ;
#76082=ORIENTED_EDGE ( 'NONE', *, *, #4626, .F. ) ;
#76085=AXIS2_PLACEMENT_3D ( 'NONE', #35400, #58120, #72768 ) ;
#76092=VECTOR ( 'NONE', #67885, 1000.000000000000114 ) ;
#76094=CARTESIAN_POINT ( 'NONE',  ( 185.2519943799831879, 3.000000000000000000, 9.000000000000001776 ) ) ;
#76107=TOROIDAL_SURFACE ( 'NONE', #42777, 1.000000000000000000, 0.5000000000000000000 ) ;
#76115=CARTESIAN_POINT ( 'NONE',  ( 159.4851178187871312, 15.00000000000000000, -6.999999999999999112 ) ) ;
#76117=DIRECTION ( 'NONE',  ( -0.3024135303179478207, -0.9531768234071973378, 4.625929269271478222E-15 ) ) ;
#76119=AXIS2_PLACEMENT_3D ( 'NONE', #69506, #4178, #26889 ) ;
#76127=DIRECTION ( 'NONE',  ( -0.000000000000000000, -0.000000000000000000, 1.000000000000000000 ) ) ;
#76129=CIRCLE ( 'NONE', #44342, 25.00000000000000355 ) ;
#76130=VERTEX_POINT ( 'NONE', #71955 ) ;
#76131=CARTESIAN_POINT ( 'NONE',  ( 196.0143093133015384, 19.33012701892219454, 12.49999999999999289 ) ) ;
#76145=DIRECTION ( 'NONE',  ( -0.000000000000000000, -1.000000000000000000, -0.000000000000000000 ) ) ;
#76146=EDGE_CURVE ( 'NONE', #75053, #85558, #56333, .T. ) ;
#76158=TOROIDAL_SURFACE ( 'NONE', #24710, 1.000000000000000000, 0.5000000000000000000 ) ;
#76160=DIRECTION ( 'NONE',  ( -0.000000000000000000, -1.000000000000000000, -0.000000000000000000 ) ) ;
#76162=CARTESIAN_POINT ( 'NONE',  ( 140.6539576904058606, 250.5000000000000568, -10.49999999999999822 ) ) ;
#76169=PLANE ( 'NONE',  #59346 ) ;
#76171=CIRCLE ( 'NONE', #70103, 0.5000000000000004441 ) ;
#76173=CARTESIAN_POINT ( 'NONE',  ( 169.9462594094670180, 249.5000000000000568, -23.92352941176469017 ) ) ;
#76178=TOROIDAL_SURFACE ( 'NONE', #29357, 3.342139515347628986, 0.5000000000000000000 ) ;
#76180=AXIS2_PLACEMENT_3D ( 'NONE', #19267, #41002, #25426 ) ;
#76184=DIRECTION ( 'NONE',  ( -0.5831039236546632365, 0.7661730729848328370, -0.2701270746362063324 ) ) ;
#76185=VECTOR ( 'NONE', #32253, 1000.000000000000114 ) ;
#76187=LINE ( 'NONE', #41091, #39791 ) ;
#76197=ORIENTED_EDGE ( 'NONE', *, *, #22273, .F. ) ;
#76201=CARTESIAN_POINT ( 'NONE',  ( 196.5385635023627344, 69.63708600452028463, -11.34458575904874067 ) ) ;
#76207=FACE_OUTER_BOUND ( 'NONE', #68408, .T. ) ;
#76226=CIRCLE ( 'NONE', #35420, 2.842139515347646750 ) ;
#76227=CARTESIAN_POINT ( 'NONE',  ( 175.2296996224750103, 154.6894116713782807, 0.000000000000000000 ) ) ;
#76244=CARTESIAN_POINT ( 'NONE',  ( 175.2296996224750103, 275.0000000000000568, 0.000000000000000000 ) ) ;
#76246=AXIS2_PLACEMENT_3D ( 'NONE', #35987, #50668, #92805 ) ;
#76255=DIRECTION ( 'NONE',  ( -0.000000000000000000, -1.000000000000000000, -0.000000000000000000 ) ) ;
#76262=CIRCLE ( 'NONE', #62710, 0.5000000000000017764 ) ;
#76271=CARTESIAN_POINT ( 'NONE',  ( 150.6539576904058606, 293.9636489450775230, -9.103929867429224387 ) ) ;
#76279=CARTESIAN_POINT ( 'NONE',  ( 175.2296996224750103, 150.9142415853029036, 22.83127060016886034 ) ) ;
#76281=CARTESIAN_POINT ( 'NONE',  ( 203.4326848949253019, 287.6892256648253010, -4.962899367210394708 ) ) ;
#76283=CARTESIAN_POINT ( 'NONE',  ( 196.2226484203252426, 42.37842866446141699, 11.63914608143143603 ) ) ;
#76295=ORIENTED_EDGE ( 'NONE', *, *, #1367, .F. ) ;
#76324=AXIS2_PLACEMENT_3D ( 'NONE', #38798, #52087, #38334 ) ;
#76334=CARTESIAN_POINT ( 'NONE',  ( 195.1541288595761330, 21.00000000164155622, -15.11439585901458749 ) ) ;
#76339=EDGE_LOOP ( 'NONE', ( #92653, #13893, #21710, #40117 ) ) ;
#76352=ORIENTED_EDGE ( 'NONE', *, *, #10009, .F. ) ;
#76359=ORIENTED_EDGE ( 'NONE', *, *, #35747, .F. ) ;
#76371=CARTESIAN_POINT ( 'NONE',  ( 0.000000000000000000, 0.000000000000000000, 12.50000000000000000 ) ) ;
#76382=DIRECTION ( 'NONE',  ( -0.9953184226294283787, 0.000000000000000000, 0.09665007798479254009 ) ) ;
#76384=VECTOR ( 'NONE', #12726, 1000.000000000000000 ) ;
#76395=LINE ( 'NONE', #18156, #2965 ) ;
#76397=ORIENTED_EDGE ( 'NONE', *, *, #5821, .F. ) ;
#76398=CARTESIAN_POINT ( 'NONE',  ( 156.4851178187871312, 0.000000000000000000, 10.00000000000000000 ) ) ;
#76404=CARTESIAN_POINT ( 'NONE',  ( 154.2759627658477086, 20.32662787347679512, -12.20915505293937642 ) ) ;
#76413=VERTEX_POINT ( 'NONE', #57329 ) ;
#76416=CARTESIAN_POINT ( 'NONE',  ( 201.0592549708491958, 40.73798607845790798, 10.50000000000000000 ) ) ;
#76420=DIRECTION ( 'NONE',  ( 0.000000000000000000, 0.000000000000000000, 1.000000000000000000 ) ) ;
#76435=CARTESIAN_POINT ( 'NONE',  ( 154.5564663305860904, 20.34868851667230061, -12.19273113389447083 ) ) ;
#76448=ORIENTED_EDGE ( 'NONE', *, *, #6509, .T. ) ;
#76451=ORIENTED_EDGE ( 'NONE', *, *, #69493, .T. ) ;
#76454=ADVANCED_FACE ( 'NONE', ( #56870 ), #63508, .F. ) ;
#76468=ORIENTED_EDGE ( 'NONE', *, *, #66484, .F. ) ;
#76484=DIRECTION ( 'NONE',  ( -0.7957555401921984073, -0.6056179655966479336, 0.000000000000000000 ) ) ;
#76500=CARTESIAN_POINT ( 'NONE',  ( 198.3171862047178422, 65.26485410360638184, 9.727777467356141017 ) ) ;
#76503=EDGE_CURVE ( 'NONE', #4269, #85072, #19, .T. ) ;
#76506=CARTESIAN_POINT ( 'NONE',  ( 199.2296996224750103, 68.12454877777268791, 0.000000000000000000 ) ) ;
#76509=( LENGTH_UNIT ( ) NAMED_UNIT ( * ) SI_UNIT ( .MILLI., .METRE. ) );
#76510=CARTESIAN_POINT ( 'NONE',  ( 209.8616357346614905, 36.89613957940296274, 12.09245862095555601 ) ) ;
#76515=ADVANCED_FACE ( 'NONE', ( #71535 ), #49269, .F. ) ;
#76524=CARTESIAN_POINT ( 'NONE',  ( 156.1449889021179160, 249.5000000000000568, 16.91223866672558529 ) ) ;
#76528=DIRECTION ( 'NONE',  ( -0.8195702660915945570, 0.000000000000000000, 0.5729786897769871823 ) ) ;
#76542=ORIENTED_EDGE ( 'NONE', *, *, #32342, .F. ) ;
#76545=DIRECTION ( 'NONE',  ( 0.000000000000000000, 1.000000000000000000, 0.000000000000000000 ) ) ;
#76555=ORIENTED_EDGE ( 'NONE', *, *, #80560, .T. ) ;
#76566=LINE ( 'NONE', #75164, #92801 ) ;
#76571=ORIENTED_EDGE ( 'NONE', *, *, #56649, .T. ) ;
#76585=DIRECTION ( 'NONE',  ( 0.000000000000000000, 1.000000000000000000, 0.000000000000000000 ) ) ;
#76587=FACE_OUTER_BOUND ( 'NONE', #36130, .T. ) ;
#76588=EDGE_CURVE ( 'NONE', #7661, #92724, #34481, .T. ) ;
#76598=CARTESIAN_POINT ( 'NONE',  ( 197.3322352251145162, 72.17950364302515709, -11.72475155278582015 ) ) ;
#76601=CARTESIAN_POINT ( 'NONE',  ( 196.7071296363291140, 19.50333209967908843, 12.79999999999999538 ) ) ;
#76610=B_SPLINE_CURVE_WITH_KNOTS ( 'NONE', 3,
 ( #36921, #65836, #51569, #85703, #57320, #87547 ),
 .UNSPECIFIED., .F., .F.,
 ( 4, 2, 4 ),
 ( 0.000000000000000000, 0.0008512308255186546487, 0.001702461651037309297 ),
 .UNSPECIFIED. ) ;
#76616=CARTESIAN_POINT ( 'NONE',  ( 154.7659666677267865, 20.47222690886501439, -12.53936336329526391 ) ) ;
#76617=CARTESIAN_POINT ( 'NONE',  ( 195.6913163135599234, 40.51256746173211809, 13.63274697749497300 ) ) ;
#76629=DIRECTION ( 'NONE',  ( -0.000000000000000000, -1.000000000000000000, -0.000000000000000000 ) ) ;
#76638=CARTESIAN_POINT ( 'NONE',  ( 195.4695760097934851, 39.54264841588432233, 15.00000000000000000 ) ) ;
#76659=EDGE_LOOP ( 'NONE', ( #1827, #63552, #59773, #5800 ) ) ;
#76666=ORIENTED_EDGE ( 'NONE', *, *, #28819, .F. ) ;
#76674=EDGE_CURVE ( 'NONE', #73473, #21018, #6093, .T. ) ;
#76682=ORIENTED_EDGE ( 'NONE', *, *, #2931, .T. ) ;
#76689=PRODUCT_CONTEXT ( 'NONE', #54134, 'mechanical' ) ;
#76693=CARTESIAN_POINT ( 'NONE',  ( 175.2296996224750103, 250.5000000000000568, 0.000000000000000000 ) ) ;
#76698=CARTESIAN_POINT ( 'NONE',  ( 196.5998995412811325, 25.70598842973117470, 11.15476524095016941 ) ) ;
#76709=CARTESIAN_POINT ( 'NONE',  ( 0.000000000000000000, 3.000000000000000000, 9.000000000000001776 ) ) ;
#76742=CARTESIAN_POINT ( 'NONE',  ( 169.7306087885279169, 249.5000000000000568, -24.89999999999998792 ) ) ;
#76747=CARTESIAN_POINT ( 'NONE',  ( 206.7809450508160865, 35.77530089738193908, 15.00000000000000000 ) ) ;
#76762=DIRECTION ( 'NONE',  ( 0.000000000000000000, 1.000000000000000000, 0.000000000000000000 ) ) ;
#76774=DIRECTION ( 'NONE',  ( 0.000000000000000000, 0.000000000000000000, -1.000000000000000000 ) ) ;
#76775=ADVANCED_FACE ( 'NONE', ( #21322 ), #45319, .T. ) ;
#76776=CARTESIAN_POINT ( 'NONE',  ( 151.6545538274111209, 20.00000000000000000, -4.874605230979886628 ) ) ;
#76783=ADVANCED_FACE ( 'NONE', ( #43558 ), #72454, .F. ) ;
#76798=CARTESIAN_POINT ( 'NONE',  ( 196.2609727609197421, 20.67721664505789647, -13.53105402382274036 ) ) ;
#76803=VERTEX_POINT ( 'NONE', #15152 ) ;
#76808=AXIS2_PLACEMENT_3D ( 'NONE', #73421, #81424, #30793 ) ;
#76811=DIRECTION ( 'NONE',  ( -0.000000000000000000, -1.000000000000000000, -0.000000000000000000 ) ) ;
#76823=ORIENTED_EDGE ( 'NONE', *, *, #91565, .F. ) ;
#76824=CARTESIAN_POINT ( 'NONE',  ( 180.0056393205866812, 250.0000000000000568, -23.52000000000002800 ) ) ;
#76835=LINE ( 'NONE', #27580, #78938 ) ;
#76840=CARTESIAN_POINT ( 'NONE',  ( 207.8858603214774519, 30.22477065800575957, 14.36621317371163897 ) ) ;
#76850=CARTESIAN_POINT ( 'NONE',  ( 0.000000000000000000, 249.5000000000000568, 12.00000000000000000 ) ) ;
#76851=AXIS2_PLACEMENT_3D ( 'NONE', #83867, #90475, #83385 ) ;
#76852=CARTESIAN_POINT ( 'NONE',  ( 209.8744251295252354, 28.03846817292548366, 15.00000000000000000 ) ) ;
#76856=CARTESIAN_POINT ( 'NONE',  ( 138.6539576904058606, 249.5000000000000568, -10.49999999999999822 ) ) ;
#76858=VERTEX_POINT ( 'NONE', #16085 ) ;
#76859=CARTESIAN_POINT ( 'NONE',  ( 159.4572718888394718, 15.48129629386928663, -10.01740370621926068 ) ) ;
#76862=CARTESIAN_POINT ( 'NONE',  ( 206.1364290716512357, 30.05009751731189738, 14.00000000000000000 ) ) ;
#76874=VERTEX_POINT ( 'NONE', #77452 ) ;
#76877=DIRECTION ( 'NONE',  ( 0.000000000000000000, 0.000000000000000000, 1.000000000000000000 ) ) ;
#76879=ORIENTED_EDGE ( 'NONE', *, *, #62384, .T. ) ;
#76881=CARTESIAN_POINT ( 'NONE',  ( 199.1087447750284980, 64.61450673763175701, 10.46317447812566570 ) ) ;
#76892=EDGE_CURVE ( 'NONE', #45087, #60346, #20160, .T. ) ;
#76895=CARTESIAN_POINT ( 'NONE',  ( 222.8344101925596306, 3.000000000000000000, 10.00000000000000000 ) ) ;
#76902=DIRECTION ( 'NONE',  ( 0.000000000000000000, 0.000000000000000000, 1.000000000000000000 ) ) ;
#76913=EDGE_LOOP ( 'NONE', ( #11834, #4360, #23220, #37944 ) ) ;
#76920=CONICAL_SURFACE ( 'NONE', #30018, 4.025000000000000355, 0.7853981633973095011 ) ;
#76947=CARTESIAN_POINT ( 'NONE',  ( 151.9308040602113579, 19.99432900746804620, -6.268121358087393347 ) ) ;
#76952=DIRECTION ( 'NONE',  ( 0.000000000000000000, -0.000000000000000000, 1.000000000000000000 ) ) ;
#76959=CARTESIAN_POINT ( 'NONE',  ( 197.3748232817348764, 215.0000000000000568, -12.45182892472558933 ) ) ;
#76964=CARTESIAN_POINT ( 'NONE',  ( 196.0143093133015384, 73.40565171261611965, 12.00000000000000711 ) ) ;
#76968=DIRECTION ( 'NONE',  ( 0.000000000000000000, 0.000000000000000000, 1.000000000000000000 ) ) ;
#76971=CARTESIAN_POINT ( 'NONE',  ( 175.2296996224750103, 250.0000000000000568, -24.00000000000000355 ) ) ;
#76977=CARTESIAN_POINT ( 'NONE',  ( 202.9738562182569694, 293.9636489450776367, -54.00000000000000000 ) ) ;
#76980=AXIS2_PLACEMENT_3D ( 'NONE', #25715, #34246, #63152 ) ;
#76987=CARTESIAN_POINT ( 'NONE',  ( 207.8033511093241827, 36.73028256270350766, 13.58522159759119852 ) ) ;
#76990=CARTESIAN_POINT ( 'NONE',  ( 196.0143093133015384, 20.19615242270663913, -11.99999999999998579 ) ) ;
#77003=ADVANCED_FACE ( 'NONE', ( #42385 ), #63745, .T. ) ;
#77006=ORIENTED_EDGE ( 'NONE', *, *, #78174, .F. ) ;
#77009=LINE ( 'NONE', #61871, #56561 ) ;
#77019=ORIENTED_EDGE ( 'NONE', *, *, #43760, .F. ) ;
#77023=ADVANCED_FACE ( 'NONE', ( #27743 ), #45448, .T. ) ;
#77033=ORIENTED_EDGE ( 'NONE', *, *, #78611, .T. ) ;
#77049=ADVANCED_FACE ( 'NONE', ( #26324 ), #62809, .F. ) ;
#77060=DIRECTION ( 'NONE',  ( 0.000000000000000000, 1.000000000000000000, 0.000000000000000000 ) ) ;
#77077=DIRECTION ( 'NONE',  ( 1.000000000000000000, -1.805997381456195657E-15, 0.000000000000000000 ) ) ;
#77078=FACE_OUTER_BOUND ( 'NONE', #55348, .T. ) ;
#77091=CARTESIAN_POINT ( 'NONE',  ( 183.0442525570908288, 275.0000000000000568, -7.500000000000000000 ) ) ;
#77093=CARTESIAN_POINT ( 'NONE',  ( 140.6539576904058606, 249.5000000000000568, 10.50000000000000000 ) ) ;
#77103=CARTESIAN_POINT ( 'NONE',  ( 195.2369406736065116, 39.74098473494063910, 14.99224007599141473 ) ) ;
#77109=CIRCLE ( 'NONE', #1476, 3.842139515347647638 ) ;
#77113=CARTESIAN_POINT ( 'NONE',  ( 150.4957602436334412, 21.00000000000000000, 3.637614988394419768 ) ) ;
#77116=AXIS2_PLACEMENT_3D ( 'NONE', #62504, #83782, #75291 ) ;
#77140=LINE ( 'NONE', #12271, #37128 ) ;
#77141=CARTESIAN_POINT ( 'NONE',  ( 195.5916183739827545, 25.43510842100078051, 14.50572835022993701 ) ) ;
#77144=ORIENTED_EDGE ( 'NONE', *, *, #11080, .F. ) ;
#77161=ORIENTED_EDGE ( 'NONE', *, *, #42403, .F. ) ;
#77162=FACE_OUTER_BOUND ( 'NONE', #54651, .T. ) ;
#77177=EDGE_LOOP ( 'NONE', ( #85772, #53618, #86937, #14189 ) ) ;
#77183=VECTOR ( 'NONE', #93642, 1000.000000000000000 ) ;
#77201=LINE ( 'NONE', #63027, #48938 ) ;
#77208=EDGE_CURVE ( 'NONE', #16269, #52326, #42342, .T. ) ;
#77210=ADVANCED_FACE ( 'NONE', ( #64227 ), #49962, .T. ) ;
#77213=FACE_OUTER_BOUND ( 'NONE', #47443, .T. ) ;
#77215=CARTESIAN_POINT ( 'NONE',  ( 183.0442525570908288, 293.9636489450775230, 0.000000000000000000 ) ) ;
#77224=B_SPLINE_CURVE_WITH_KNOTS ( 'NONE', 3,
 ( #73037, #64584, #72128, #7244 ),
 .UNSPECIFIED., .F., .F.,
 ( 4, 4 ),
 ( 1.734723475976807094E-18, 0.0008449500572417431576 ),
 .UNSPECIFIED. ) ;
#77227=LINE ( 'NONE', #10939, #83101 ) ;
#77229=DIRECTION ( 'NONE',  ( 0.000000000000000000, 1.000000000000000000, 0.000000000000000000 ) ) ;
#77242=DIRECTION ( 'NONE',  ( 0.000000000000000000, 0.000000000000000000, 1.000000000000000000 ) ) ;
#77247=CIRCLE ( 'NONE', #60630, 25.00000000000000355 ) ;
#77258=EDGE_LOOP ( 'NONE', ( #84363, #43260, #72740, #55012 ) ) ;
#77260=VERTEX_POINT ( 'NONE', #44718 ) ;
#77277=CARTESIAN_POINT ( 'NONE',  ( 197.2116943569230045, 249.5000000000000568, -12.92446933126075592 ) ) ;
#77289=VERTEX_POINT ( 'NONE', #21092 ) ;
#77290=FACE_OUTER_BOUND ( 'NONE', #80985, .T. ) ;
#77317=CYLINDRICAL_SURFACE ( 'NONE', #32285, 2.000000000000000888 ) ;
#77320=CIRCLE ( 'NONE', #71318, 24.50000000000000355 ) ;
#77327=CARTESIAN_POINT ( 'NONE',  ( 155.9223079842153368, 17.31716537716996740, -7.900495735315888446 ) ) ;
#77329=DIRECTION ( 'NONE',  ( -0.5000000000000046629, 0.8660254037844359321, 0.000000000000000000 ) ) ;
#77344=CARTESIAN_POINT ( 'NONE',  ( 158.3135449435333442, 1.828427124746191623, -9.000000000000001776 ) ) ;
#77346=EDGE_LOOP ( 'NONE', ( #45354, #79649, #24856, #6952 ) ) ;
#77369=DIRECTION ( 'NONE',  ( 0.000000000000000000, 1.000000000000000000, 0.000000000000000000 ) ) ;
#77388=AXIS2_PLACEMENT_3D ( 'NONE', #50030, #78010, #20704 ) ;
#77397=EDGE_LOOP ( 'NONE', ( #35226, #92157, #26211, #81009 ) ) ;
#77399=CIRCLE ( 'NONE', #72866, 4.499999999999990230 ) ;
#77404=ORIENTED_EDGE ( 'NONE', *, *, #88613, .T. ) ;
#77406=ORIENTED_EDGE ( 'NONE', *, *, #72224, .F. ) ;
#77413=CARTESIAN_POINT ( 'NONE',  ( 152.4883615486606914, 19.90193753873172611, -8.271207965221249125 ) ) ;
#77420=EDGE_CURVE ( 'NONE', #54877, #13227, #35774, .T. ) ;
#77426=CARTESIAN_POINT ( 'NONE',  ( 209.1374487190023501, 30.94653725228601715, 12.00000000000000000 ) ) ;
#77435=CARTESIAN_POINT ( 'NONE',  ( 197.2116943569230330, 250.0000000000000568, -11.92446933126075237 ) ) ;
#77442=EDGE_CURVE ( 'NONE', #75053, #4038, #82095, .T. ) ;
#77452=CARTESIAN_POINT ( 'NONE',  ( 208.4306832106271088, 20.44233620800389772, 7.500000000000013323 ) ) ;
#77453=LINE ( 'NONE', #4543, #58682 ) ;
#77458=B_SPLINE_CURVE_WITH_KNOTS ( 'NONE', 3,
 ( #76094, #83178, #4586, #10277, #68058, #33460 ),
 .UNSPECIFIED., .F., .F.,
 ( 4, 2, 4 ),
 ( 0.000000000000000000, 0.0005356813221244592508, 0.001071362644248918502 ),
 .UNSPECIFIED. ) ;
#77475=LINE ( 'NONE', #20181, #44485 ) ;
#77497=CARTESIAN_POINT ( 'NONE',  ( 154.9842916688209868, 128.0000000000000568, -12.88888888888889461 ) ) ;
#77501=ORIENTED_EDGE ( 'NONE', *, *, #47924, .T. ) ;
#77510=ORIENTED_EDGE ( 'NONE', *, *, #49942, .T. ) ;
#77517=VECTOR ( 'NONE', #89738, 1000.000000000000114 ) ;
#77518=CARTESIAN_POINT ( 'NONE',  ( 156.6530531571616791, 18.17946993580249782, 9.832064661605528499 ) ) ;
#77526=LINE ( 'NONE', #5572, #3437 ) ;
#77528=DIRECTION ( 'NONE',  ( 0.000000000000000000, 1.000000000000000000, 0.000000000000000000 ) ) ;
#77529=AXIS2_PLACEMENT_3D ( 'NONE', #12187, #4616, #27819 ) ;
#77532=ORIENTED_EDGE ( 'NONE', *, *, #60248, .T. ) ;
#77533=CARTESIAN_POINT ( 'NONE',  ( 195.4781563537916043, 27.48493576247232895, 15.00000000000000000 ) ) ;
#77537=ADVANCED_FACE ( 'NONE', ( #74536 ), #75691, .T. ) ;
#77548=CARTESIAN_POINT ( 'NONE',  ( 193.6287975281925071, 275.6568570078858329, 16.89650703334467963 ) ) ;
#77551=VECTOR ( 'NONE', #10853, 1000.000000000000000 ) ;
#77552=VECTOR ( 'NONE', #58380, 1000.000000000000000 ) ;
#77562=ADVANCED_FACE ( 'NONE', ( #46114 ), #2114, .T. ) ;
#77564=CARTESIAN_POINT ( 'NONE',  ( 175.2296996224750103, 140.2072866198470251, 0.000000000000000000 ) ) ;
#77575=CARTESIAN_POINT ( 'NONE',  ( 196.1601127431574412, 41.43610473273403727, 14.06370431049791137 ) ) ;
#77584=ORIENTED_EDGE ( 'NONE', *, *, #65290, .F. ) ;
#77585=DIRECTION ( 'NONE',  ( 0.000000000000000000, 0.000000000000000000, 1.000000000000000000 ) ) ;
#77588=CARTESIAN_POINT ( 'NONE',  ( 208.4306832106271088, -74.55766379199613425, -7.500000000000013323 ) ) ;
#77592=AXIS2_PLACEMENT_3D ( 'NONE', #80576, #65948, #51687 ) ;
#77595=AXIS2_PLACEMENT_3D ( 'NONE', #69307, #33315, #3980 ) ;
#77600=ORIENTED_EDGE ( 'NONE', *, *, #24713, .F. ) ;
#77601=DIRECTION ( 'NONE',  ( 0.000000000000000000, 1.000000000000000000, 0.000000000000000000 ) ) ;
#77605=AXIS2_PLACEMENT_3D ( 'NONE', #46088, #18153, #67886 ) ;
#77606=ORIENTED_EDGE ( 'NONE', *, *, #54222, .F. ) ;
#77612=CARTESIAN_POINT ( 'NONE',  ( 198.0296422097436846, 67.77566895945791714, -9.842458531120671594 ) ) ;
#77614=DIRECTION ( 'NONE',  ( -0.3994899938748465162, 0.000000000000000000, -0.9167375550253601402 ) ) ;
#77615=CARTESIAN_POINT ( 'NONE',  ( 138.6539576904058606, 130.8284271247462414, 11.67157287525380838 ) ) ;
#77618=VERTEX_POINT ( 'NONE', #9188 ) ;
#77632=EDGE_CURVE ( 'NONE', #20922, #37280, #89187, .T. ) ;
#77636=ORIENTED_EDGE ( 'NONE', *, *, #10818, .F. ) ;
#77652=ORIENTED_EDGE ( 'NONE', *, *, #57360, .T. ) ;
#77653=CARTESIAN_POINT ( 'NONE',  ( 194.7155524329731122, 19.93649182339144232, -14.17849501842133719 ) ) ;
#77655=VECTOR ( 'NONE', #28760, 1000.000000000000000 ) ;
#77675=CIRCLE ( 'NONE', #64128, 5.568361562975243650 ) ;
#77677=CARTESIAN_POINT ( 'NONE',  ( 196.2452211277167748, 71.67373103464963435, 13.59235650557800135 ) ) ;
#77690=CIRCLE ( 'NONE', #55041, 1.000000000000000888 ) ;
#77692=EDGE_CURVE ( 'NONE', #22214, #17985, #80225, .T. ) ;
#77693=DIRECTION ( 'NONE',  ( 0.000000000000000000, 0.000000000000000000, 1.000000000000000000 ) ) ;
#77705=LINE ( 'NONE', #28912, #46802 ) ;
#77719=CARTESIAN_POINT ( 'NONE',  ( 185.7724743053495615, 214.9732557907763635, 23.01307087489506742 ) ) ;
#77722=CIRCLE ( 'NONE', #14215, 2.000000000000001776 ) ;
#77728=CIRCLE ( 'NONE', #50488, 4.999999999999977796 ) ;
#77734=ORIENTED_EDGE ( 'NONE', *, *, #66553, .F. ) ;
#77739=CIRCLE ( 'NONE', #36916, 25.00000000000000355 ) ;
#77752=DIRECTION ( 'NONE',  ( 0.9531768234071978929, -0.3024135303179465439, -0.000000000000000000 ) ) ;
#77757=ADVANCED_FACE ( 'NONE', ( #59416 ), #90128, .T. ) ;
#77768=DIRECTION ( 'NONE',  ( -0.000000000000000000, 1.000000000000000000, -0.000000000000000000 ) ) ;
#77773=B_SPLINE_CURVE_WITH_KNOTS ( 'NONE', 3,
 ( #81818, #45833, #44900, #74737, #75200, #24530, #9858, #38732, #67638, #15574, #36889, #87520, #44444, #73350, #8462, #73803, #66248, #59136 ),
 .UNSPECIFIED., .F., .F.,
 ( 4, 2, 2, 2, 2, 2, 2, 2, 4 ),
 ( 0.000000000000000000, 0.0006105671578862054225, 0.001221134315772410845, 0.001831701473658616268, 0.002442268631544821690, 0.003052835789431026896, 0.003663402947317232535, 0.004273970105203438175, 0.004884537263089643380 ),
 .UNSPECIFIED. ) ;
#77779=DIRECTION ( 'NONE',  ( 0.000000000000000000, 1.000000000000000000, 0.000000000000000000 ) ) ;
#77804=CARTESIAN_POINT ( 'NONE',  ( 210.1640492649783312, 37.84931640281050846, 12.09245862095555779 ) ) ;
#77806=DIRECTION ( 'NONE',  ( -1.000000000000000000, 0.000000000000000000, -5.880589007913310608E-16 ) ) ;
#77809=CARTESIAN_POINT ( 'NONE',  ( 157.4851178187871312, 14.99999999999999645, -9.000000000000000000 ) ) ;
#77819=ORIENTED_EDGE ( 'NONE', *, *, #56462, .F. ) ;
#77824=EDGE_LOOP ( 'NONE', ( #74346, #40576, #21762, #20564, #7504, #24767 ) ) ;
#77841=DIRECTION ( 'NONE',  ( 1.000000000000000000, -0.000000000000000000, 0.000000000000000000 ) ) ;
#77849=CARTESIAN_POINT ( 'NONE',  ( 159.4851178187871312, 3.000000000000000000, 9.000000000000001776 ) ) ;
#77857=VERTEX_POINT ( 'NONE', #45629 ) ;
#77868=EDGE_CURVE ( 'NONE', #33195, #31059, #42432, .T. ) ;
#77880=ORIENTED_EDGE ( 'NONE', *, *, #48014, .F. ) ;
#77882=( BOUNDED_SURFACE ( )  B_SPLINE_SURFACE ( 3, 2, ( 
 ( #76131, #76601, #61478 ),
 ( #41036, #39642, #69034 ),
 ( #10781, #83216, #69491 ),
 ( #68566, #69964, #91245 ),
 ( #3702, #32587, #18361 ),
 ( #61926, #90308, #33983 ),
 ( #48631, #17903, #47221 ),
 ( #40577, #46757, #19300 ),
 ( #4164, #33036, #47702 ),
 ( #89852, #25013, #90763 ) ),
 .UNSPECIFIED., .F., .F., .F. ) 
 B_SPLINE_SURFACE_WITH_KNOTS ( ( 4, 2, 2, 2, 4 ),
 ( 3, 3 ),
 ( 6.806784082777886269, 7.068583470577035399, 7.330382858376184529, 7.592182246175333660, 7.853981633974482790 ),
 ( 0.000000000000000000, 1.000000000000000000 ),
 .UNSPECIFIED. ) 
 GEOMETRIC_REPRESENTATION_ITEM ( )  RATIONAL_B_SPLINE_SURFACE ( (
 ( 1.000000000000000000, 0.7905694150420951027, 1.000000000000000000),
 ( 1.000000000000000000, 0.8144940228947546990, 1.000000000000000000),
 ( 1.000000000000000000, 0.8408337462327619694, 1.000000000000000000),
 ( 1.000000000000000000, 0.8912170613361163340, 1.000000000000000000),
 ( 1.000000000000000000, 0.9152160855729576383, 1.000000000000000000),
 ( 1.000000000000000000, 0.9556126078140139146, 1.000000000000000000),
 ( 1.000000000000000000, 0.9720148405105164535, 1.000000000000000000),
 ( 1.000000000000000000, 0.9942062568700493763, 1.000000000000000000),
 ( 1.000000000000000000, 1.000000000000000000, 1.000000000000000000),
 ( 1.000000000000000000, 1.000000000000000000, 1.000000000000000000) ) ) 
 REPRESENTATION_ITEM ( '' )  SURFACE ( )  );
#77887=VERTEX_POINT ( 'NONE', #23878 ) ;
#77888=( BOUNDED_CURVE ( )  B_SPLINE_CURVE ( 3, ( #13063, #33401, #48534, #84519 ),
 .UNSPECIFIED., .F., .F. ) 
 B_SPLINE_CURVE_WITH_KNOTS ( ( 4, 4 ),
 ( 4.278565243615663150, 4.712388980384691450 ),
 .UNSPECIFIED. ) 
 CURVE ( )  GEOMETRIC_REPRESENTATION_ITEM ( )  RATIONAL_B_SPLINE_CURVE ( ( 1.000000000000000000, 0.9843778111405747655, 0.9843778111405747655, 1.000000000000000000 ) ) 
 REPRESENTATION_ITEM ( '' )  );
#77889=AXIS2_PLACEMENT_3D ( 'NONE', #25051, #24103, #16541 ) ;
#77898=CARTESIAN_POINT ( 'NONE',  ( 200.2296996224750103, 68.12454877777268791, 0.000000000000000000 ) ) ;
#77904=CARTESIAN_POINT ( 'NONE',  ( 212.2107582607290510, 32.98517505407394168, 14.69807322781335657 ) ) ;
#77913=CARTESIAN_POINT ( 'NONE',  ( 203.5977283565847813, 62.01285785379744198, -7.000000000000000888 ) ) ;
#77921=CARTESIAN_POINT ( 'NONE',  ( 207.8905253643919195, 30.23467176727723782, 14.36943405361669157 ) ) ;
#77924=LINE ( 'NONE', #54248, #89514 ) ;
#77925=CARTESIAN_POINT ( 'NONE',  ( 188.7149167944524493, 8.542400036368780647, 10.00000000000000000 ) ) ;
#77936=DIRECTION ( 'NONE',  ( -0.000000000000000000, -0.000000000000000000, 1.000000000000000000 ) ) ;
#77939=CARTESIAN_POINT ( 'NONE',  ( 200.2349812190172713, 66.43136063442170780, 7.741079165001067963 ) ) ;
#77948=ADVANCED_FACE ( 'NONE', ( #17718 ), #38551, .F. ) ;
#77957=DIRECTION ( 'NONE',  ( 0.000000000000000000, 0.000000000000000000, 1.000000000000000000 ) ) ;
#77970=ORIENTED_EDGE ( 'NONE', *, *, #46209, .T. ) ;
#77982=CARTESIAN_POINT ( 'NONE',  ( 154.4030696693785956, 128.9756020784251120, -12.16842021443607713 ) ) ;
#77996=ORIENTED_EDGE ( 'NONE', *, *, #49490, .F. ) ;
#78001=CARTESIAN_POINT ( 'NONE',  ( 196.6877655503061533, 293.9636489450776367, -59.00000000000003553 ) ) ;
#78002=DIRECTION ( 'NONE',  ( -1.000000000000000000, -0.000000000000000000, -0.000000000000000000 ) ) ;
#78003=DIRECTION ( 'NONE',  ( 0.000000000000000000, 0.000000000000000000, 1.000000000000000000 ) ) ;
#78010=DIRECTION ( 'NONE',  ( -0.9693563597868444237, -0.2456588035076248677, -0.000000000000000000 ) ) ;
#78012=ORIENTED_EDGE ( 'NONE', *, *, #34464, .T. ) ;
#78014=DIRECTION ( 'NONE',  ( -0.000000000000000000, -0.000000000000000000, -1.000000000000000000 ) ) ;
#78031=AXIS2_PLACEMENT_3D ( 'NONE', #48597, #63789, #50003 ) ;
#78043=CARTESIAN_POINT ( 'NONE',  ( 159.4851178187871312, 0.000000000000000000, 9.000000000000001776 ) ) ;
#78056=CARTESIAN_POINT ( 'NONE',  ( 195.8217498488526189, 40.98913131717844038, 14.50814483734951921 ) ) ;
#78064=ORIENTED_EDGE ( 'NONE', *, *, #53698, .F. ) ;
#78065=CARTESIAN_POINT ( 'NONE',  ( 150.7067237505056596, 20.03350844490810800, 5.072059973230453878 ) ) ;
#78067=CARTESIAN_POINT ( 'NONE',  ( 207.8273378092535211, 29.30631323223389018, 13.54762445178045738 ) ) ;
#78077=VERTEX_POINT ( 'NONE', #56526 ) ;
#78084=ORIENTED_EDGE ( 'NONE', *, *, #46974, .F. ) ;
#78095=ORIENTED_EDGE ( 'NONE', *, *, #63231, .T. ) ;
#78101=ORIENTED_EDGE ( 'NONE', *, *, #20867, .F. ) ;
#78108=EDGE_CURVE ( 'NONE', #90054, #25728, #85383, .T. ) ;
#78112=EDGE_LOOP ( 'NONE', ( #78695, #78688, #680, #11535 ) ) ;
#78113=DIRECTION ( 'NONE',  ( 0.000000000000000000, -1.000000000000000000, 0.000000000000000000 ) ) ;
#78116=EDGE_CURVE ( 'NONE', #53738, #19033, #81432, .T. ) ;
#78128=ORIENTED_EDGE ( 'NONE', *, *, #46981, .T. ) ;
#78129=ORIENTED_EDGE ( 'NONE', *, *, #36918, .F. ) ;
#78130=CARTESIAN_POINT ( 'NONE',  ( 202.9738562182569694, 293.9636489450776367, 3.999999999999991562 ) ) ;
#78153=CARTESIAN_POINT ( 'NONE',  ( 165.0427047786672290, 275.0000000000000568, 23.37680765314704701 ) ) ;
#78155=CARTESIAN_POINT ( 'NONE',  ( 201.2104617360081704, 25.32700003806615996, 10.00000000000000000 ) ) ;
#78166=CARTESIAN_POINT ( 'NONE',  ( 138.6539576904058606, 249.5000000000000568, 10.50000000000000000 ) ) ;
#78174=EDGE_CURVE ( 'NONE', #50719, #79037, #92313, .T. ) ;
#78177=CARTESIAN_POINT ( 'NONE',  ( 208.4306832106271088, -74.55766379199613425, 0.000000000000000000 ) ) ;
#78179=CARTESIAN_POINT ( 'NONE',  ( 165.2494399300530290, 8.542400036368780647, 10.00000000000000000 ) ) ;
#78191=DIRECTION ( 'NONE',  ( 0.000000000000000000, 1.000000000000000000, 0.000000000000000000 ) ) ;
#78192=DIRECTION ( 'NONE',  ( 0.000000000000000000, -0.000000000000000000, 1.000000000000000000 ) ) ;
#78193=EDGE_CURVE ( 'NONE', #35594, #75749, #50005, .T. ) ;
#78207=ORIENTED_EDGE ( 'NONE', *, *, #56930, .T. ) ;
#78211=EDGE_CURVE ( 'NONE', #10842, #86547, #22759, .T. ) ;
#78223=DIRECTION ( 'NONE',  ( 1.000000000000000000, 0.000000000000000000, 0.000000000000000000 ) ) ;
#78229=ORIENTED_EDGE ( 'NONE', *, *, #34825, .T. ) ;
#78236=ORIENTED_EDGE ( 'NONE', *, *, #899, .F. ) ;
#78240=ADVANCED_FACE ( 'NONE', ( #47510 ), #87771, .T. ) ;
#78258=EDGE_LOOP ( 'NONE', ( #82843, #73414, #92141, #82971 ) ) ;
#78265=CARTESIAN_POINT ( 'NONE',  ( 197.5379522065468052, 250.0000000000000568, -11.97918851819043873 ) ) ;
#78266=FACE_OUTER_BOUND ( 'NONE', #49102, .T. ) ;
#78274=DIRECTION ( 'NONE',  ( -1.000000000000000000, -0.000000000000000000, -0.000000000000000000 ) ) ;
#78276=DIRECTION ( 'NONE',  ( -1.000000000000000000, 0.000000000000000000, 0.000000000000000000 ) ) ;
#78279=LINE ( 'NONE', #88132, #44249 ) ;
#78294=VERTEX_POINT ( 'NONE', #91999 ) ;
#78309=CARTESIAN_POINT ( 'NONE',  ( 175.2296996224750103, 276.0000000000000568, 0.000000000000000000 ) ) ;
#78317=CARTESIAN_POINT ( 'NONE',  ( 152.4536156746142410, 275.5000000000000568, -12.49999999999999289 ) ) ;
#78327=VERTEX_POINT ( 'NONE', #76416 ) ;
#78355=CIRCLE ( 'NONE', #67727, 6.286090667950827715 ) ;
#78361=CARTESIAN_POINT ( 'NONE',  ( 164.2231345125756263, 300.2961574867697436, -7.500000000000000000 ) ) ;
#78373=DIRECTION ( 'NONE',  ( 0.5370370370370398660, -2.048677426712644618E-14, 0.8435586647355814982 ) ) ;
#78380=PLANE ( 'NONE',  #13404 ) ;
#78397=DIRECTION ( 'NONE',  ( 0.000000000000000000, 0.000000000000000000, -1.000000000000000000 ) ) ;
#78401=EDGE_CURVE ( 'NONE', #83027, #37103, #57599, .T. ) ;
#78402=CARTESIAN_POINT ( 'NONE',  ( 175.2296996224749250, 275.5000000000000568, -24.99999999999999289 ) ) ;
#78416=CIRCLE ( 'NONE', #2835, 4.000000000000003553 ) ;
#78430=ORIENTED_EDGE ( 'NONE', *, *, #15267, .T. ) ;
#78434=( BOUNDED_CURVE ( )  B_SPLINE_CURVE ( 3, ( #75730, #90379, #62963, #84224 ),
 .UNSPECIFIED., .F., .F. ) 
 B_SPLINE_CURVE_WITH_KNOTS ( ( 4, 4 ),
 ( 6.022196528194273313, 6.283185307179586232 ),
 .UNSPECIFIED. ) 
 CURVE ( )  GEOMETRIC_REPRESENTATION_ITEM ( )  RATIONAL_B_SPLINE_CURVE ( ( 1.000000000000000000, 0.9943317885200936290, 0.9943317885200936290, 1.000000000000000000 ) ) 
 REPRESENTATION_ITEM ( '' )  );
#78442=CARTESIAN_POINT ( 'NONE',  ( 198.6357980679388220, 66.99333465236068719, 8.405329074384228605 ) ) ;
#78443=CARTESIAN_POINT ( 'NONE',  ( 152.4536156746142410, 130.6065089285656313, -11.50000000000000000 ) ) ;
#78446=EDGE_LOOP ( 'NONE', ( #55489, #78901, #79222, #44963 ) ) ;
#78455=VERTEX_POINT ( 'NONE', #83485 ) ;
#78461=FACE_OUTER_BOUND ( 'NONE', #21123, .T. ) ;
#78473=DIRECTION ( 'NONE',  ( 1.000000000000000000, 0.000000000000000000, 0.000000000000000000 ) ) ;
#78480=VECTOR ( 'NONE', #89170, 1000.000000000000000 ) ;
#78488=CARTESIAN_POINT ( 'NONE',  ( 196.7631351679105194, 292.9610677455149812, -7.940802731072580833 ) ) ;
#78502=DIRECTION ( 'NONE',  ( 0.7957555401921980742, 0.6056179655966482667, 0.000000000000000000 ) ) ;
#78504=LINE ( 'NONE', #13642, #74764 ) ;
#78518=CARTESIAN_POINT ( 'NONE',  ( 195.0811277900482992, 39.56969527624787730, 15.19607843187435137 ) ) ;
#78527=ORIENTED_EDGE ( 'NONE', *, *, #70157, .F. ) ;
#78528=CARTESIAN_POINT ( 'NONE',  ( 151.0356227161011020, 20.07892719423917427, 6.469110745572608678 ) ) ;
#78530=DIRECTION ( 'NONE',  ( 0.000000000000000000, 1.000000000000000000, 0.000000000000000000 ) ) ;
#78539=ORIENTED_EDGE ( 'NONE', *, *, #87659, .T. ) ;
#78545=ORIENTED_EDGE ( 'NONE', *, *, #45139, .F. ) ;
#78554=CARTESIAN_POINT ( 'NONE',  ( 199.4767649826798674, 41.62711076580291092, 9.000000000000001776 ) ) ;
#78562=ORIENTED_EDGE ( 'NONE', *, *, #80612, .T. ) ;
#78572=CARTESIAN_POINT ( 'NONE',  ( 208.4306832106271088, -74.55766379199613425, 0.000000000000000000 ) ) ;
#78586=ORIENTED_EDGE ( 'NONE', *, *, #41597, .F. ) ;
#78587=ORIENTED_EDGE ( 'NONE', *, *, #49649, .F. ) ;
#78588=CARTESIAN_POINT ( 'NONE',  ( 208.0849289532862372, 28.61657807523931396, 11.99999999999999822 ) ) ;
#78602=CARTESIAN_POINT ( 'NONE',  ( 201.2509219215139922, 65.09645894978945080, -5.329070518200752656E-14 ) ) ;
#78603=FACE_OUTER_BOUND ( 'NONE', #50973, .T. ) ;
#78611=EDGE_CURVE ( 'NONE', #88883, #62986, #39972, .T. ) ;
#78612=CYLINDRICAL_SURFACE ( 'NONE', #21781, 0.5000000000000004441 ) ;
#78614=CIRCLE ( 'NONE', #37753, 0.5000000000000004441 ) ;
#78619=VECTOR ( 'NONE', #26186, 1000.000000000000000 ) ;
#78627=DIRECTION ( 'NONE',  ( -0.000000000000000000, 1.000000000000000000, -0.000000000000000000 ) ) ;
#78636=EDGE_CURVE ( 'NONE', #48115, #73985, #84893, .T. ) ;
#78667=ORIENTED_EDGE ( 'NONE', *, *, #73884, .F. ) ;
#78673=CIRCLE ( 'NONE', #56035, 1.999999999999992673 ) ;
#78676=ORIENTED_EDGE ( 'NONE', *, *, #60993, .F. ) ;
#78688=ORIENTED_EDGE ( 'NONE', *, *, #30078, .F. ) ;
#78695=ORIENTED_EDGE ( 'NONE', *, *, #88464, .T. ) ;
#78696=CARTESIAN_POINT ( 'NONE',  ( 195.2251806849246805, 24.84528228517684667, 13.27436667035662232 ) ) ;
#78710=CARTESIAN_POINT ( 'NONE',  ( 156.4947056272797852, 21.00000000000000000, 15.00000000000000000 ) ) ;
#78720=ADVANCED_FACE ( 'NONE', ( #63640 ), #438, .F. ) ;
#78731=CARTESIAN_POINT ( 'NONE',  ( 170.8178014930282700, 8.542400036368780647, -9.000000000000001776 ) ) ;
#78734=LINE ( 'NONE', #85819, #29076 ) ;
#78735=LINE ( 'NONE', #35172, #41256 ) ;
#78743=EDGE_CURVE ( 'NONE', #59134, #23299, #29952, .T. ) ;
#78746=EDGE_LOOP ( 'NONE', ( #33494, #55559, #51729, #61798 ) ) ;
#78748=AXIS2_PLACEMENT_3D ( 'NONE', #90682, #80709, #72232 ) ;
#78750=DIRECTION ( 'NONE',  ( 0.000000000000000000, 0.000000000000000000, 1.000000000000000000 ) ) ;
#78768=DIRECTION ( 'NONE',  ( 0.9998346970812741485, 0.000000000000000000, -0.01818181818182024179 ) ) ;
#78776=CARTESIAN_POINT ( 'NONE',  ( 140.6539576904058606, 276.0000000000000568, 10.50000000000000000 ) ) ;
#78783=ORIENTED_EDGE ( 'NONE', *, *, #14703, .F. ) ;
#78786=ORIENTED_EDGE ( 'NONE', *, *, #40401, .F. ) ;
#78803=VERTEX_POINT ( 'NONE', #28108 ) ;
#78809=VERTEX_POINT ( 'NONE', #93409 ) ;
#78812=ORIENTED_EDGE ( 'NONE', *, *, #15031, .F. ) ;
#78817=AXIS2_PLACEMENT_3D ( 'NONE', #90028, #82924, #19361 ) ;
#78832=DIRECTION ( 'NONE',  ( 0.000000000000000000, 0.000000000000000000, 1.000000000000000000 ) ) ;
#78836=CARTESIAN_POINT ( 'NONE',  ( 175.2296996224750103, 247.0000000000001137, 9.550761578869391144 ) ) ;
#78839=CARTESIAN_POINT ( 'NONE',  ( 164.2231345125756263, 300.2961574867697436, -7.500000000000000000 ) ) ;
#78854=CARTESIAN_POINT ( 'NONE',  ( 209.1929142650026279, 37.10830422238664283, 12.90287354992391045 ) ) ;
#78874=TOROIDAL_SURFACE ( 'NONE', #38023, 24.00000000000000355, 1.000000000000000000 ) ;
#78896=CARTESIAN_POINT ( 'NONE',  ( 139.6539576904058606, 132.0000000000000568, -10.49999999999999822 ) ) ;
#78901=ORIENTED_EDGE ( 'NONE', *, *, #75967, .F. ) ;
#78909=EDGE_LOOP ( 'NONE', ( #26472, #19489, #9245, #89425 ) ) ;
#78914=LINE ( 'NONE', #84598, #32604 ) ;
#78915=DIRECTION ( 'NONE',  ( 0.000000000000000000, 1.000000000000000000, 0.000000000000000000 ) ) ;
#78916=CARTESIAN_POINT ( 'NONE',  ( 155.4202272374197946, 20.25578850494681760, 12.04866793599625296 ) ) ;
#78923=DIRECTION ( 'NONE',  ( 0.000000000000000000, 1.000000000000000000, 0.000000000000000000 ) ) ;
#78924=EDGE_CURVE ( 'NONE', #44442, #61882, #71661, .T. ) ;
#78927=VERTEX_POINT ( 'NONE', #7696 ) ;
#78928=ORIENTED_EDGE ( 'NONE', *, *, #66277, .F. ) ;
#78929=DIRECTION ( 'NONE',  ( -0.000000000000000000, -1.000000000000000000, -0.000000000000000000 ) ) ;
#78938=VECTOR ( 'NONE', #41767, 1000.000000000000000 ) ;
#78962=CARTESIAN_POINT ( 'NONE',  ( 194.7453183674696220, 20.99999999999998934, 15.62500000000049205 ) ) ;
#78975=LINE ( 'NONE', #42992, #9505 ) ;
#78985=EDGE_LOOP ( 'NONE', ( #28045, #56323, #57978, #5736, #40328, #5277, #21730, #69221 ) ) ;
#78986=CARTESIAN_POINT ( 'NONE',  ( 196.1963538710215857, 305.7026273589066250, 13.99999999999999112 ) ) ;
#78988=DIRECTION ( 'NONE',  ( -0.000000000000000000, -0.000000000000000000, 1.000000000000000000 ) ) ;
#78996=EDGE_CURVE ( 'NONE', #1023, #44839, #28561, .T. ) ;
#78998=EDGE_LOOP ( 'NONE', ( #35731, #10409, #85042, #11599 ) ) ;
#78999=CARTESIAN_POINT ( 'NONE',  ( 195.4524165401237212, 39.48855364940461499, 14.00000000000000000 ) ) ;
#79012=CARTESIAN_POINT ( 'NONE',  ( 196.3790618868739273, 71.92834069484581505, -11.42109594865351774 ) ) ;
#79037=VERTEX_POINT ( 'NONE', #58836 ) ;
#79046=EDGE_CURVE ( 'NONE', #57506, #55010, #64110, .T. ) ;
#79069=CARTESIAN_POINT ( 'NONE',  ( 154.5625123364532101, 249.5000000000000568, 13.15740740740741721 ) ) ;
#79078=CIRCLE ( 'NONE', #38214, 4.999999999999990230 ) ;
#79080=CARTESIAN_POINT ( 'NONE',  ( 200.3186454232214828, 276.0000000000000568, -3.421094783296261710 ) ) ;
#79082=DIRECTION ( 'NONE',  ( -0.000000000000000000, -0.000000000000000000, -1.000000000000000000 ) ) ;
#79092=AXIS2_PLACEMENT_3D ( 'NONE', #14628, #56796, #63435 ) ;
#79098=FACE_OUTER_BOUND ( 'NONE', #82749, .T. ) ;
#79099=FACE_OUTER_BOUND ( 'NONE', #4466, .T. ) ;
#79110=DIRECTION ( 'NONE',  ( 0.000000000000000000, 1.000000000000000000, 0.000000000000000000 ) ) ;
#79111=AXIS2_PLACEMENT_3D ( 'NONE', #74271, #59631, #8930 ) ;
#79119=CIRCLE ( 'NONE', #62420, 0.5000000000000004441 ) ;
#79127=DIRECTION ( 'NONE',  ( -1.000000000000000000, 0.000000000000000000, -0.000000000000000000 ) ) ;
#79138=ORIENTED_EDGE ( 'NONE', *, *, #23136, .T. ) ;
#79141=AXIS2_PLACEMENT_3D ( 'NONE', #61022, #16983, #23149 ) ;
#79144=EDGE_CURVE ( 'NONE', #24392, #86306, #54891, .T. ) ;
#79148=CIRCLE ( 'NONE', #91203, 4.103083949679980691 ) ;
#79150=AXIS2_PLACEMENT_3D ( 'NONE', #76244, #82862, #11376 ) ;
#79155=DIRECTION ( 'NONE',  ( 0.000000000000000000, 0.000000000000000000, 1.000000000000000000 ) ) ;
#79162=AXIS2_PLACEMENT_3D ( 'NONE', #69868, #55206, #10220 ) ;
#79168=ORIENTED_EDGE ( 'NONE', *, *, #53102, .T. ) ;
#79171=CIRCLE ( 'NONE', #27810, 0.4999999999999985567 ) ;
#79182=AXIS2_PLACEMENT_3D ( 'NONE', #53330, #18285, #76051 ) ;
#79193=ORIENTED_EDGE ( 'NONE', *, *, #52823, .T. ) ;
#79200=CARTESIAN_POINT ( 'NONE',  ( 170.2305261370685798, 214.9910457053126720, -24.90909090909089940 ) ) ;
#79208=LINE ( 'NONE', #44116, #39096 ) ;
#79211=CARTESIAN_POINT ( 'NONE',  ( 156.1449889021179160, 249.5000000000000568, 16.91223866672558529 ) ) ;
#79212=DIRECTION ( 'NONE',  ( -1.000000000000000000, 0.000000000000000000, 0.000000000000000000 ) ) ;
#79222=ORIENTED_EDGE ( 'NONE', *, *, #92101, .T. ) ;
#79223=VECTOR ( 'NONE', #71373, 1000.000000000000000 ) ;
#79238=ORIENTED_EDGE ( 'NONE', *, *, #74086, .F. ) ;
#79245=DIRECTION ( 'NONE',  ( 0.000000000000000000, 0.000000000000000000, 1.000000000000000000 ) ) ;
#79247=AXIS2_PLACEMENT_3D ( 'NONE', #57189, #49132, #36316 ) ;
#79259=TOROIDAL_SURFACE ( 'NONE', #62637, 1.500000000000001776, 0.5000000000000000000 ) ;
#79261=VERTEX_POINT ( 'NONE', #44132 ) ;
#79264=ORIENTED_EDGE ( 'NONE', *, *, #49823, .F. ) ;
#79269=EDGE_CURVE ( 'NONE', #93327, #59332, #77224, .T. ) ;
#79282=ORIENTED_EDGE ( 'NONE', *, *, #1109, .T. ) ;
#79289=ORIENTED_EDGE ( 'NONE', *, *, #41709, .F. ) ;
#79297=AXIS2_PLACEMENT_3D ( 'NONE', #1151, #37131, #37578 ) ;
#79303=CARTESIAN_POINT ( 'NONE',  ( 204.6539576904058606, 300.2961574867697436, 4.888549259831427740 ) ) ;
#79306=AXIS2_PLACEMENT_3D ( 'NONE', #3730, #68594, #83243 ) ;
#79326=FACE_OUTER_BOUND ( 'NONE', #21978, .T. ) ;
#79330=CARTESIAN_POINT ( 'NONE',  ( 209.4418336267437439, 29.74545085957678481, 14.26380412667039010 ) ) ;
#79334=TOROIDAL_SURFACE ( 'NONE', #91387, 24.50000000000001066, 0.5000000000000000000 ) ;
#79343=CARTESIAN_POINT ( 'NONE',  ( 209.5577655351089561, 36.99254819693167917, 12.09245862089555423 ) ) ;
#79357=EDGE_CURVE ( 'NONE', #44839, #35945, #17051, .T. ) ;
#79392=CIRCLE ( 'NONE', #17327, 1.499999999999998002 ) ;
#79397=ORIENTED_EDGE ( 'NONE', *, *, #35999, .T. ) ;
#79398=DIRECTION ( 'NONE',  ( 1.000000000000000000, 0.000000000000000000, 0.000000000000000000 ) ) ;
#79399=CARTESIAN_POINT ( 'NONE',  ( 208.6208076322478746, 32.98517505407394168, 15.00000000000000000 ) ) ;
#79406=CARTESIAN_POINT ( 'NONE',  ( 208.4611680579919266, 29.54524714476348279, 14.80559097128782220 ) ) ;
#79410=VERTEX_POINT ( 'NONE', #88147 ) ;
#79426=CARTESIAN_POINT ( 'NONE',  ( 198.4647887804454456, 289.5778437905237297, -6.693278644409265787 ) ) ;
#79436=CARTESIAN_POINT ( 'NONE',  ( 175.2296996224750103, 20.99999999999998934, 0.000000000000000000 ) ) ;
#79452=CARTESIAN_POINT ( 'NONE',  ( 155.4526335419784573, 18.61728136335971229, 8.651974842893862316 ) ) ;
#79454=AXIS2_PLACEMENT_3D ( 'NONE', #61463, #26394, #38713 ) ;
#79457=CARTESIAN_POINT ( 'NONE',  ( 151.0890045490263560, 131.0000000000000568, -11.50000000000000178 ) ) ;
#79467=VERTEX_POINT ( 'NONE', #9070 ) ;
#79468=CARTESIAN_POINT ( 'NONE',  ( 197.1180234003297755, 72.74234001486334478, 12.08831112423764509 ) ) ;
#79470=FACE_OUTER_BOUND ( 'NONE', #64171, .T. ) ;
#79481=DIRECTION ( 'NONE',  ( 1.000000000000000000, 0.000000000000000000, 0.000000000000000000 ) ) ;
#79487=ORIENTED_EDGE ( 'NONE', *, *, #19203, .F. ) ;
#79497=VERTEX_POINT ( 'NONE', #59777 ) ;
#79512=CARTESIAN_POINT ( 'NONE',  ( 157.1811243746104196, 250.0348692542015954, 16.89756558802390529 ) ) ;
#79513=ORIENTED_EDGE ( 'NONE', *, *, #32042, .F. ) ;
#79528=ORIENTED_EDGE ( 'NONE', *, *, #5542, .F. ) ;
#79562=CARTESIAN_POINT ( 'NONE',  ( 154.7381521964376816, 128.4861308677327258, 12.50226176572442860 ) ) ;
#79565=CARTESIAN_POINT ( 'NONE',  ( 197.2511406043087163, 71.96799660027704704, -11.91673342594003060 ) ) ;
#79566=DIRECTION ( 'NONE',  ( -0.8660254037844413721, 0.4999999999999951705, 0.000000000000000000 ) ) ;
#79575=CARTESIAN_POINT ( 'NONE',  ( 186.6539576904058890, 276.0000000000000568, -11.60392986742922439 ) ) ;
#79580=EDGE_CURVE ( 'NONE', #557, #24392, #8619, .T. ) ;
#79584=VECTOR ( 'NONE', #16011, 1000.000000000000000 ) ;
#79618=CARTESIAN_POINT ( 'NONE',  ( 208.4455020912638190, 36.83759663588386246, 13.33594775738876592 ) ) ;
#79624=EDGE_LOOP ( 'NONE', ( #10573, #79744, #59684, #36471 ) ) ;
#79641=DIRECTION ( 'NONE',  ( 0.000000000000000000, -0.000000000000000000, 1.000000000000000000 ) ) ;
#79649=ORIENTED_EDGE ( 'NONE', *, *, #82838, .T. ) ;
#79657=CARTESIAN_POINT ( 'NONE',  ( 196.0143093133015384, 24.42324672360809856, 11.99999999999998934 ) ) ;
#79661=CIRCLE ( 'NONE', #35639, 4.999999999999990230 ) ;
#79664=CARTESIAN_POINT ( 'NONE',  ( 209.6607606054017197, 36.26300151376644010, 14.77867248455306104 ) ) ;
#79669=CARTESIAN_POINT ( 'NONE',  ( 196.0528114083369928, 24.85032509642524090, 13.83578131212104623 ) ) ;
#79670=LINE ( 'NONE', #43666, #38230 ) ;
#79681=CARTESIAN_POINT ( 'NONE',  ( 197.1933712184921603, 24.89666632552609826, 12.64285714285713702 ) ) ;
#79684=EDGE_CURVE ( 'NONE', #66468, #13665, #9450, .T. ) ;
#79692=ORIENTED_EDGE ( 'NONE', *, *, #69946, .T. ) ;
#79696=CARTESIAN_POINT ( 'NONE',  ( 199.5134772723581307, 299.2165499503948922, -6.035833136898175688 ) ) ;
#79699=DIRECTION ( 'NONE',  ( 0.000000000000000000, 0.000000000000000000, 1.000000000000000000 ) ) ;
#79741=ORIENTED_EDGE ( 'NONE', *, *, #40562, .T. ) ;
#79744=ORIENTED_EDGE ( 'NONE', *, *, #42294, .T. ) ;
#79753=CARTESIAN_POINT ( 'NONE',  ( 175.2296996224750103, 276.0000000000000568, 0.000000000000000000 ) ) ;
#79764=DIRECTION ( 'NONE',  ( 0.000000000000000000, 0.000000000000000000, 1.000000000000000000 ) ) ;
#79774=CARTESIAN_POINT ( 'NONE',  ( 210.1640492649794396, 37.84931640281016030, 12.09245862095555601 ) ) ;
#79777=EDGE_CURVE ( 'NONE', #52563, #56772, #53336, .T. ) ;
#79781=EDGE_CURVE ( 'NONE', #91332, #11243, #42808, .T. ) ;
#79826=CIRCLE ( 'NONE', #16356, 2.999999999999997335 ) ;
#79843=FACE_OUTER_BOUND ( 'NONE', #84614, .T. ) ;
#79844=CARTESIAN_POINT ( 'NONE',  ( 196.8803347170859865, 24.42324672360810212, 12.49999999999998757 ) ) ;
#79852=CARTESIAN_POINT ( 'NONE',  ( 152.4536156746142410, 250.0000000000000568, 12.00000000000000000 ) ) ;
#79854=CARTESIAN_POINT ( 'NONE',  ( 165.2424497756046549, 214.5000000000000568, 22.91843887563435800 ) ) ;
#79857=ORIENTED_EDGE ( 'NONE', *, *, #70067, .T. ) ;
#79858=CARTESIAN_POINT ( 'NONE',  ( 201.2104617360081704, 41.21457449016152452, 9.000000000000000000 ) ) ;
#79860=ADVANCED_FACE ( 'NONE', ( #60697 ), #37949, .T. ) ;
#79885=CARTESIAN_POINT ( 'NONE',  ( 140.6539576904058606, 250.5000000000000568, 10.50000000000000000 ) ) ;
#79887=ADVANCED_FACE ( 'NONE', ( #73955 ), #53584, .F. ) ;
#79895=CARTESIAN_POINT ( 'NONE',  ( 207.6243754364163294, 29.64962331212859681, 14.86901082953205666 ) ) ;
#79909=EDGE_CURVE ( 'NONE', #93327, #51424, #90011, .T. ) ;
#79913=CARTESIAN_POINT ( 'NONE',  ( 196.8803347170859865, 73.40565171261609123, 12.49999999999999289 ) ) ;
#79941=ORIENTED_EDGE ( 'NONE', *, *, #73162, .T. ) ;
#79954=CARTESIAN_POINT ( 'NONE',  ( 175.2296996224750103, 160.0000000000000568, 0.000000000000000000 ) ) ;
#79957=CARTESIAN_POINT ( 'NONE',  ( 201.2104617360081704, 15.00000000000000000, -9.000000000000001776 ) ) ;
#79958=CIRCLE ( 'NONE', #67929, 0.5000000000000004441 ) ;
#79959=B_SPLINE_CURVE_WITH_KNOTS ( 'NONE', 3,
 ( #89405, #24559, #53444, #39211, #82327, #17477, #68126, #89882 ),
 .UNSPECIFIED., .F., .F.,
 ( 4, 2, 2, 4 ),
 ( 0.000000000000000000, 0.001862880473700167768, 0.002794320710550249158, 0.003725760947400331199 ),
 .UNSPECIFIED. ) ;
#79973=ORIENTED_EDGE ( 'NONE', *, *, #16723, .F. ) ;
#79989=DIRECTION ( 'NONE',  ( 0.000000000000000000, 0.000000000000000000, 1.000000000000000000 ) ) ;
#79990=CARTESIAN_POINT ( 'NONE',  ( 152.4536156746142410, 250.0000000000000568, 12.50000000000000000 ) ) ;
#79998=DIRECTION ( 'NONE',  ( 0.000000000000000000, 1.000000000000000000, 0.000000000000000000 ) ) ;
#80001=LINE ( 'NONE', #15139, #49003 ) ;
#80003=CARTESIAN_POINT ( 'NONE',  ( 175.2296996224750103, 20.00000000000000000, 0.000000000000000000 ) ) ;
#80015=CARTESIAN_POINT ( 'NONE',  ( 199.7104933562245321, 66.88149622424963070, -10.01660547250589950 ) ) ;
#80016=DIRECTION ( 'NONE',  ( 0.000000000000000000, -1.000000000000000000, -0.000000000000000000 ) ) ;
#80026=ORIENTED_EDGE ( 'NONE', *, *, #58451, .T. ) ;
#80038=ORIENTED_EDGE ( 'NONE', *, *, #1524, .T. ) ;
#80041=DIRECTION ( 'NONE',  ( 0.000000000000000000, 1.000000000000000000, 0.000000000000000000 ) ) ;
#80062=ORIENTED_EDGE ( 'NONE', *, *, #60388, .F. ) ;
#80068=CARTESIAN_POINT ( 'NONE',  ( 165.7865175155837676, 3.000000000000000000, 10.00000000000000000 ) ) ;
#80080=EDGE_LOOP ( 'NONE', ( #71202, #2530 ) ) ;
#80081=DIRECTION ( 'NONE',  ( 0.000000000000000000, 1.000000000000000000, 0.000000000000000000 ) ) ;
#80086=CIRCLE ( 'NONE', #51285, 0.4999999999999941158 ) ;
#80094=AXIS2_PLACEMENT_3D ( 'NONE', #38531, #66953, #58469 ) ;
#80099=EDGE_CURVE ( 'NONE', #21221, #83682, #91168, .T. ) ;
#80108=CARTESIAN_POINT ( 'NONE',  ( 154.4002798831584187, 19.39811195953276624, 12.47990318407953048 ) ) ;
#80116=CARTESIAN_POINT ( 'NONE',  ( 150.4957602436334412, 21.00000000000000000, -3.637614988394445081 ) ) ;
#80119=CARTESIAN_POINT ( 'NONE',  ( 208.7651279064949961, 35.82729677688830350, 14.29018184646296064 ) ) ;
#80120=CARTESIAN_POINT ( 'NONE',  ( 199.0743954165634761, 250.0000000000000568, -2.725891136377211144 ) ) ;
#80129=EDGE_CURVE ( 'NONE', #65802, #83549, #80571, .T. ) ;
#80130=ORIENTED_EDGE ( 'NONE', *, *, #63139, .F. ) ;
#80138=APPLICATION_CONTEXT ( 'automotive_design' ) ;
#80144=ORIENTED_EDGE ( 'NONE', *, *, #71290, .F. ) ;
#80149=CARTESIAN_POINT ( 'NONE',  ( 197.6014737559247578, 297.2619998337689822, -7.302417866276520009 ) ) ;
#80153=DIRECTION ( 'NONE',  ( 0.000000000000000000, 1.000000000000000000, 0.000000000000000000 ) ) ;
#80168=ORIENTED_EDGE ( 'NONE', *, *, #66060, .F. ) ;
#80190=EDGE_CURVE ( 'NONE', #87468, #77289, #11889, .T. ) ;
#80198=VERTEX_POINT ( 'NONE', #25620 ) ;
#80201=ORIENTED_EDGE ( 'NONE', *, *, #47293, .F. ) ;
#80212=EDGE_CURVE ( 'NONE', #48115, #12757, #9461, .T. ) ;
#80223=DIRECTION ( 'NONE',  ( 0.000000000000000000, 1.000000000000000000, 0.000000000000000000 ) ) ;
#80225=CIRCLE ( 'NONE', #19730, 4.999999999999986677 ) ;
#80227=CARTESIAN_POINT ( 'NONE',  ( 196.0143093133015384, 19.33012701892218743, 12.49999999999999112 ) ) ;
#80229=CARTESIAN_POINT ( 'NONE',  ( 219.8344101925596021, 0.000000000000000000, -10.00000000000000000 ) ) ;
#80231=LINE ( 'NONE', #35759, #25469 ) ;
#80235=CARTESIAN_POINT ( 'NONE',  ( 208.6459800967728029, 38.33095280557449769, 12.00000000000000000 ) ) ;
#80286=DIRECTION ( 'NONE',  ( 0.000000000000000000, 0.000000000000000000, 1.000000000000000000 ) ) ;
#80289=TOROIDAL_SURFACE ( 'NONE', #42498, 1.000000000000000000, 0.5000000000000000000 ) ;
#80302=ORIENTED_EDGE ( 'NONE', *, *, #3249, .T. ) ;
#80303=DIRECTION ( 'NONE',  ( 0.000000000000000000, 1.000000000000000000, 0.000000000000000000 ) ) ;
#80309=CARTESIAN_POINT ( 'NONE',  ( 209.4655899500923510, 29.65170969176866933, 14.77867248455306282 ) ) ;
#80310=DIRECTION ( 'NONE',  ( -1.000000000000000000, 0.000000000000000000, 0.000000000000000000 ) ) ;
#80314=FACE_OUTER_BOUND ( 'NONE', #66921, .T. ) ;
#80317=EDGE_CURVE ( 'NONE', #79467, #3893, #74499, .T. ) ;
#80327=DIRECTION ( 'NONE',  ( -0.000000000000000000, 1.000000000000000000, -0.000000000000000000 ) ) ;
#80334=EDGE_CURVE ( 'NONE', #5341, #88648, #67010, .T. ) ;
#80337=SPHERICAL_SURFACE ( 'NONE', #30687, 2.000000000000000000 ) ;
#80344=CARTESIAN_POINT ( 'NONE',  ( 152.4536156746142410, 275.5000000000000568, 14.50000000000000000 ) ) ;
#80351=CARTESIAN_POINT ( 'NONE',  ( 209.1592146219059885, 29.43398993274398734, 14.70257046291166070 ) ) ;
#80367=LINE ( 'NONE', #29735, #75620 ) ;
#80369=CARTESIAN_POINT ( 'NONE',  ( 175.2296996224750103, 133.0000000000000000, -23.00000000000000711 ) ) ;
#80389=FACE_BOUND ( 'NONE', #83214, .T. ) ;
#80394=ORIENTED_EDGE ( 'NONE', *, *, #5869, .F. ) ;
#80410=EDGE_CURVE ( 'NONE', #87519, #77887, #79119, .T. ) ;
#80412=AXIS2_PLACEMENT_3D ( 'NONE', #41520, #25458, #54337 ) ;
#80414=VECTOR ( 'NONE', #63150, 1000.000000000000000 ) ;
#80422=CARTESIAN_POINT ( 'NONE',  ( 199.4894028483730892, 67.51180740859732055, -8.507532329691386508 ) ) ;
#80427=ORIENTED_EDGE ( 'NONE', *, *, #29447, .F. ) ;
#80432=EDGE_CURVE ( 'NONE', #76874, #75355, #68489, .T. ) ;
#80442=CARTESIAN_POINT ( 'NONE',  ( 154.7659666677267580, 19.56018909072084710, -12.94946946941271193 ) ) ;
#80450=DIRECTION ( 'NONE',  ( 0.000000000000000000, 0.000000000000000000, 1.000000000000000000 ) ) ;
#80453=CARTESIAN_POINT ( 'NONE',  ( 152.4536156746142410, 250.0000000000000568, 12.00000000000000000 ) ) ;
#80455=CARTESIAN_POINT ( 'NONE',  ( 175.2296996224750103, 138.1603916158177583, 0.000000000000000000 ) ) ;
#80467=CYLINDRICAL_SURFACE ( 'NONE', #56675, 0.5000000000000004441 ) ;
#80475=CIRCLE ( 'NONE', #51743, 0.5000000000000004441 ) ;
#80476=EDGE_LOOP ( 'NONE', ( #86350, #35455, #15061, #45465 ) ) ;
#80480=FACE_OUTER_BOUND ( 'NONE', #29278, .T. ) ;
#80485=AXIS2_PLACEMENT_3D ( 'NONE', #67778, #37934, #75802 ) ;
#80491=ORIENTED_EDGE ( 'NONE', *, *, #47293, .T. ) ;
#80495=EDGE_CURVE ( 'NONE', #85558, #71226, #11026, .T. ) ;
#80499=DIRECTION ( 'NONE',  ( 1.000000000000000000, 0.000000000000000000, 0.000000000000000000 ) ) ;
#80508=ORIENTED_EDGE ( 'NONE', *, *, #67393, .T. ) ;
#80534=VERTEX_POINT ( 'NONE', #5280 ) ;
#80545=CARTESIAN_POINT ( 'NONE',  ( 160.5350683151633291, 276.0000000000000568, 20.22542485937379908 ) ) ;
#80555=EDGE_CURVE ( 'NONE', #90280, #50719, #26176, .T. ) ;
#80560=EDGE_CURVE ( 'NONE', #81908, #70640, #64073, .T. ) ;
#80563=CARTESIAN_POINT ( 'NONE',  ( 170.2299524499825338, 214.9970011440366875, -24.94063848305468412 ) ) ;
#80569=DIRECTION ( 'NONE',  ( -0.000000000000000000, -0.000000000000000000, 1.000000000000000000 ) ) ;
#80571=CIRCLE ( 'NONE', #89618, 0.4999999999999960587 ) ;
#80572=DIRECTION ( 'NONE',  ( 0.000000000000000000, 0.000000000000000000, 1.000000000000000000 ) ) ;
#80575=DIRECTION ( 'NONE',  ( -0.9893575751536619611, 0.000000000000000000, -0.1455045995357745758 ) ) ;
#80576=CARTESIAN_POINT ( 'NONE',  ( 140.6539576904058606, 0.000000000000000000, 10.50000000000000000 ) ) ;
#80586=CARTESIAN_POINT ( 'NONE',  ( 195.0629117428269126, 293.9636489450776367, -40.00000000000000711 ) ) ;
#80589=CARTESIAN_POINT ( 'NONE',  ( 196.3889435609981149, 25.22386505340214669, 13.78671447301574915 ) ) ;
#80602=CARTESIAN_POINT ( 'NONE',  ( 160.5350683151633291, 249.5000000000000568, 24.72542485937378842 ) ) ;
#80605=DIRECTION ( 'NONE',  ( -0.7453559924999223485, 0.000000000000000000, -0.6666666666666750674 ) ) ;
#80607=CIRCLE ( 'NONE', #14141, 0.5000000000000004441 ) ;
#80612=EDGE_CURVE ( 'NONE', #25728, #29030, #91243, .T. ) ;
#80617=TOROIDAL_SURFACE ( 'NONE', #88174, 4.499999999999986677, 0.5000000000000000000 ) ;
#80622=VERTEX_POINT ( 'NONE', #28452 ) ;
#80625=ORIENTED_EDGE ( 'NONE', *, *, #52172, .T. ) ;
#80639=CIRCLE ( 'NONE', #33744, 0.5000000000000004441 ) ;
#80647=ORIENTED_EDGE ( 'NONE', *, *, #25145, .F. ) ;
#80651=AXIS2_PLACEMENT_3D ( 'NONE', #48797, #75819, #61630 ) ;
#80655=EDGE_LOOP ( 'NONE', ( #62268, #67488 ) ) ;
#80656=DIRECTION ( 'NONE',  ( -0.2156506209390900430, 0.000000000000000000, 0.9764705882352960886 ) ) ;
#80659=ORIENTED_EDGE ( 'NONE', *, *, #6263, .T. ) ;
#80674=PLANE ( 'NONE',  #64181 ) ;
#80683=AXIS2_PLACEMENT_3D ( 'NONE', #55299, #11724, #39183 ) ;
#80687=CIRCLE ( 'NONE', #53454, 1.999999999999988454 ) ;
#80690=DIRECTION ( 'NONE',  ( -0.3024135303179478207, -0.9531768234071973378, 0.000000000000000000 ) ) ;
#80694=DIRECTION ( 'NONE',  ( 0.000000000000000000, 0.000000000000000000, -1.000000000000000000 ) ) ;
#80699=VECTOR ( 'NONE', #12331, 1000.000000000000000 ) ;
#80700=TOROIDAL_SURFACE ( 'NONE', #3579, 25.50000000000000355, 0.5000000000000000000 ) ;
#80709=DIRECTION ( 'NONE',  ( -1.000000000000000000, 0.000000000000000000, 0.000000000000000000 ) ) ;
#80752=CARTESIAN_POINT ( 'NONE',  ( 169.9462594094670180, 276.0000000000000568, -23.92352941176469727 ) ) ;
#80761=AXIS2_PLACEMENT_3D ( 'NONE', #51567, #87545, #942 ) ;
#80768=ORIENTED_EDGE ( 'NONE', *, *, #47322, .F. ) ;
#80769=DIRECTION ( 'NONE',  ( 0.000000000000000000, -0.000000000000000000, 1.000000000000000000 ) ) ;
#80770=TOROIDAL_SURFACE ( 'NONE', #12731, 25.50000000000000355, 0.5000000000000000000 ) ;
#80771=CIRCLE ( 'NONE', #59645, 20.15985230015483154 ) ;
#80811=CARTESIAN_POINT ( 'NONE',  ( 140.6539576904058606, 131.0000000000000568, 11.50000000000000000 ) ) ;
#80820=CARTESIAN_POINT ( 'NONE',  ( 208.2875714627639923, 29.44753873154004964, 14.76836928283343120 ) ) ;
#80823=DIRECTION ( 'NONE',  ( 0.000000000000000000, 0.000000000000000000, 1.000000000000000000 ) ) ;
#80839=DIRECTION ( 'NONE',  ( 0.000000000000000000, -0.000000000000000000, -1.000000000000000000 ) ) ;
#80852=ORIENTED_EDGE ( 'NONE', *, *, #14513, .T. ) ;
#80853=CARTESIAN_POINT ( 'NONE',  ( 195.3198774247918550, 42.06793861907576826, 13.13082619117232497 ) ) ;
#80864=DIRECTION ( 'NONE',  ( 1.000000000000000000, 0.000000000000000000, -0.000000000000000000 ) ) ;
#80874=AXIS2_PLACEMENT_3D ( 'NONE', #43400, #88697, #72295 ) ;
#80885=DIRECTION ( 'NONE',  ( -0.000000000000000000, -1.000000000000000000, -0.000000000000000000 ) ) ;
#80886=CARTESIAN_POINT ( 'NONE',  ( 212.4629471475955427, 32.98517505407394168, 10.00000000000000000 ) ) ;
#80896=SHAPE_REPRESENTATION ( 'Pneumatic Power Actuating Cylinder', ( #18940 ), #37050 ) ;
#80899=VERTEX_POINT ( 'NONE', #13782 ) ;
#80901=DIRECTION ( 'NONE',  ( 0.000000000000000000, 0.000000000000000000, 1.000000000000000000 ) ) ;
#80919=EDGE_CURVE ( 'NONE', #8050, #45887, #42870, .T. ) ;
#80920=VECTOR ( 'NONE', #8898, 1000.000000000000000 ) ;
#80927=CARTESIAN_POINT ( 'NONE',  ( 154.3961680540041073, 19.39715479370783768, 12.47437324411263937 ) ) ;
#80930=DIRECTION ( 'NONE',  ( 0.9998346970812742596, 0.000000000000000000, 0.01818181818181330636 ) ) ;
#80954=ORIENTED_EDGE ( 'NONE', *, *, #80410, .T. ) ;
#80955=CARTESIAN_POINT ( 'NONE',  ( 158.6539576904058606, 276.0000000000000568, -11.60392986742922439 ) ) ;
#80970=DIRECTION ( 'NONE',  ( 0.000000000000000000, 0.000000000000000000, 1.000000000000000000 ) ) ;
#80971=EDGE_CURVE ( 'NONE', #26249, #27568, #89686, .T. ) ;
#80975=DIRECTION ( 'NONE',  ( -0.000000000000000000, -1.000000000000000000, -0.000000000000000000 ) ) ;
#80984=VECTOR ( 'NONE', #48145, 1000.000000000000000 ) ;
#80985=EDGE_LOOP ( 'NONE', ( #63642, #88302 ) ) ;
#81009=ORIENTED_EDGE ( 'NONE', *, *, #66611, .F. ) ;
#81019=CARTESIAN_POINT ( 'NONE',  ( 209.4803090767392462, 35.69423656899339647, 14.26380412667042030 ) ) ;
#81029=EDGE_CURVE ( 'NONE', #63422, #4490, #65559, .T. ) ;
#81033=DIRECTION ( 'NONE',  ( -0.000000000000000000, -0.000000000000000000, 1.000000000000000000 ) ) ;
#81039=CYLINDRICAL_SURFACE ( 'NONE', #89448, 2.000000000000007105 ) ;
#81042=CARTESIAN_POINT ( 'NONE',  ( 200.4025527154073245, 25.63806215016873580, 10.01693176487371240 ) ) ;
#81045=CARTESIAN_POINT ( 'NONE',  ( 201.0592549708491958, 40.73798607845792219, 10.49999999999999822 ) ) ;
#81060=DIRECTION ( 'NONE',  ( -0.000000000000000000, -1.000000000000000000, -0.000000000000000000 ) ) ;
#81072=FACE_OUTER_BOUND ( 'NONE', #27431, .T. ) ;
#81073=EDGE_CURVE ( 'NONE', #82490, #89945, #42157, .T. ) ;
#81090=EDGE_LOOP ( 'NONE', ( #29421, #80427, #54892, #20239 ) ) ;
#81096=EDGE_CURVE ( 'NONE', #2308, #83547, #56490, .T. ) ;
#81104=ORIENTED_EDGE ( 'NONE', *, *, #67389, .T. ) ;
#81114=EDGE_LOOP ( 'NONE', ( #7175, #55842, #29985, #45546, #61096, #36611 ) ) ;
#81125=ORIENTED_EDGE ( 'NONE', *, *, #39601, .T. ) ;
#81136=CARTESIAN_POINT ( 'NONE',  ( 193.8739039770516968, 214.6009552038330526, 16.65543863426445270 ) ) ;
#81141=CARTESIAN_POINT ( 'NONE',  ( 207.6662022560301182, 36.29800326561209545, 14.90057469441957316 ) ) ;
#81148=CARTESIAN_POINT ( 'NONE',  ( 140.6539576904058606, 250.5000000000000568, 12.00000000000000000 ) ) ;
#81151=CARTESIAN_POINT ( 'NONE',  ( 152.2747007761510076, 129.8137010776104603, 12.50000000000000178 ) ) ;
#81153=CARTESIAN_POINT ( 'NONE',  ( 155.0741174296533984, 18.62644422905990638, -11.41100038915083914 ) ) ;
#81171=CARTESIAN_POINT ( 'NONE',  ( 152.4536156746142410, 250.5000000000000568, -14.50000000000000000 ) ) ;
#81174=DIRECTION ( 'NONE',  ( -0.000000000000000000, -1.000000000000000000, -0.000000000000000000 ) ) ;
#81203=ORIENTED_EDGE ( 'NONE', *, *, #6509, .F. ) ;
#81212=CARTESIAN_POINT ( 'NONE',  ( 175.2296996224750103, 250.0000000000000568, 0.000000000000000000 ) ) ;
#81225=VERTEX_POINT ( 'NONE', #72025 ) ;
#81226=DIRECTION ( 'NONE',  ( 0.000000000000000000, 0.000000000000000000, -1.000000000000000000 ) ) ;
#81232=DIRECTION ( 'NONE',  ( 0.000000000000000000, 0.000000000000000000, 1.000000000000000000 ) ) ;
#81233=FACE_BOUND ( 'NONE', #71970, .T. ) ;
#81239=CARTESIAN_POINT ( 'NONE',  ( 185.2519943799831879, 3.000000000000000000, 10.00000000000000000 ) ) ;
#81252=ADVANCED_FACE ( 'NONE', ( #57347 ), #86187, .F. ) ;
#81253=EDGE_CURVE ( 'NONE', #60748, #50317, #21339, .T. ) ;
#81254=CARTESIAN_POINT ( 'NONE',  ( 209.3463262141449661, 1.051285333831499136, -7.457902384259533335 ) ) ;
#81264=CARTESIAN_POINT ( 'NONE',  ( 199.0143093133015668, 16.83012701892219098, 9.999999999999998224 ) ) ;
#81269=DIRECTION ( 'NONE',  ( -0.000000000000000000, -1.000000000000000000, -0.000000000000000000 ) ) ;
#81272=DIRECTION ( 'NONE',  ( 0.000000000000000000, 1.000000000000000000, -0.000000000000000000 ) ) ;
#81295=ORIENTED_EDGE ( 'NONE', *, *, #80971, .T. ) ;
#81296=CARTESIAN_POINT ( 'NONE',  ( 197.9840890846857349, 69.90067952545793162, 11.10260959755656174 ) ) ;
#81298=DIRECTION ( 'NONE',  ( -0.000000000000000000, -1.000000000000000000, -0.000000000000000000 ) ) ;
#81307=ORIENTED_EDGE ( 'NONE', *, *, #64718, .T. ) ;
#81321=ORIENTED_EDGE ( 'NONE', *, *, #3347, .T. ) ;
#81335=CARTESIAN_POINT ( 'NONE',  ( 164.2231345125756263, 300.2961574867697436, 7.500000000000000000 ) ) ;
#81347=CARTESIAN_POINT ( 'NONE',  ( 207.0561972617101674, 35.35788477359428583, 15.00000000000000178 ) ) ;
#81353=CARTESIAN_POINT ( 'NONE',  ( 196.8865788344860164, 19.32388290151324028, -12.43054049969427588 ) ) ;
#81369=CARTESIAN_POINT ( 'NONE',  ( 155.7140808774800007, 20.99999999999999645, -15.62500000000000711 ) ) ;
#81377=DIRECTION ( 'NONE',  ( 0.000000000000000000, 0.000000000000000000, -1.000000000000000000 ) ) ;
#81381=DIRECTION ( 'NONE',  ( 0.000000000000000000, 0.000000000000000000, 1.000000000000000000 ) ) ;
#81390=CARTESIAN_POINT ( 'NONE',  ( 205.7786681169002350, 32.98517505407394168, 10.00000000000000000 ) ) ;
#81393=CYLINDRICAL_SURFACE ( 'NONE', #77889, 0.9999999999999991118 ) ;
#81404=FACE_OUTER_BOUND ( 'NONE', #18705, .T. ) ;
#81424=DIRECTION ( 'NONE',  ( 0.000000000000000000, 1.000000000000000000, 0.000000000000000000 ) ) ;
#81432=( BOUNDED_CURVE ( )  B_SPLINE_CURVE ( 3, ( #69772, #3976, #77344, #61740 ),
 .UNSPECIFIED., .F., .F. ) 
 B_SPLINE_CURVE_WITH_KNOTS ( ( 4, 4 ),
 ( 3.141592653589793116, 4.712388980384689674 ),
 .UNSPECIFIED. ) 
 CURVE ( )  GEOMETRIC_REPRESENTATION_ITEM ( )  RATIONAL_B_SPLINE_CURVE ( ( 1.000000000000000000, 0.8047378541243649375, 0.8047378541243649375, 1.000000000000000000 ) ) 
 REPRESENTATION_ITEM ( '' )  );
#81436=( BOUNDED_SURFACE ( )  B_SPLINE_SURFACE ( 3, 2, ( 
 ( #50195, #28901, #57789 ),
 ( #53924, #53457, #82792 ),
 ( #10355, #40157, #45397 ),
 ( #9420, #60117, #23651 ) ),
 .UNSPECIFIED., .F., .F., .F. ) 
 B_SPLINE_SURFACE_WITH_KNOTS ( ( 4, 4 ),
 ( 3, 3 ),
 ( -1.728218262941894068E-16, 0.0009404805950306077342 ),
 ( 0.000000000000000000, 1.000000000000000000 ),
 .UNSPECIFIED. ) 
 GEOMETRIC_REPRESENTATION_ITEM ( )  RATIONAL_B_SPLINE_SURFACE ( (
 ( 1.000000000000000000, 0.6287211027134009811, 1.000000000000000000),
 ( 1.000000000000000000, 0.6575897825471116453, 1.000000000000000000),
 ( 1.000000000000000000, 0.6851250445827015145, 1.000000000000000000),
 ( 1.000000000000000000, 0.7071067811865358044, 1.000000000000000000) ) ) 
 REPRESENTATION_ITEM ( '' )  SURFACE ( )  );
#81443=ORIENTED_EDGE ( 'NONE', *, *, #40562, .F. ) ;
#81450=CARTESIAN_POINT ( 'NONE',  ( 199.1087447750284980, 64.61450673763175701, 10.46317447812566570 ) ) ;
#81461=ORIENTED_EDGE ( 'NONE', *, *, #78636, .T. ) ;
#81481=ADVANCED_FACE ( 'NONE', ( #38323 ), #61005, .F. ) ;
#81486=CARTESIAN_POINT ( 'NONE',  ( 196.4644011024695658, 24.42492343596410365, 11.30625710096401093 ) ) ;
#81492=DIRECTION ( 'NONE',  ( -0.000000000000000000, -0.000000000000000000, 1.000000000000000000 ) ) ;
#81511=CARTESIAN_POINT ( 'NONE',  ( 196.1984952657759038, 25.39230566755399821, 14.04035613084743339 ) ) ;
#81540=ORIENTED_EDGE ( 'NONE', *, *, #54222, .T. ) ;
#81550=AXIS2_PLACEMENT_3D ( 'NONE', #37046, #2916, #65958 ) ;
#81576=ORIENTED_EDGE ( 'NONE', *, *, #8605, .F. ) ;
#81578=EDGE_CURVE ( 'NONE', #36174, #79410, #17115, .T. ) ;
#81589=CARTESIAN_POINT ( 'NONE',  ( 211.4629471475955427, 32.98517505407394168, 10.00000000000000000 ) ) ;
#81592=DIRECTION ( 'NONE',  ( -0.000000000000000000, -0.000000000000000000, 1.000000000000000000 ) ) ;
#81595=DIRECTION ( 'NONE',  ( -0.000000000000000000, -0.000000000000000000, 1.000000000000000000 ) ) ;
#81598=EDGE_CURVE ( 'NONE', #47569, #443, #67691, .T. ) ;
#81603=DIRECTION ( 'NONE',  ( 0.000000000000000000, 0.000000000000000000, 1.000000000000000000 ) ) ;
#81604=CARTESIAN_POINT ( 'NONE',  ( 194.3594574420116317, 20.00000000000002842, 14.58911678380875010 ) ) ;
#81607=CARTESIAN_POINT ( 'NONE',  ( 165.2494399300530290, 8.542400036368780647, -9.000000000000001776 ) ) ;
#81615=CARTESIAN_POINT ( 'NONE',  ( 209.5561215397301282, 38.04219307066034617, 12.07126757350762247 ) ) ;
#81622=TOROIDAL_SURFACE ( 'NONE', #10588, 27.00000000000000355, 2.000000000000000000 ) ;
#81626=CIRCLE ( 'NONE', #51416, 0.5000000000000004441 ) ;
#81631=CARTESIAN_POINT ( 'NONE',  ( 152.1970149279871976, 130.7370361098515446, -11.50000000000000000 ) ) ;
#81649=CARTESIAN_POINT ( 'NONE',  ( 152.4536156746142410, 249.5000000000000568, -14.50000000000000000 ) ) ;
#81666=EDGE_CURVE ( 'NONE', #89341, #10071, #74310, .T. ) ;
#81671=CARTESIAN_POINT ( 'NONE',  ( 138.6539576904058606, 275.0000000000000568, 10.50000000000000000 ) ) ;
#81685=CARTESIAN_POINT ( 'NONE',  ( 199.4392256788250677, 65.82574266882504332, -7.741079165001071516 ) ) ;
#81687=VECTOR ( 'NONE', #37181, 1000.000000000000000 ) ;
#81691=VECTOR ( 'NONE', #86401, 1000.000000000000000 ) ;
#81698=EDGE_LOOP ( 'NONE', ( #51037, #86686, #5891, #63223 ) ) ;
#81699=DIRECTION ( 'NONE',  ( 1.000000000000000000, 0.000000000000000000, 0.000000000000000000 ) ) ;
#81712=CARTESIAN_POINT ( 'NONE',  ( 153.6987871352777404, 19.48326534539592458, 11.45812909364015297 ) ) ;
#81715=EDGE_CURVE ( 'NONE', #81225, #90630, #53408, .T. ) ;
#81723=DIRECTION ( 'NONE',  ( 0.000000000000000000, 0.000000000000000000, 1.000000000000000000 ) ) ;
#81728=EDGE_CURVE ( 'NONE', #21852, #63583, #37394, .T. ) ;
#81729=DIRECTION ( 'NONE',  ( 0.000000000000000000, 1.000000000000000000, 0.000000000000000000 ) ) ;
#81770=FACE_OUTER_BOUND ( 'NONE', #28143, .T. ) ;
#81779=DIRECTION ( 'NONE',  ( -1.000000000000000000, 0.000000000000000000, -0.000000000000000000 ) ) ;
#81784=ORIENTED_EDGE ( 'NONE', *, *, #742, .T. ) ;
#81790=EDGE_CURVE ( 'NONE', #77618, #43923, #2819, .T. ) ;
#81812=DIRECTION ( 'NONE',  ( 0.000000000000000000, 0.000000000000000000, 1.000000000000000000 ) ) ;
#81816=ORIENTED_EDGE ( 'NONE', *, *, #28179, .F. ) ;
#81817=EDGE_LOOP ( 'NONE', ( #84340, #62402, #91597, #58198, #71729, #44037, #47488, #10995, #19958, #30714, #25524, #6203, #72608, #58276, #8682, #58741, #10590, #72387, #82730, #67233, #55982, #8567, #93127, #70890, #34895, #40116 ) ) ;
#81818=CARTESIAN_POINT ( 'NONE',  ( 195.0811277904324754, 39.36132622696000283, 15.19607843137254477 ) ) ;
#81829=AXIS2_PLACEMENT_3D ( 'NONE', #63620, #71170, #50778 ) ;
#81833=CARTESIAN_POINT ( 'NONE',  ( 201.2104617360081704, 15.00000000000000000, -9.000000000000001776 ) ) ;
#81841=DIRECTION ( 'NONE',  ( 0.000000000000000000, 1.000000000000000000, 0.000000000000000000 ) ) ;
#81845=CARTESIAN_POINT ( 'NONE',  ( 175.2296996224750103, 249.5000000000000568, 24.50000000000000355 ) ) ;
#81856=ADVANCED_FACE ( 'NONE', ( #80480 ), #8971, .F. ) ;
#81858=DIRECTION ( 'NONE',  ( 0.5068419345592596326, 0.000000000000000000, 0.8620390091940313138 ) ) ;
#81883=DIRECTION ( 'NONE',  ( -0.000000000000000000, -1.000000000000000000, -0.000000000000000000 ) ) ;
#81885=CARTESIAN_POINT ( 'NONE',  ( 175.2296996224750103, 214.5000000000000568, 0.000000000000000000 ) ) ;
#81889=CARTESIAN_POINT ( 'NONE',  ( 154.1407330040854333, 250.0000000000000568, 13.42592592592592915 ) ) ;
#81890=AXIS2_PLACEMENT_3D ( 'NONE', #11521, #4884, #84408 ) ;
#81893=ADVANCED_FACE ( 'NONE', ( #58730 ), #31245, .F. ) ;
#81904=B_SPLINE_CURVE_WITH_KNOTS ( 'NONE', 3,
 ( #19554, #49379, #13411, #42254, #6296, #55557, #91979, #49831 ),
 .UNSPECIFIED., .F., .F.,
 ( 4, 2, 2, 4 ),
 ( 0.000000000000000000, 0.0002353609534302478071, 0.0004707219068604956143, 0.0009414438137210617017 ),
 .UNSPECIFIED. ) ;
#81907=ORIENTED_EDGE ( 'NONE', *, *, #15556, .T. ) ;
#81908=VERTEX_POINT ( 'NONE', #59191 ) ;
#81925=ORIENTED_EDGE ( 'NONE', *, *, #909, .T. ) ;
#81926=FACE_OUTER_BOUND ( 'NONE', #64879, .T. ) ;
#81935=CARTESIAN_POINT ( 'NONE',  ( 207.9723288469463114, 36.44590423839540705, 14.83890152313991706 ) ) ;
#81947=FACE_OUTER_BOUND ( 'NONE', #7511, .T. ) ;
#81948=AXIS2_PLACEMENT_3D ( 'NONE', #52255, #89153, #30483 ) ;
#81951=TOROIDAL_SURFACE ( 'NONE', #56310, 24.50000000000000355, 0.5000000000000000000 ) ;
#81957=CIRCLE ( 'NONE', #21502, 7.999911143031724237 ) ;
#81959=DIRECTION ( 'NONE',  ( -0.000000000000000000, -1.000000000000000000, -0.000000000000000000 ) ) ;
#81962=CARTESIAN_POINT ( 'NONE',  ( 200.1126601882107252, 214.5000000000000568, -2.416251949619908856 ) ) ;
#81973=CARTESIAN_POINT ( 'NONE',  ( 156.4851178187871312, 15.00000000000000000, -7.000000000000000888 ) ) ;
#81981=( BOUNDED_CURVE ( )  B_SPLINE_CURVE ( 3, ( #46015, #10030, #16220, #82473 ),
 .UNSPECIFIED., .F., .F. ) 
 B_SPLINE_CURVE_WITH_KNOTS ( ( 4, 4 ),
 ( 0.000000000000000000, 0.5235987755982975944 ),
 .UNSPECIFIED. ) 
 CURVE ( )  GEOMETRIC_REPRESENTATION_ITEM ( )  RATIONAL_B_SPLINE_CURVE ( ( 1.000000000000000000, 0.9772838841927122822, 0.9772838841927122822, 1.000000000000000000 ) ) 
 REPRESENTATION_ITEM ( '' )  );
#81988=( BOUNDED_CURVE ( )  B_SPLINE_CURVE ( 3, ( #62304, #55672, #32009, #89754 ),
 .UNSPECIFIED., .F., .F. ) 
 B_SPLINE_CURVE_WITH_KNOTS ( ( 4, 4 ),
 ( 4.278565243615664038, 4.712388980384691450 ),
 .UNSPECIFIED. ) 
 CURVE ( )  GEOMETRIC_REPRESENTATION_ITEM ( )  RATIONAL_B_SPLINE_CURVE ( ( 1.000000000000000000, 0.9843778111405747655, 0.9843778111405747655, 1.000000000000000000 ) ) 
 REPRESENTATION_ITEM ( '' )  );
#81990=CARTESIAN_POINT ( 'NONE',  ( 156.4677141125678475, 15.48129629386925643, 7.027845929950953696 ) ) ;
#82011=ORIENTED_EDGE ( 'NONE', *, *, #7720, .F. ) ;
#82014=EDGE_CURVE ( 'NONE', #4883, #47327, #67070, .T. ) ;
#82028=CARTESIAN_POINT ( 'NONE',  ( 150.6539576904058606, 293.9636489450775230, 0.000000000000000000 ) ) ;
#82036=CIRCLE ( 'NONE', #33649, 4.499999999999990230 ) ;
#82043=CARTESIAN_POINT ( 'NONE',  ( 157.4851178187871312, 15.28877977928702236, 6.999999999998999023 ) ) ;
#82058=CARTESIAN_POINT ( 'NONE',  ( 193.8056763105550147, 214.8829733828359849, 16.96953521546779697 ) ) ;
#82062=AXIS2_PLACEMENT_3D ( 'NONE', #73509, #24222, #39340 ) ;
#82069=CARTESIAN_POINT ( 'NONE',  ( 154.1772290835186539, 20.65814982784575449, 13.49254024716540812 ) ) ;
#82070=CARTESIAN_POINT ( 'NONE',  ( 160.6539576904058606, 293.9636489450775230, 0.000000000000000000 ) ) ;
#82073=CARTESIAN_POINT ( 'NONE',  ( 165.0427047786672290, 215.0000000000000568, 23.37680765314704701 ) ) ;
#82075=CARTESIAN_POINT ( 'NONE',  ( 157.9772837799833383, 17.93151222991821214, -10.94239627425337602 ) ) ;
#82086=AXIS2_PLACEMENT_3D ( 'NONE', #92792, #930, #87084 ) ;
#82095=LINE ( 'NONE', #60809, #71188 ) ;
#82097=VECTOR ( 'NONE', #3368, 1000.000000000000000 ) ;
#82122=AXIS2_PLACEMENT_3D ( 'NONE', #82208, #17363, #75118 ) ;
#82132=AXIS2_PLACEMENT_3D ( 'NONE', #17023, #67237, #29847 ) ;
#82134=ORIENTED_EDGE ( 'NONE', *, *, #11662, .F. ) ;
#82136=VERTEX_POINT ( 'NONE', #10369 ) ;
#82147=ADVANCED_FACE ( 'NONE', ( #15630 ), #17956, .T. ) ;
#82159=ORIENTED_EDGE ( 'NONE', *, *, #44158, .T. ) ;
#82163=AXIS2_PLACEMENT_3D ( 'NONE', #66356, #44554, #1937 ) ;
#82167=CARTESIAN_POINT ( 'NONE',  ( 198.6884013828325521, 64.61450673763174279, -9.555809373750800972 ) ) ;
#82169=CIRCLE ( 'NONE', #41335, 24.00000000000000355 ) ;
#82174=CARTESIAN_POINT ( 'NONE',  ( 197.2644541368101159, 214.9596432740807757, -12.42446933126076480 ) ) ;
#82175=CIRCLE ( 'NONE', #15691, 24.00000000000001066 ) ;
#82186=VECTOR ( 'NONE', #64345, 1000.000000000000000 ) ;
#82190=CARTESIAN_POINT ( 'NONE',  ( 153.4178427586908811, 19.62198520651892863, 10.83765028963029842 ) ) ;
#82203=EDGE_CURVE ( 'NONE', #75996, #64501, #70019, .T. ) ;
#82205=PLANE ( 'NONE',  #87905 ) ;
#82208=CARTESIAN_POINT ( 'NONE',  ( 175.2296996224750103, 250.5000000000000568, 0.000000000000000000 ) ) ;
#82212=ORIENTED_EDGE ( 'NONE', *, *, #90310, .F. ) ;
#82216=CARTESIAN_POINT ( 'NONE',  ( 193.9535050655732675, 215.0000000000000568, 17.26454883540666430 ) ) ;
#82219=FACE_OUTER_BOUND ( 'NONE', #14667, .T. ) ;
#82232=EDGE_LOOP ( 'NONE', ( #66313, #75178, #84836, #50623 ) ) ;
#82234=CIRCLE ( 'NONE', #12718, 0.5000000000000004441 ) ;
#82242=CIRCLE ( 'NONE', #53526, 3.842139515347647638 ) ;
#82246=ORIENTED_EDGE ( 'NONE', *, *, #88732, .T. ) ;
#82247=DIRECTION ( 'NONE',  ( 1.000000000000000000, 0.000000000000000000, 0.000000000000000000 ) ) ;
#82257=CARTESIAN_POINT ( 'NONE',  ( 165.0427047786672290, 250.5000000000000568, 23.37680765314704701 ) ) ;
#82258=AXIS2_PLACEMENT_3D ( 'NONE', #15701, #569, #44563 ) ;
#82259=CARTESIAN_POINT ( 'NONE',  ( 152.4536156746142410, 130.6065089285656313, 11.50000000000000000 ) ) ;
#82263=ORIENTED_EDGE ( 'NONE', *, *, #7928, .F. ) ;
#82272=EDGE_CURVE ( 'NONE', #87519, #44024, #76129, .T. ) ;
#82273=VERTEX_POINT ( 'NONE', #39696 ) ;
#82278=DIRECTION ( 'NONE',  ( -0.000000000000000000, -1.000000000000000000, -0.000000000000000000 ) ) ;
#82280=EDGE_CURVE ( 'NONE', #38685, #80899, #76187, .T. ) ;
#82283=DIRECTION ( 'NONE',  ( -1.000000000000000000, 0.000000000000000000, 0.000000000000000000 ) ) ;
#82294=ORIENTED_EDGE ( 'NONE', *, *, #27622, .F. ) ;
#82306=AXIS2_PLACEMENT_3D ( 'NONE', #44215, #81595, #73122 ) ;
#82311=CARTESIAN_POINT ( 'NONE',  ( 208.6208076322478746, 32.98517505407394168, 15.00000000000000000 ) ) ;
#82312=AXIS2_PLACEMENT_3D ( 'NONE', #11293, #76629, #54832 ) ;
#82323=CIRCLE ( 'NONE', #15759, 4.103083949679980691 ) ;
#82327=CARTESIAN_POINT ( 'NONE',  ( 195.4048939377254612, 20.66407592107141511, 13.00192971195525260 ) ) ;
#82335=AXIS2_PLACEMENT_3D ( 'NONE', #58290, #80041, #28008 ) ;
#82338=CARTESIAN_POINT ( 'NONE',  ( 209.7513585654922679, 305.7026273589066818, -40.00000000000000711 ) ) ;
#82348=ORIENTED_EDGE ( 'NONE', *, *, #78116, .T. ) ;
#82349=CARTESIAN_POINT ( 'NONE',  ( 175.2296996224750103, 247.0000000000001137, 0.000000000000000000 ) ) ;
#82352=CARTESIAN_POINT ( 'NONE',  ( 164.2231345125756263, 264.6571197653884155, -7.500000000000000000 ) ) ;
#82366=DIRECTION ( 'NONE',  ( 0.4999999999999966693, 0.8660254037844405950, 0.000000000000000000 ) ) ;
#82367=ORIENTED_EDGE ( 'NONE', *, *, #33815, .T. ) ;
#82370=CARTESIAN_POINT ( 'NONE',  ( 196.0143093133015384, 20.19615242270663913, -11.99999999999998579 ) ) ;
#82371=CARTESIAN_POINT ( 'NONE',  ( 195.4790382475684680, 26.04803379143200104, 14.66351318240304558 ) ) ;
#82379=VERTEX_POINT ( 'NONE', #77588 ) ;
#82383=VECTOR ( 'NONE', #80016, 1000.000000000000000 ) ;
#82390=ORIENTED_EDGE ( 'NONE', *, *, #51997, .T. ) ;
#82391=EDGE_LOOP ( 'NONE', ( #71192, #27191, #80062, #74102 ) ) ;
#82396=CARTESIAN_POINT ( 'NONE',  ( 197.7672738693491965, 26.00182986903273274, 10.01345434887959662 ) ) ;
#82404=AXIS2_PLACEMENT_3D ( 'NONE', #39166, #89836, #68078 ) ;
#82408=EDGE_LOOP ( 'NONE', ( #32526, #38468, #54561, #31241 ) ) ;
#82428=CARTESIAN_POINT ( 'NONE',  ( 154.7659666677267580, 19.56018909072085066, 12.94946946941272437 ) ) ;
#82430=CARTESIAN_POINT ( 'NONE',  ( 211.1232656141943949, 0.000000000000000000, 7.000000000000000000 ) ) ;
#82436=EDGE_CURVE ( 'NONE', #48386, #52785, #59510, .T. ) ;
#82441=CARTESIAN_POINT ( 'NONE',  ( 195.4048939377254612, 20.66407592107141511, -13.00192971195525260 ) ) ;
#82444=CARTESIAN_POINT ( 'NONE',  ( 197.8829252751895069, 41.74573726702125498, 11.20279836830544795 ) ) ;
#82445=DIRECTION ( 'NONE',  ( 0.000000000000000000, 0.000000000000000000, 1.000000000000000000 ) ) ;
#82463=VECTOR ( 'NONE', #92636, 1000.000000000000000 ) ;
#82470=CARTESIAN_POINT ( 'NONE',  ( 156.1243321211828743, 16.88031981475914023, 7.577257116167345430 ) ) ;
#82473=CARTESIAN_POINT ( 'NONE',  ( 196.0143093133015384, 73.40565171261609123, -11.99999999999998046 ) ) ;
#82490=VERTEX_POINT ( 'NONE', #68621 ) ;
#82513=B_SPLINE_CURVE_WITH_KNOTS ( 'NONE', 3,
 ( #72510, #62027, #24158, #60173, #68197, #68666, #53520, #32206 ),
 .UNSPECIFIED., .F., .F.,
 ( 4, 2, 2, 4 ),
 ( 0.0006959094422096703380, 0.002907332141605427356, 0.005118754841001184157, 0.009541600239792700361 ),
 .UNSPECIFIED. ) ;
#82519=ORIENTED_EDGE ( 'NONE', *, *, #51459, .F. ) ;
#82520=CARTESIAN_POINT ( 'NONE',  ( 150.6539576904058606, 293.9636489450775230, 0.000000000000000000 ) ) ;
#82524=ORIENTED_EDGE ( 'NONE', *, *, #59598, .T. ) ;
#82535=CARTESIAN_POINT ( 'NONE',  ( 179.7289557593406357, 249.5000000000000568, -24.91818181818183575 ) ) ;
#82539=CARTESIAN_POINT ( 'NONE',  ( 208.4306832106271656, 1.063508326895939327, -7.500000000000014211 ) ) ;
#82545=CARTESIAN_POINT ( 'NONE',  ( 209.5770068336137797, 1.043152431597804020, 7.415392722555408156 ) ) ;
#82549=EDGE_CURVE ( 'NONE', #8050, #64275, #10560, .T. ) ;
#82552=ORIENTED_EDGE ( 'NONE', *, *, #66060, .T. ) ;
#82553=CARTESIAN_POINT ( 'NONE',  ( 156.3466120839444216, 16.19322481500736188, -7.221609175748793241 ) ) ;
#82555=DIRECTION ( 'NONE',  ( 1.000000000000000000, 0.000000000000000000, 0.000000000000000000 ) ) ;
#82558=CARTESIAN_POINT ( 'NONE',  ( 157.2832821354339501, 16.68119283998691316, -9.201835683359409046 ) ) ;
#82572=ORIENTED_EDGE ( 'NONE', *, *, #28796, .T. ) ;
#82574=CARTESIAN_POINT ( 'NONE',  ( 197.5016171081239236, 69.66454985082778251, 11.63779655374072242 ) ) ;
#82591=DIRECTION ( 'NONE',  ( 0.000000000000000000, 0.000000000000000000, 1.000000000000000000 ) ) ;
#82604=EDGE_LOOP ( 'NONE', ( #69033, #75612, #38583, #87004 ) ) ;
#82626=ORIENTED_EDGE ( 'NONE', *, *, #91723, .F. ) ;
#82632=CARTESIAN_POINT ( 'NONE',  ( 198.3009384528458270, 65.29331921385960413, -9.735304354939227522 ) ) ;
#82641=EDGE_CURVE ( 'NONE', #77260, #19571, #74823, .T. ) ;
#82652=CARTESIAN_POINT ( 'NONE',  ( 198.0297899315801260, 67.77535909854674401, 9.842341523430512495 ) ) ;
#82666=CARTESIAN_POINT ( 'NONE',  ( 196.8803347170859865, 20.19615242270636557, -12.49999999999999289 ) ) ;
#82678=CYLINDRICAL_SURFACE ( 'NONE', #54130, 5.568361562975243650 ) ;
#82681=FACE_OUTER_BOUND ( 'NONE', #1104, .T. ) ;
#82695=CARTESIAN_POINT ( 'NONE',  ( 201.2104617360081704, 41.21457449016152452, 9.000000000000000000 ) ) ;
#82707=ORIENTED_EDGE ( 'NONE', *, *, #35999, .F. ) ;
#82708=CARTESIAN_POINT ( 'NONE',  ( 153.9133111279456045, 20.47222690886501795, -13.06183683676589524 ) ) ;
#82717=CARTESIAN_POINT ( 'NONE',  ( 196.2176501911084472, 72.73677621079856692, 11.64780326838285873 ) ) ;
#82721=ORIENTED_EDGE ( 'NONE', *, *, #22274, .F. ) ;
#82730=ORIENTED_EDGE ( 'NONE', *, *, #35371, .F. ) ;
#82747=CARTESIAN_POINT ( 'NONE',  ( 156.9431851590352665, 249.5000000000000568, 17.51463615629799975 ) ) ;
#82749=EDGE_LOOP ( 'NONE', ( #82134, #7931, #84568 ) ) ;
#82750=ORIENTED_EDGE ( 'NONE', *, *, #3777, .T. ) ;
#82751=DIRECTION ( 'NONE',  ( -1.000000000000000000, 0.000000000000000000, 0.000000000000000000 ) ) ;
#82755=EDGE_CURVE ( 'NONE', #72640, #74021, #55351, .T. ) ;
#82759=B_SPLINE_CURVE_WITH_KNOTS ( 'NONE', 3,
 ( #68150, #10832, #26460, #39233 ),
 .UNSPECIFIED., .F., .F.,
 ( 4, 4 ),
 ( 3.469446951953613804E-18, 0.0008421770481696917027 ),
 .UNSPECIFIED. ) ;
#82767=DIRECTION ( 'NONE',  ( 0.000000000000000000, 0.000000000000000000, -1.000000000000000000 ) ) ;
#82768=CARTESIAN_POINT ( 'NONE',  ( 195.4583199688989339, 39.99286515677976439, 13.91341927790974431 ) ) ;
#82792=CARTESIAN_POINT ( 'NONE',  ( 207.1704462279909649, 29.87979000412345698, 14.95737379494775077 ) ) ;
#82803=CARTESIAN_POINT ( 'NONE',  ( 197.8477145984406889, 64.61450673763175701, -7.741079165001063522 ) ) ;
#82805=CARTESIAN_POINT ( 'NONE',  ( 175.2296996224750103, 149.6461846693799487, 24.00000000000001066 ) ) ;
#82813=ORIENTED_EDGE ( 'NONE', *, *, #80432, .T. ) ;
#82817=CARTESIAN_POINT ( 'NONE',  ( 199.2296996224750103, 68.12454877777268791, -4.263256414560601746E-14 ) ) ;
#82823=CARTESIAN_POINT ( 'NONE',  ( 196.9534188175200029, 25.84350552936208700, 12.42857142857141817 ) ) ;
#82824=CARTESIAN_POINT ( 'NONE',  ( 199.9311642430735105, 312.1715086799357550, 9.103929867429130240 ) ) ;
#82838=EDGE_CURVE ( 'NONE', #59807, #55580, #53936, .T. ) ;
#82843=ORIENTED_EDGE ( 'NONE', *, *, #43223, .F. ) ;
#82844=AXIS2_PLACEMENT_3D ( 'NONE', #27265, #55685, #78397 ) ;
#82845=CARTESIAN_POINT ( 'NONE',  ( 185.8264795993290193, 275.0000000000000568, 23.09031830825835385 ) ) ;
#82861=VERTEX_POINT ( 'NONE', #34505 ) ;
#82862=DIRECTION ( 'NONE',  ( -0.000000000000000000, -1.000000000000000000, -0.000000000000000000 ) ) ;
#82870=CARTESIAN_POINT ( 'NONE',  ( 209.0052894622294843, 36.56177042507920305, 14.71714099304908885 ) ) ;
#82880=CARTESIAN_POINT ( 'NONE',  ( 201.2104617360081704, 250.0000000000000568, -15.00000000000000000 ) ) ;
#82892=EDGE_CURVE ( 'NONE', #38685, #19715, #21803, .T. ) ;
#82893=CARTESIAN_POINT ( 'NONE',  ( 198.1257640572240177, 41.66869203097355268, 11.52974254711191726 ) ) ;
#82894=PLANE ( 'NONE',  #42771 ) ;
#82904=VECTOR ( 'NONE', #61832, 1000.000000000000000 ) ;
#82910=DIRECTION ( 'NONE',  ( -0.5729786897769871823, -0.000000000000000000, -0.8195702660915947790 ) ) ;
#82921=CARTESIAN_POINT ( 'NONE',  ( 185.8264795993290477, 214.9910457053126720, 23.09031830825835385 ) ) ;
#82924=DIRECTION ( 'NONE',  ( 0.000000000000000000, 1.000000000000000000, 0.000000000000000000 ) ) ;
#82928=ADVANCED_FACE ( 'NONE', ( #64820 ), #79259, .T. ) ;
#82938=EDGE_LOOP ( 'NONE', ( #63521, #3794 ) ) ;
#82957=FACE_OUTER_BOUND ( 'NONE', #58674, .T. ) ;
#82958=EDGE_CURVE ( 'NONE', #52628, #88979, #5630, .T. ) ;
#82962=EDGE_CURVE ( 'NONE', #15639, #18551, #7476, .T. ) ;
#82964=ORIENTED_EDGE ( 'NONE', *, *, #45009, .T. ) ;
#82971=ORIENTED_EDGE ( 'NONE', *, *, #64747, .T. ) ;
#82972=CARTESIAN_POINT ( 'NONE',  ( 157.0248177074852549, 17.42562647115544650, 9.460300111312282212 ) ) ;
#82976=ORIENTED_EDGE ( 'NONE', *, *, #47924, .F. ) ;
#82977=ORIENTED_EDGE ( 'NONE', *, *, #43977, .T. ) ;
#82990=CARTESIAN_POINT ( 'NONE',  ( 207.7670128149124196, 29.57000807141141507, 14.83937854961792979 ) ) ;
#83000=DIRECTION ( 'NONE',  ( 0.000000000000000000, 0.000000000000000000, 1.000000000000000000 ) ) ;
#83001=LINE ( 'NONE', #2558, #65536 ) ;
#83004=CARTESIAN_POINT ( 'NONE',  ( 184.8939426562960193, 2.965303559109565334, 10.00000000000000000 ) ) ;
#83007=CARTESIAN_POINT ( 'NONE',  ( 208.9490645430419704, 38.23479348326421956, 12.02378101520620746 ) ) ;
#83027=VERTEX_POINT ( 'NONE', #70960 ) ;
#83029=DIRECTION ( 'NONE',  ( 0.000000000000000000, 1.000000000000000000, 0.000000000000000000 ) ) ;
#83034=ADVANCED_FACE ( 'NONE', ( #36361 ), #35445, .F. ) ;
#83044=CIRCLE ( 'NONE', #86095, 3.000000000000007994 ) ;
#83046=DIRECTION ( 'NONE',  ( -1.000000000000000000, 0.000000000000000000, 0.000000000000000000 ) ) ;
#83059=ORIENTED_EDGE ( 'NONE', *, *, #79909, .T. ) ;
#83062=ORIENTED_EDGE ( 'NONE', *, *, #76588, .T. ) ;
#83076=ADVANCED_FACE ( 'NONE', ( #43462 ), #85149, .T. ) ;
#83083=ORIENTED_EDGE ( 'NONE', *, *, #12828, .F. ) ;
#83085=B_SPLINE_CURVE_WITH_KNOTS ( 'NONE', 3,
 ( #23962, #29694, #81254, #37244, #87417, #16399 ),
 .UNSPECIFIED., .F., .F.,
 ( 4, 2, 4 ),
 ( 0.002740393443096640798, 0.004110592855002227590, 0.005480792266907814382 ),
 .UNSPECIFIED. ) ;
#83090=CARTESIAN_POINT ( 'NONE',  ( 0.000000000000000000, 3.000000000000000000, 7.000000000000000000 ) ) ;
#83101=VECTOR ( 'NONE', #39806, 1000.000000000000000 ) ;
#83108=VECTOR ( 'NONE', #4412, 1000.000000000000000 ) ;
#83111=FACE_OUTER_BOUND ( 'NONE', #55050, .T. ) ;
#83137=FACE_OUTER_BOUND ( 'NONE', #39452, .T. ) ;
#83150=ORIENTED_EDGE ( 'NONE', *, *, #80612, .F. ) ;
#83167=DIRECTION ( 'NONE',  ( -0.000000000000000000, 1.000000000000000000, 0.000000000000000000 ) ) ;
#83171=ADVANCED_FACE ( 'NONE', ( #86531 ), #21698, .T. ) ;
#83175=CIRCLE ( 'NONE', #66575, 8.550761578869359170 ) ;
#83178=CARTESIAN_POINT ( 'NONE',  ( 185.0717070212824922, 2.982529536179759688, 9.000000000000001776 ) ) ;
#83181=TOROIDAL_SURFACE ( 'NONE', #16622, 24.50000000000000355, 0.5000000000000000000 ) ;
#83184=EDGE_LOOP ( 'NONE', ( #64420, #33830, #20045, #59073 ) ) ;
#83202=CARTESIAN_POINT ( 'NONE',  ( 152.8344704311132602, 129.4968913933752503, 12.52864452723162003 ) ) ;
#83203=CARTESIAN_POINT ( 'NONE',  ( 199.2296996224750103, 66.10105075020101140, 0.000000000000000000 ) ) ;
#83211=CARTESIAN_POINT ( 'NONE',  ( 193.6552470326849402, 250.5000000000000568, 16.89672165344822119 ) ) ;
#83214=EDGE_LOOP ( 'NONE', ( #93205, #9126 ) ) ;
#83216=CARTESIAN_POINT ( 'NONE',  ( 197.1285099842257011, 19.08195175178710556, 12.05325424581539906 ) ) ;
#83243=DIRECTION ( 'NONE',  ( 0.7957555401921962979, 0.6056179655966504871, 0.000000000000000000 ) ) ;
#83246=DIRECTION ( 'NONE',  ( 0.000000000000000000, 0.000000000000000000, 1.000000000000000000 ) ) ;
#83256=CARTESIAN_POINT ( 'NONE',  ( 179.1465552314772083, 8.542400036368780647, 25.74970488511327815 ) ) ;
#83265=DIRECTION ( 'NONE',  ( 0.000000000000000000, 0.000000000000000000, 1.000000000000000000 ) ) ;
#83267=CARTESIAN_POINT ( 'NONE',  ( 153.6539576904058038, 130.0000000000000568, -12.50000000000000000 ) ) ;
#83280=CARTESIAN_POINT ( 'NONE',  ( 195.2616234104794728, 71.31492948064700954, -13.29451844366211510 ) ) ;
#83283=ADVANCED_FACE ( 'NONE', ( #79470 ), #84481, .F. ) ;
#83286=CARTESIAN_POINT ( 'NONE',  ( 199.0061125298537377, 275.0000000000000568, -7.725424859374024678 ) ) ;
#83287=CARTESIAN_POINT ( 'NONE',  ( 195.8614702967192329, 25.38294244956506773, 14.12010220544310535 ) ) ;
#83301=ADVANCED_FACE ( 'NONE', ( #856 ), #8405, .T. ) ;
#83305=ORIENTED_EDGE ( 'NONE', *, *, #49429, .F. ) ;
#83323=DIRECTION ( 'NONE',  ( 0.000000000000000000, 0.000000000000000000, -1.000000000000000000 ) ) ;
#83342=CARTESIAN_POINT ( 'NONE',  ( 201.2509219214787777, 65.09645894983574976, 2.633798379907748455 ) ) ;
#83352=DIRECTION ( 'NONE',  ( -0.000000000000000000, -1.000000000000000000, -0.000000000000000000 ) ) ;
#83354=DIRECTION ( 'NONE',  ( 1.110223024625155531E-13, 0.000000000000000000, 1.000000000000000000 ) ) ;
#83356=DIRECTION ( 'NONE',  ( -1.000000000000000000, 0.000000000000000000, 0.000000000000000000 ) ) ;
#83368=ORIENTED_EDGE ( 'NONE', *, *, #8361, .F. ) ;
#83371=VECTOR ( 'NONE', #83167, 1000.000000000000000 ) ;
#83385=DIRECTION ( 'NONE',  ( 0.000000000000000000, 0.000000000000000000, 1.000000000000000000 ) ) ;
#83399=ORIENTED_EDGE ( 'NONE', *, *, #584, .T. ) ;
#83417=PLANE ( 'NONE',  #14292 ) ;
#83422=EDGE_LOOP ( 'NONE', ( #22550, #44601, #14753, #3903 ) ) ;
#83430=ORIENTED_EDGE ( 'NONE', *, *, #41338, .F. ) ;
#83435=ORIENTED_EDGE ( 'NONE', *, *, #51069, .T. ) ;
#83441=AXIS2_PLACEMENT_3D ( 'NONE', #63816, #6966, #42459 ) ;
#83456=CARTESIAN_POINT ( 'NONE',  ( 175.2296996224750103, 250.0000000000000568, 0.000000000000000000 ) ) ;
#83461=FACE_OUTER_BOUND ( 'NONE', #51167, .T. ) ;
#83462=DIRECTION ( 'NONE',  ( 0.000000000000000000, -0.000000000000000000, -1.000000000000000000 ) ) ;
#83465=SPHERICAL_SURFACE ( 'NONE', #54394, 3.000000000000000000 ) ;
#83468=CARTESIAN_POINT ( 'NONE',  ( 202.4403316624504043, 63.53362652955857470, 6.999999999998341771 ) ) ;
#83470=CARTESIAN_POINT ( 'NONE',  ( 152.4536156746142410, 129.7208004331680797, -12.50000000000000000 ) ) ;
#83485=CARTESIAN_POINT ( 'NONE',  ( 150.4957602436334412, 20.99999999999998934, 3.637614988394418880 ) ) ;
#83490=LINE ( 'NONE', #91041, #74544 ) ;
#83505=LINE ( 'NONE', #38087, #16672 ) ;
#83508=TOROIDAL_SURFACE ( 'NONE', #42701, 4.499999999999990230, 0.5000000000000000000 ) ;
#83522=VERTEX_POINT ( 'NONE', #67581 ) ;
#83525=ORIENTED_EDGE ( 'NONE', *, *, #72959, .T. ) ;
#83547=VERTEX_POINT ( 'NONE', #8857 ) ;
#83549=VERTEX_POINT ( 'NONE', #36828 ) ;
#83557=DIRECTION ( 'NONE',  ( -1.000000000000000000, -4.095251346825557639E-15, 0.000000000000000000 ) ) ;
#83561=CARTESIAN_POINT ( 'NONE',  ( 195.5353459679622290, 20.92212392303436985, -14.58720617293945310 ) ) ;
#83570=AXIS2_PLACEMENT_3D ( 'NONE', #40935, #25355, #11150 ) ;
#83573=TOROIDAL_SURFACE ( 'NONE', #57928, 4.499999999999993783, 0.5000000000000000000 ) ;
#83576=CARTESIAN_POINT ( 'NONE',  ( 197.0936144127869341, 69.78646135765499992, 10.59529938563716200 ) ) ;
#83578=AXIS2_PLACEMENT_3D ( 'NONE', #70267, #84898, #20047 ) ;
#83582=CARTESIAN_POINT ( 'NONE',  ( 175.2296996224750103, 158.6892791692949629, 24.00000000000001066 ) ) ;
#83585=CARTESIAN_POINT ( 'NONE',  ( 196.8872833010042882, 42.02416330566287428, 12.48796469961284572 ) ) ;
#83589=CIRCLE ( 'NONE', #12587, 7.999911143031724237 ) ;
#83591=CARTESIAN_POINT ( 'NONE',  ( 160.5350683151633291, 249.5000000000000568, 25.22542485937379197 ) ) ;
#83600=DIRECTION ( 'NONE',  ( 0.000000000000000000, 0.000000000000000000, -1.000000000000000000 ) ) ;
#83602=EDGE_CURVE ( 'NONE', #31710, #51979, #60480, .T. ) ;
#83605=CARTESIAN_POINT ( 'NONE',  ( 175.2296996224750103, 140.2072866198470251, -24.00000000000002132 ) ) ;
#83608=AXIS2_PLACEMENT_3D ( 'NONE', #14368, #51245, #78750 ) ;
#83622=DIRECTION ( 'NONE',  ( 0.000000000000000000, 0.000000000000000000, 1.000000000000000000 ) ) ;
#83632=EDGE_LOOP ( 'NONE', ( #62123, #24031, #45222, #68542 ) ) ;
#83645=CARTESIAN_POINT ( 'NONE',  ( 200.6103193995254230, 250.5000000000000568, -2.464576988612312114 ) ) ;
#83660=ORIENTED_EDGE ( 'NONE', *, *, #22726, .T. ) ;
#83665=CARTESIAN_POINT ( 'NONE',  ( 185.2786201558346306, 214.5679412853093595, 22.89156442063597297 ) ) ;
#83668=CYLINDRICAL_SURFACE ( 'NONE', #42787, 3.000000000000000000 ) ;
#83679=CARTESIAN_POINT ( 'NONE',  ( 195.0120035674127337, 41.75829791874501495, 13.59005667143956764 ) ) ;
#83682=VERTEX_POINT ( 'NONE', #80369 ) ;
#83697=DIRECTION ( 'NONE',  ( -0.000000000000000000, -1.000000000000000000, -0.000000000000000000 ) ) ;
#83698=CARTESIAN_POINT ( 'NONE',  ( 196.8702642586143270, 40.96915988761478644, 12.42857142857141994 ) ) ;
#83709=AXIS2_PLACEMENT_3D ( 'NONE', #27244, #85921, #14460 ) ;
#83712=PLANE ( 'NONE',  #14282 ) ;
#83721=EDGE_CURVE ( 'NONE', #19500, #87290, #26306, .T. ) ;
#83725=CARTESIAN_POINT ( 'NONE',  ( 195.4738470807140800, 39.72044523931811000, 14.98562018837177590 ) ) ;
#83732=AXIS2_PLACEMENT_3D ( 'NONE', #3663, #84117, #32068 ) ;
#83750=ORIENTED_EDGE ( 'NONE', *, *, #50836, .F. ) ;
#83760=DIRECTION ( 'NONE',  ( -0.000000000000000000, -1.000000000000000000, -0.000000000000000000 ) ) ;
#83761=CARTESIAN_POINT ( 'NONE',  ( 196.1314029556922947, 25.10402156816986974, 13.71726109663742754 ) ) ;
#83770=ORIENTED_EDGE ( 'NONE', *, *, #11869, .F. ) ;
#83780=ORIENTED_EDGE ( 'NONE', *, *, #90876, .F. ) ;
#83782=DIRECTION ( 'NONE',  ( -0.000000000000000000, -1.000000000000000000, -0.000000000000000000 ) ) ;
#83787=CARTESIAN_POINT ( 'NONE',  ( 197.2991597539432860, 24.58358476407964588, 10.37296855621334757 ) ) ;
#83799=CARTESIAN_POINT ( 'NONE',  ( 202.9738562182569694, 293.9636489450776367, -54.00000000000000000 ) ) ;
#83801=CIRCLE ( 'NONE', #62693, 3.589950628481164419 ) ;
#83803=AXIS2_PLACEMENT_3D ( 'NONE', #56929, #72064, #84823 ) ;
#83810=AXIS2_PLACEMENT_3D ( 'NONE', #47816, #76255, #56357 ) ;
#83818=VECTOR ( 'NONE', #56900, 1000.000000000000000 ) ;
#83836=DIRECTION ( 'NONE',  ( 1.000000000000000000, 0.000000000000000000, -0.000000000000000000 ) ) ;
#83838=CARTESIAN_POINT ( 'NONE',  ( 204.6539576904058606, 293.9636489450776367, 3.999999999999991562 ) ) ;
#83839=LINE ( 'NONE', #90448, #82097 ) ;
#83847=EDGE_CURVE ( 'NONE', #4469, #38261, #77690, .T. ) ;
#83850=ORIENTED_EDGE ( 'NONE', *, *, #63587, .F. ) ;
#83854=DIRECTION ( 'NONE',  ( 0.000000000000000000, 1.000000000000000000, 0.000000000000000000 ) ) ;
#83867=CARTESIAN_POINT ( 'NONE',  ( 185.4166944662832179, 276.0000000000000568, 23.37680765314684450 ) ) ;
#83880=AXIS2_PLACEMENT_3D ( 'NONE', #86003, #21615, #50498 ) ;
#83885=ORIENTED_EDGE ( 'NONE', *, *, #28405, .T. ) ;
#83906=EDGE_LOOP ( 'NONE', ( #2501, #15933 ) ) ;
#83914=CARTESIAN_POINT ( 'NONE',  ( 139.1539576904058606, 250.5000000000000568, -10.49999999999999822 ) ) ;
#83917=EDGE_CURVE ( 'NONE', #92859, #16590, #16444, .T. ) ;
#83919=ORIENTED_EDGE ( 'NONE', *, *, #89946, .T. ) ;
#83943=DIRECTION ( 'NONE',  ( -0.9693563597868444237, -0.2456588035076248677, 0.000000000000000000 ) ) ;
#83945=VECTOR ( 'NONE', #17174, 1000.000000000000000 ) ;
#83948=CYLINDRICAL_SURFACE ( 'NONE', #33175, 0.5000000000000004441 ) ;
#83950=EDGE_LOOP ( 'NONE', ( #92257, #64636, #55823, #59564 ) ) ;
#83951=CARTESIAN_POINT ( 'NONE',  ( 156.4869342561215433, 15.84738232520326839, -9.998183562659054502 ) ) ;
#83957=CARTESIAN_POINT ( 'NONE',  ( 154.4364498827578984, 20.25578850496138017, -11.06489058133415959 ) ) ;
#83967=ORIENTED_EDGE ( 'NONE', *, *, #17906, .T. ) ;
#83972=EDGE_LOOP ( 'NONE', ( #60030, #27668, #38585, #72185 ) ) ;
#83974=CARTESIAN_POINT ( 'NONE',  ( 175.2296996224750103, 275.0000000000000568, 0.000000000000000000 ) ) ;
#83989=CARTESIAN_POINT ( 'NONE',  ( 140.6539576904058606, 249.5000000000000568, -10.49999999999999822 ) ) ;
#84026=B_SPLINE_CURVE_WITH_KNOTS ( 'NONE', 3,
 ( #38445, #88160, #74916, #75830, #67352, #16217 ),
 .UNSPECIFIED., .F., .F.,
 ( 4, 2, 4 ),
 ( 0.000000000000000000, 0.0005356813221244592508, 0.001071362644248918502 ),
 .UNSPECIFIED. ) ;
#84029=ORIENTED_EDGE ( 'NONE', *, *, #47145, .F. ) ;
#84037=FACE_OUTER_BOUND ( 'NONE', #65685, .T. ) ;
#84042=CARTESIAN_POINT ( 'NONE',  ( 195.1488485761295237, 20.98501176085694198, -15.11070357071327663 ) ) ;
#84049=CARTESIAN_POINT ( 'NONE',  ( 153.4663172977970760, 19.61030786773756063, -12.30588869046549227 ) ) ;
#84053=CARTESIAN_POINT ( 'NONE',  ( 196.1374725241009287, 72.62824853675920167, 11.78667506127216491 ) ) ;
#84060=FACE_OUTER_BOUND ( 'NONE', #22367, .T. ) ;
#84065=PLANE ( 'NONE',  #54669 ) ;
#84074=LINE ( 'NONE', #33903, #4253 ) ;
#84081=CIRCLE ( 'NONE', #43282, 0.5000000000000000000 ) ;
#84092=ADVANCED_FACE ( 'NONE', ( #25862 ), #61423, .T. ) ;
#84095=ORIENTED_EDGE ( 'NONE', *, *, #61560, .T. ) ;
#84117=DIRECTION ( 'NONE',  ( 0.9764705882352960886, 0.000000000000000000, -0.2156506209390900708 ) ) ;
#84131=ORIENTED_EDGE ( 'NONE', *, *, #8590, .T. ) ;
#84138=DIRECTION ( 'NONE',  ( 0.000000000000000000, 0.000000000000000000, 1.000000000000000000 ) ) ;
#84146=ADVANCED_FACE ( 'NONE', ( #19247 ), #88277, .T. ) ;
#84148=EDGE_CURVE ( 'NONE', #21852, #16590, #77009, .T. ) ;
#84149=CARTESIAN_POINT ( 'NONE',  ( 154.7659666677267865, 20.47222690886501439, 12.53936336329526391 ) ) ;
#84151=ORIENTED_EDGE ( 'NONE', *, *, #66023, .T. ) ;
#84152=DIRECTION ( 'NONE',  ( 0.000000000000000000, 1.000000000000000000, 0.000000000000000000 ) ) ;
#84166=CARTESIAN_POINT ( 'NONE',  ( 192.9623460957494956, 276.0000000000000568, 16.90571646082668522 ) ) ;
#84167=CARTESIAN_POINT ( 'NONE',  ( 195.7604110529815387, 40.59022550416383979, 13.56018423268811546 ) ) ;
#84179=CARTESIAN_POINT ( 'NONE',  ( 205.4738562182569694, 293.9636489450776367, -44.00000000000000000 ) ) ;
#84181=EDGE_CURVE ( 'NONE', #28384, #69769, #91308, .T. ) ;
#84191=CARTESIAN_POINT ( 'NONE',  ( 195.5412247871907994, 40.24049585611148672, 14.88037134915001403 ) ) ;
#84195=CIRCLE ( 'NONE', #16153, 4.025000000000000355 ) ;
#84203=CARTESIAN_POINT ( 'NONE',  ( 198.6884013828325521, 64.61450673763174279, 9.555809373750800972 ) ) ;
#84224=CARTESIAN_POINT ( 'NONE',  ( 200.4551663813218170, 64.49084098419280053, 0.000000000000000000 ) ) ;
#84225=CARTESIAN_POINT ( 'NONE',  ( 160.5350683151633291, 275.0000000000000568, 20.22542485937379908 ) ) ;
#84226=DIRECTION ( 'NONE',  ( 0.000000000000000000, 0.000000000000000000, 1.000000000000000000 ) ) ;
#84245=ORIENTED_EDGE ( 'NONE', *, *, #6444, .T. ) ;
#84246=CARTESIAN_POINT ( 'NONE',  ( 155.8658096505380684, 20.95954935106544426, -14.18771993490441830 ) ) ;
#84255=ADVANCED_FACE ( 'NONE', ( #39125 ), #8131, .T. ) ;
#84271=CARTESIAN_POINT ( 'NONE',  ( 208.6208076322478746, 32.98517505407394168, 13.08022668053247095 ) ) ;
#84284=CARTESIAN_POINT ( 'NONE',  ( 152.4536156746142410, 249.5000000000000568, -12.00000000000000000 ) ) ;
#84298=DIRECTION ( 'NONE',  ( 0.000000000000000000, 0.000000000000000000, 1.000000000000000000 ) ) ;
#84307=VERTEX_POINT ( 'NONE', #25404 ) ;
#84321=EDGE_CURVE ( 'NONE', #78294, #57275, #15110, .T. ) ;
#84324=PLANE ( 'NONE',  #40512 ) ;
#84340=ORIENTED_EDGE ( 'NONE', *, *, #4248, .T. ) ;
#84345=ADVANCED_FACE ( 'NONE', ( #4108 ), #90255, .F. ) ;
#84351=ORIENTED_EDGE ( 'NONE', *, *, #75975, .T. ) ;
#84363=ORIENTED_EDGE ( 'NONE', *, *, #52765, .T. ) ;
#84370=ORIENTED_EDGE ( 'NONE', *, *, #78108, .T. ) ;
#84371=DIRECTION ( 'NONE',  ( 1.000000000000000000, 0.000000000000000000, 0.000000000000000000 ) ) ;
#84376=ORIENTED_EDGE ( 'NONE', *, *, #4626, .T. ) ;
#84383=PLANE ( 'NONE',  #38155 ) ;
#84393=ADVANCED_FACE ( 'NONE', ( #69435 ), #26387, .T. ) ;
#84399=LINE ( 'NONE', #10106, #2009 ) ;
#84405=CARTESIAN_POINT ( 'NONE',  ( 201.2104617360081704, 60.19600395700749829, -7.000000000000000888 ) ) ;
#84407=EDGE_LOOP ( 'NONE', ( #67837, #46957, #676, #4961 ) ) ;
#84408=DIRECTION ( 'NONE',  ( 0.000000000000000000, 0.000000000000000000, 1.000000000000000000 ) ) ;
#84426=CARTESIAN_POINT ( 'NONE',  ( 206.4403749041381388, 36.15246451355368862, 13.98713712351916172 ) ) ;
#84430=CARTESIAN_POINT ( 'NONE',  ( 197.4657836131030706, 215.0000000000000568, -12.48225014817974987 ) ) ;
#84444=CARTESIAN_POINT ( 'NONE',  ( 185.8264795993290193, 275.5000000000000568, 23.09031830825835385 ) ) ;
#84451=DIRECTION ( 'NONE',  ( 0.6573509547581669610, 0.1665889405894028785, -0.7349407099568147084 ) ) ;
#84462=VERTEX_POINT ( 'NONE', #39581 ) ;
#84467=EDGE_CURVE ( 'NONE', #19834, #13609, #85322, .T. ) ;
#84479=VERTEX_POINT ( 'NONE', #48105 ) ;
#84481=( BOUNDED_SURFACE ( )  B_SPLINE_SURFACE ( 3, 2, ( 
 ( #27396, #14604, #379 ),
 ( #58163, #70503, #78067 ),
 ( #22159, #20302, #13210 ),
 ( #34965, #92715, #63877 ),
 ( #20763, #49635, #31591 ),
 ( #38676, #87920, #52880 ) ),
 .UNSPECIFIED., .F., .F., .F. ) 
 B_SPLINE_SURFACE_WITH_KNOTS ( ( 4, 2, 4 ),
 ( 3, 3 ),
 ( 0.005169333131382347624, 0.006119585499877700299, 0.007069837868373052975 ),
 ( 0.000000000000000000, 0.5783792227927410101 ),
 .UNSPECIFIED. ) 
 GEOMETRIC_REPRESENTATION_ITEM ( )  RATIONAL_B_SPLINE_SURFACE ( (
 ( 1.000000000000000000, 0.8305966477414097326, 0.8571520539184362963),
 ( 1.000000000000000000, 0.8412850701494818395, 0.8661649758440579383),
 ( 1.000000000000000000, 0.8530303058598047716, 0.8760690466613954008),
 ( 1.000000000000000000, 0.8717109521664421212, 0.8918213438904722956),
 ( 1.000000000000000000, 0.8783573442016358035, 0.8974258578414773257),
 ( 1.000000000000000000, 0.8782019693812768146, 0.8972948393364408304) ) ) 
 REPRESENTATION_ITEM ( '' )  SURFACE ( )  );
#84487=( BOUNDED_SURFACE ( )  B_SPLINE_SURFACE ( 3, 2, ( 
 ( #13405, #64081, #63612 ),
 ( #25708, #27600, #54590 ),
 ( #22346, #51218, #42718 ),
 ( #80108, #56970, #71635 ),
 ( #20958, #49826, #37470 ),
 ( #13864, #43202, #86268 ) ),
 .UNSPECIFIED., .F., .F., .F. ) 
 B_SPLINE_SURFACE_WITH_KNOTS ( ( 4, 2, 4 ),
 ( 3, 3 ),
 ( 0.006633574617387602568, 0.007266361004544705585, 0.007899147391701808602 ),
 ( 0.000000000000000000, 1.000000000000000000 ),
 .UNSPECIFIED. ) 
 GEOMETRIC_REPRESENTATION_ITEM ( )  RATIONAL_B_SPLINE_SURFACE ( (
 ( 1.000000000000000000, 0.8333723006562869795, 1.000000000000000000),
 ( 1.000000000000000000, 0.8265668121450767680, 1.000000000000000000),
 ( 1.000000000000000000, 0.8184438728316124623, 1.000000000000000000),
 ( 1.000000000000000000, 0.7999168228917755696, 1.000000000000000000),
 ( 1.000000000000000000, 0.7897639513982999127, 1.000000000000000000),
 ( 1.000000000000000000, 0.7791885400064296752, 1.000000000000000000) ) ) 
 REPRESENTATION_ITEM ( '' )  SURFACE ( )  );
#84490=ADVANCED_FACE ( 'NONE', ( #11202 ), #67219, .T. ) ;
#84498=CARTESIAN_POINT ( 'NONE',  ( 153.1687287787711114, 19.71439303875248683, -10.22517819557502605 ) ) ;
#84510=CARTESIAN_POINT ( 'NONE',  ( 153.3662540421047424, 20.33090216074013412, 12.12586741969728443 ) ) ;
#84519=CARTESIAN_POINT ( 'NONE',  ( 201.2104617360081704, 60.19600395700749829, -9.000000000000000000 ) ) ;
#84523=DIRECTION ( 'NONE',  ( 0.5831039236546639026, -0.7661730729848326149, -0.2701270746362063879 ) ) ;
#84552=EDGE_CURVE ( 'NONE', #47807, #37341, #27519, .T. ) ;
#84557=CARTESIAN_POINT ( 'NONE',  ( 154.3564990690576906, 19.12150670424914267, 10.40578999957047479 ) ) ;
#84567=ORIENTED_EDGE ( 'NONE', *, *, #75724, .T. ) ;
#84568=ORIENTED_EDGE ( 'NONE', *, *, #7722, .T. ) ;
#84578=DIRECTION ( 'NONE',  ( -0.2156506209390900430, 0.000000000000000000, 0.9764705882352960886 ) ) ;
#84583=ORIENTED_EDGE ( 'NONE', *, *, #57879, .F. ) ;
#84592=ORIENTED_EDGE ( 'NONE', *, *, #65327, .T. ) ;
#84596=ORIENTED_EDGE ( 'NONE', *, *, #40020, .T. ) ;
#84598=CARTESIAN_POINT ( 'NONE',  ( 205.4738562182569694, 293.9636489450776367, -44.00000000000000000 ) ) ;
#84600=VECTOR ( 'NONE', #15725, 1000.000000000000000 ) ;
#84601=DIRECTION ( 'NONE',  ( -0.000000000000000000, -0.000000000000000000, -1.000000000000000000 ) ) ;
#84604=CIRCLE ( 'NONE', #55904, 1.499999999999999556 ) ;
#84610=DIRECTION ( 'NONE',  ( 0.000000000000000000, 0.000000000000000000, 1.000000000000000000 ) ) ;
#84612=EDGE_CURVE ( 'NONE', #52994, #23580, #48574, .T. ) ;
#84613=ORIENTED_EDGE ( 'NONE', *, *, #48, .F. ) ;
#84614=EDGE_LOOP ( 'NONE', ( #42434, #27149, #70520, #47887 ) ) ;
#84644=CARTESIAN_POINT ( 'NONE',  ( 175.2296996224750103, 128.0000000000000568, 0.000000000000000000 ) ) ;
#84654=CARTESIAN_POINT ( 'NONE',  ( 196.7035422149454291, 42.02664470600696944, 12.80665658919290628 ) ) ;
#84660=AXIS2_PLACEMENT_3D ( 'NONE', #12854, #79110, #49281 ) ;
#84663=EDGE_LOOP ( 'NONE', ( #75637, #55630, #3030, #89022 ) ) ;
#84666=CARTESIAN_POINT ( 'NONE',  ( 201.2104617360081704, 60.19600395700749829, 9.000000000000001776 ) ) ;
#84671=EDGE_CURVE ( 'NONE', #17165, #46065, #45964, .T. ) ;
#84672=ADVANCED_FACE ( 'NONE', ( #14838 ), #645, .T. ) ;
#84679=VERTEX_POINT ( 'NONE', #58394 ) ;
#84680=CARTESIAN_POINT ( 'NONE',  ( 194.2870706633419218, 39.56969527624839600, 14.58823529460389246 ) ) ;
#84689=EDGE_CURVE ( 'NONE', #84890, #70200, #77475, .T. ) ;
#84692=DIRECTION ( 'NONE',  ( -0.000000000000000000, -1.000000000000000000, -0.000000000000000000 ) ) ;
#84705=ORIENTED_EDGE ( 'NONE', *, *, #40483, .F. ) ;
#84714=DIRECTION ( 'NONE',  ( 0.7806247497998081153, 0.000000000000000000, 0.6249999999999895639 ) ) ;
#84729=DIRECTION ( 'NONE',  ( -1.000000000000000000, 0.000000000000000000, 0.000000000000000000 ) ) ;
#84738=CARTESIAN_POINT ( 'NONE',  ( 150.6539576904058606, 293.9636489450775230, -9.103929867429224387 ) ) ;
#84741=AXIS2_PLACEMENT_3D ( 'NONE', #41810, #20532, #4902 ) ;
#84751=CARTESIAN_POINT ( 'NONE',  ( 198.7962788613918690, 70.38469146216345962, 8.627472241157438049 ) ) ;
#84775=ORIENTED_EDGE ( 'NONE', *, *, #12020, .F. ) ;
#84778=CARTESIAN_POINT ( 'NONE',  ( 180.7287904564219332, 249.5000000000000568, -24.90000000000002345 ) ) ;
#84782=EDGE_CURVE ( 'NONE', #14615, #37664, #74714, .T. ) ;
#84791=CARTESIAN_POINT ( 'NONE',  ( 154.1407330040854333, 275.5000000000000568, 13.42592592592592915 ) ) ;
#84792=CYLINDRICAL_SURFACE ( 'NONE', #85898, 1.000000000000000888 ) ;
#84808=ORIENTED_EDGE ( 'NONE', *, *, #22107, .F. ) ;
#84823=DIRECTION ( 'NONE',  ( 0.000000000000000000, 0.000000000000000000, 1.000000000000000000 ) ) ;
#84836=ORIENTED_EDGE ( 'NONE', *, *, #50049, .F. ) ;
#84860=ADVANCED_FACE ( 'NONE', ( #73051 ), #91096, .T. ) ;
#84865=DIRECTION ( 'NONE',  ( -0.4472135954999548191, 0.4472135954999599261, 0.7745966692414840704 ) ) ;
#84866=CARTESIAN_POINT ( 'NONE',  ( 196.0143093133015384, 19.33012701892219098, 12.49999999999999467 ) ) ;
#84879=DIRECTION ( 'NONE',  ( 0.000000000000000000, 1.000000000000000000, 0.000000000000000000 ) ) ;
#84888=EDGE_CURVE ( 'NONE', #70448, #12291, #42261, .T. ) ;
#84890=VERTEX_POINT ( 'NONE', #52643 ) ;
#84893=LINE ( 'NONE', #48923, #38259 ) ;
#84898=DIRECTION ( 'NONE',  ( 0.000000000000000000, 1.000000000000000000, 0.000000000000000000 ) ) ;
#84928=ORIENTED_EDGE ( 'NONE', *, *, #25761, .T. ) ;
#84939=CIRCLE ( 'NONE', #39554, 0.5000000000000048850 ) ;
#84950=VERTEX_POINT ( 'NONE', #24234 ) ;
#84952=VECTOR ( 'NONE', #13184, 1000.000000000000000 ) ;
#84959=VERTEX_POINT ( 'NONE', #67806 ) ;
#84969=EDGE_CURVE ( 'NONE', #75719, #10071, #84026, .T. ) ;
#84979=CYLINDRICAL_SURFACE ( 'NONE', #68452, 4.999999999999990230 ) ;
#84984=CARTESIAN_POINT ( 'NONE',  ( 216.5288609127277084, 293.9636489450776935, -40.00000000000000711 ) ) ;
#84987=DIRECTION ( 'NONE',  ( -0.000000000000000000, -1.000000000000000000, -0.000000000000000000 ) ) ;
#84990=CARTESIAN_POINT ( 'NONE',  ( 209.7513585654923816, 282.2246705312486483, 13.99999999999999112 ) ) ;
#84991=CARTESIAN_POINT ( 'NONE',  ( 175.2296996224750103, 140.2072866198470251, 0.000000000000000000 ) ) ;
#84997=ADVANCED_FACE ( 'NONE', ( #81072, #89085, #39351 ), #10954, .T. ) ;
#85002=VECTOR ( 'NONE', #16952, 1000.000000000000000 ) ;
#85007=CARTESIAN_POINT ( 'NONE',  ( 208.2940771383659069, 37.39347744730360290, 12.94649967098113841 ) ) ;
#85009=AXIS2_PLACEMENT_3D ( 'NONE', #92934, #7232, #28548 ) ;
#85011=LINE ( 'NONE', #28217, #54328 ) ;
#85025=EDGE_CURVE ( 'NONE', #69004, #85642, #2930, .T. ) ;
#85030=CARTESIAN_POINT ( 'NONE',  ( 190.2832783574276903, 8.542400036368780647, 25.74970488511327815 ) ) ;
#85032=EDGE_CURVE ( 'NONE', #13010, #17769, #58101, .T. ) ;
#85040=( BOUNDED_CURVE ( )  B_SPLINE_CURVE ( 3, ( #34562, #68680, #40226, #70564 ),
 .UNSPECIFIED., .F., .F. ) 
 B_SPLINE_CURVE_WITH_KNOTS ( ( 4, 4 ),
 ( 0.000000000000000000, 0.2609887789853130857 ),
 .UNSPECIFIED. ) 
 CURVE ( )  GEOMETRIC_REPRESENTATION_ITEM ( )  RATIONAL_B_SPLINE_CURVE ( ( 1.000000000000000000, 0.9943317885200935180, 0.9943317885200935180, 1.000000000000000000 ) ) 
 REPRESENTATION_ITEM ( '' )  );
#85042=ORIENTED_EDGE ( 'NONE', *, *, #46621, .F. ) ;
#85043=ORIENTED_EDGE ( 'NONE', *, *, #33978, .F. ) ;
#85055=DIRECTION ( 'NONE',  ( 1.000000000000000000, 0.000000000000000000, 0.000000000000000000 ) ) ;
#85068=ORIENTED_EDGE ( 'NONE', *, *, #17385, .F. ) ;
#85072=VERTEX_POINT ( 'NONE', #3392 ) ;
#85076=CIRCLE ( 'NONE', #3422, 6.286090667950827715 ) ;
#85077=CARTESIAN_POINT ( 'NONE',  ( 197.1123855246549113, 19.09807621135331601, 10.09807621135331246 ) ) ;
#85078=CIRCLE ( 'NONE', #50341, 4.103083949679980691 ) ;
#85085=FACE_OUTER_BOUND ( 'NONE', #56227, .T. ) ;
#85086=DIRECTION ( 'NONE',  ( 1.000000000000000000, 0.000000000000000000, 0.000000000000000000 ) ) ;
#85090=ORIENTED_EDGE ( 'NONE', *, *, #42395, .T. ) ;
#85091=DIRECTION ( 'NONE',  ( 0.000000000000000000, 1.000000000000000000, 0.000000000000000000 ) ) ;
#85107=FACE_OUTER_BOUND ( 'NONE', #41754, .T. ) ;
#85122=EDGE_CURVE ( 'NONE', #13924, #77289, #76262, .T. ) ;
#85134=DIRECTION ( 'NONE',  ( 1.000000000000000000, 0.000000000000000000, 0.000000000000000000 ) ) ;
#85139=CIRCLE ( 'NONE', #82086, 4.999999999999985789 ) ;
#85143=CIRCLE ( 'NONE', #74603, 4.999999999999986677 ) ;
#85145=ORIENTED_EDGE ( 'NONE', *, *, #31275, .F. ) ;
#85146=CARTESIAN_POINT ( 'NONE',  ( 151.4851178187871312, 20.00000000000000000, 3.492110388858642889 ) ) ;
#85149=CYLINDRICAL_SURFACE ( 'NONE', #33825, 25.00000000000001066 ) ;
#85155=CIRCLE ( 'NONE', #20140, 0.4999999999999998335 ) ;
#85160=ORIENTED_EDGE ( 'NONE', *, *, #42029, .F. ) ;
#85161=FACE_OUTER_BOUND ( 'NONE', #31848, .T. ) ;
#85165=AXIS2_PLACEMENT_3D ( 'NONE', #12452, #4877, #69279 ) ;
#85166=ADVANCED_FACE ( 'NONE', ( #61641 ), #41219, .T. ) ;
#85168=ORIENTED_EDGE ( 'NONE', *, *, #53277, .T. ) ;
#85174=CARTESIAN_POINT ( 'NONE',  ( 198.6801208295229344, 66.92094681839049031, -8.363400713796702135 ) ) ;
#85175=AXIS2_PLACEMENT_3D ( 'NONE', #80344, #67088, #59046 ) ;
#85176=DIRECTION ( 'NONE',  ( 0.000000000000000000, -1.000000000000000000, 0.000000000000000000 ) ) ;
#85186=VECTOR ( 'NONE', #47271, 1000.000000000000114 ) ;
#85187=ORIENTED_EDGE ( 'NONE', *, *, #63994, .T. ) ;
#85209=ORIENTED_EDGE ( 'NONE', *, *, #29336, .F. ) ;
#85210=ORIENTED_EDGE ( 'NONE', *, *, #31277, .F. ) ;
#85211=CARTESIAN_POINT ( 'NONE',  ( 196.0143093133017658, 19.33012701892200624, -12.49999999999967315 ) ) ;
#85221=AXIS2_PLACEMENT_3D ( 'NONE', #64304, #20240, #70450 ) ;
#85227=CARTESIAN_POINT ( 'NONE',  ( 199.5308170082192021, 67.35660163415921886, -10.35296668938369180 ) ) ;
#85228=DIRECTION ( 'NONE',  ( 0.000000000000000000, 0.000000000000000000, 1.000000000000000000 ) ) ;
#85229=TOROIDAL_SURFACE ( 'NONE', #61047, 24.00000000000002132, 2.046895004029262388 ) ;
#85236=AXIS2_PLACEMENT_3D ( 'NONE', #89506, #24672, #54015 ) ;
#85244=AXIS2_PLACEMENT_3D ( 'NONE', #18858, #33997, #11279 ) ;
#85251=DIRECTION ( 'NONE',  ( -0.000000000000000000, -1.000000000000000000, -0.000000000000000000 ) ) ;
#85253=FACE_OUTER_BOUND ( 'NONE', #16934, .T. ) ;
#85263=EDGE_LOOP ( 'NONE', ( #49818, #37084, #14601, #29560 ) ) ;
#85264=CARTESIAN_POINT ( 'NONE',  ( 180.7287904564219332, 250.5000000000000568, -24.90000000000003411 ) ) ;
#85277=DIRECTION ( 'NONE',  ( -0.000000000000000000, -1.000000000000000000, -0.000000000000000000 ) ) ;
#85278=EDGE_CURVE ( 'NONE', #25728, #25873, #71761, .T. ) ;
#85279=FACE_OUTER_BOUND ( 'NONE', #42103, .T. ) ;
#85282=VECTOR ( 'NONE', #92540, 1000.000000000000000 ) ;
#85287=AXIS2_PLACEMENT_3D ( 'NONE', #45381, #60565, #29820 ) ;
#85293=VERTEX_POINT ( 'NONE', #55936 ) ;
#85305=VERTEX_POINT ( 'NONE', #84791 ) ;
#85308=AXIS2_PLACEMENT_3D ( 'NONE', #21401, #14783, #58796 ) ;
#85322=CIRCLE ( 'NONE', #88341, 2.046895004029262832 ) ;
#85326=ORIENTED_EDGE ( 'NONE', *, *, #34702, .T. ) ;
#85336=DIRECTION ( 'NONE',  ( -1.000000000000000000, -0.000000000000000000, 0.000000000000000000 ) ) ;
#85344=ADVANCED_FACE ( 'NONE', ( #40287 ), #68697, .T. ) ;
#85346=ADVANCED_FACE ( 'NONE', ( #69204 ), #5751, .F. ) ;
#85355=LINE ( 'NONE', #1386, #12566 ) ;
#85362=DIRECTION ( 'NONE',  ( 0.000000000000000000, 1.000000000000000000, 9.656854691831248164E-17 ) ) ;
#85366=CARTESIAN_POINT ( 'NONE',  ( 196.8702642586143270, 40.96915988761478644, 12.42857142857141994 ) ) ;
#85369=DIRECTION ( 'NONE',  ( 0.000000000000000000, 1.000000000000000000, 0.000000000000000000 ) ) ;
#85383=LINE ( 'NONE', #11060, #66643 ) ;
#85385=ORIENTED_EDGE ( 'NONE', *, *, #20244, .F. ) ;
#85401=CARTESIAN_POINT ( 'NONE',  ( 152.4536156746142410, 275.5000000000000568, 12.49999999999999289 ) ) ;
#85416=ORIENTED_EDGE ( 'NONE', *, *, #50473, .T. ) ;
#85443=CIRCLE ( 'NONE', #23396, 0.5000000000000004441 ) ;
#85453=LINE ( 'NONE', #4976, #53238 ) ;
#85459=CARTESIAN_POINT ( 'NONE',  ( 160.5350683151633291, 275.5000000000000568, 20.22542485937379908 ) ) ;
#85466=CARTESIAN_POINT ( 'NONE',  ( 183.0442525570908288, 293.9636489450775230, 0.000000000000000000 ) ) ;
#85477=CARTESIAN_POINT ( 'NONE',  ( 197.3290507633359709, 70.40097505901294994, -11.81033421933028649 ) ) ;
#85490=FACE_OUTER_BOUND ( 'NONE', #92730, .T. ) ;
#85529=CARTESIAN_POINT ( 'NONE',  ( 197.1396238179664806, 70.11630495483946390, 10.20652033329685793 ) ) ;
#85547=CARTESIAN_POINT ( 'NONE',  ( 208.6208076322478746, 32.98517505407394168, 10.00000000000000000 ) ) ;
#85550=DIRECTION ( 'NONE',  ( -1.000000000000000000, 0.000000000000000000, 0.000000000000000000 ) ) ;
#85556=DIRECTION ( 'NONE',  ( -0.000000000000000000, -1.000000000000000000, -0.000000000000000000 ) ) ;
#85558=VERTEX_POINT ( 'NONE', #26101 ) ;
#85559=ORIENTED_EDGE ( 'NONE', *, *, #21626, .T. ) ;
#85560=CARTESIAN_POINT ( 'NONE',  ( 209.5647629949351654, 27.95999215251566028, 12.09245862095555424 ) ) ;
#85575=CARTESIAN_POINT ( 'NONE',  ( 207.6662022560301182, 36.29800326561209545, 14.90057469441957316 ) ) ;
#85577=CIRCLE ( 'NONE', #50853, 0.5000000000000004441 ) ;
#85589=DIRECTION ( 'NONE',  ( 0.000000000000000000, 0.000000000000000000, -1.000000000000000000 ) ) ;
#85591=CARTESIAN_POINT ( 'NONE',  ( 165.7865175155837676, 3.000000000000000000, -9.000000000000001776 ) ) ;
#85604=CARTESIAN_POINT ( 'NONE',  ( 196.8803347170859865, 42.36571313990104670, 12.49999999999999112 ) ) ;
#85609=( BOUNDED_SURFACE ( )  B_SPLINE_SURFACE ( 3, 2, ( 
 ( #33636, #27010, #18978 ),
 ( #83342, #47353, #55897 ),
 ( #26057, #54013, #4290 ),
 ( #47830, #11859, #84751 ),
 ( #11395, #19899, #40247 ),
 ( #62059, #77677, #40708 ) ),
 .UNSPECIFIED., .F., .F., .F. ) 
 B_SPLINE_SURFACE_WITH_KNOTS ( ( 4, 2, 4 ),
 ( 3, 3 ),
 ( 0.000000000000000000, 0.2633701841259441512, 0.5267403682518883024 ),
 ( 0.000000000000000000, 1.000000000000000000 ),
 .UNSPECIFIED. ) 
 GEOMETRIC_REPRESENTATION_ITEM ( )  RATIONAL_B_SPLINE_SURFACE ( (
 ( 1.000000000000000000, 0.9475641245298920268, 1.000000000000000000),
 ( 1.000000000000000000, 0.9475641245298920268, 1.000000000000000000),
 ( 1.000000000000000000, 0.9451322790880677394, 1.000000000000000000),
 ( 1.000000000000000000, 0.9354614375526321135, 1.000000000000000000),
 ( 1.000000000000000000, 0.9282241625909624094, 1.000000000000000000),
 ( 1.000000000000000000, 0.9186651033962678348, 1.000000000000000000) ) ) 
 REPRESENTATION_ITEM ( '' )  SURFACE ( )  );
#85615=DIRECTION ( 'NONE',  ( 0.000000000000000000, 1.000000000000000000, 0.000000000000000000 ) ) ;
#85617=CARTESIAN_POINT ( 'NONE',  ( 175.2296996224750103, 275.0000000000000568, 0.000000000000000000 ) ) ;
#85627=CARTESIAN_POINT ( 'NONE',  ( 195.1989865542159066, 41.04625909772627779, 13.32094405520072122 ) ) ;
#85638=DIRECTION ( 'NONE',  ( -0.6056179655966479336, 0.7957555401921982963, 0.000000000000000000 ) ) ;
#85639=DIRECTION ( 'NONE',  ( 0.000000000000000000, 1.000000000000000000, 0.000000000000000000 ) ) ;
#85642=VERTEX_POINT ( 'NONE', #47872 ) ;
#85648=ORIENTED_EDGE ( 'NONE', *, *, #90537, .F. ) ;
#85673=ORIENTED_EDGE ( 'NONE', *, *, #11195, .T. ) ;
#85674=ORIENTED_EDGE ( 'NONE', *, *, #63406, .T. ) ;
#85675=CARTESIAN_POINT ( 'NONE',  ( 209.3191041914274706, 28.92934851230250715, 12.09245862095555424 ) ) ;
#85691=FACE_OUTER_BOUND ( 'NONE', #18104, .T. ) ;
#85699=ADVANCED_FACE ( 'NONE', ( #63065 ), #89829, .T. ) ;
#85703=CARTESIAN_POINT ( 'NONE',  ( 151.9245405993102338, 130.8357700577111018, 11.49999999999999645 ) ) ;
#85714=DIRECTION ( 'NONE',  ( -0.000000000000000000, -1.000000000000000000, -0.000000000000000000 ) ) ;
#85724=VERTEX_POINT ( 'NONE', #68745 ) ;
#85725=LINE ( 'NONE', #79575, #25657 ) ;
#85740=EDGE_CURVE ( 'NONE', #6120, #26691, #34626, .T. ) ;
#85741=CARTESIAN_POINT ( 'NONE',  ( 170.4537599243631405, 275.0000000000000568, -23.51999999999999602 ) ) ;
#85753=ORIENTED_EDGE ( 'NONE', *, *, #42570, .T. ) ;
#85767=FACE_OUTER_BOUND ( 'NONE', #5646, .T. ) ;
#85772=ORIENTED_EDGE ( 'NONE', *, *, #17827, .F. ) ;
#85780=DIRECTION ( 'NONE',  ( 0.000000000000000000, 1.000000000000000000, 0.000000000000000000 ) ) ;
#85790=DIRECTION ( 'NONE',  ( 0.000000000000000000, 0.000000000000000000, 1.000000000000000000 ) ) ;
#85804=EDGE_CURVE ( 'NONE', #85293, #19459, #87587, .T. ) ;
#85807=DIRECTION ( 'NONE',  ( 0.000000000000000000, -0.8660254037844385966, 0.5000000000000000000 ) ) ;
#85808=CARTESIAN_POINT ( 'NONE',  ( 200.7568414405312467, 39.78480925505071752, 10.50000000000000000 ) ) ;
#85814=CARTESIAN_POINT ( 'NONE',  ( 208.6208076322478746, 32.98517505407394168, 14.69807322781335657 ) ) ;
#85816=DIRECTION ( 'NONE',  ( -1.000000000000000000, 0.000000000000000000, 0.000000000000000000 ) ) ;
#85819=CARTESIAN_POINT ( 'NONE',  ( 156.4851178187871312, 1.000000000000000000, 7.000000000000000000 ) ) ;
#85830=ORIENTED_EDGE ( 'NONE', *, *, #58734, .F. ) ;
#85870=ORIENTED_EDGE ( 'NONE', *, *, #74086, .T. ) ;
#85888=VERTEX_POINT ( 'NONE', #43586 ) ;
#85896=ORIENTED_EDGE ( 'NONE', *, *, #51587, .T. ) ;
#85898=AXIS2_PLACEMENT_3D ( 'NONE', #19942, #49298, #48814 ) ;
#85905=CARTESIAN_POINT ( 'NONE',  ( 175.2296996224750103, 21.00000000000000000, 0.000000000000000000 ) ) ;
#85917=DIRECTION ( 'NONE',  ( 0.000000000000000000, 0.000000000000000000, -1.000000000000000000 ) ) ;
#85921=DIRECTION ( 'NONE',  ( 1.000000000000000000, 0.000000000000000000, -0.000000000000000000 ) ) ;
#85924=EDGE_CURVE ( 'NONE', #10184, #20922, #86665, .T. ) ;
#85925=FACE_OUTER_BOUND ( 'NONE', #53620, .T. ) ;
#85929=DIRECTION ( 'NONE',  ( -0.000000000000000000, -0.000000000000000000, 1.000000000000000000 ) ) ;
#85942=CARTESIAN_POINT ( 'NONE',  ( 209.6916979138304953, 36.36051277703914053, 13.48241519114203690 ) ) ;
#85946=EDGE_CURVE ( 'NONE', #3443, #35022, #55112, .T. ) ;
#85958=VECTOR ( 'NONE', #16116, 1000.000000000000000 ) ;
#85973=ORIENTED_EDGE ( 'NONE', *, *, #48633, .F. ) ;
#85983=CARTESIAN_POINT ( 'NONE',  ( 140.6539576904058606, 276.0000000000000568, -12.00000000000000178 ) ) ;
#86001=VERTEX_POINT ( 'NONE', #7599 ) ;
#86003=CARTESIAN_POINT ( 'NONE',  ( 219.8344101925596021, 35.72494958537217968, 7.000000000000000000 ) ) ;
#86011=PLANE ( 'NONE',  #20137 ) ;
#86013=DIRECTION ( 'NONE',  ( 0.000000000000000000, 0.000000000000000000, 1.000000000000000000 ) ) ;
#86014=EDGE_LOOP ( 'NONE', ( #87945, #7760, #45004, #22715, #2523 ) ) ;
#86015=CARTESIAN_POINT ( 'NONE',  ( 185.4166944662832179, 215.0000000000000568, 22.87680765314684095 ) ) ;
#86022=AXIS2_PLACEMENT_3D ( 'NONE', #52276, #23862, #16299 ) ;
#86030=CARTESIAN_POINT ( 'NONE',  ( 197.1711655576864644, 291.5339772727334662, -7.625735220792024371 ) ) ;
#86031=DIRECTION ( 'NONE',  ( 0.000000000000000000, 0.000000000000000000, -1.000000000000000000 ) ) ;
#86053=FACE_OUTER_BOUND ( 'NONE', #58330, .T. ) ;
#86068=ADVANCED_FACE ( 'NONE', ( #92844 ), #10097, .F. ) ;
#86072=CARTESIAN_POINT ( 'NONE',  ( 153.2628468892467311, 20.37991841447510311, 11.93555113920849386 ) ) ;
#86074=DIRECTION ( 'NONE',  ( 0.000000000000000000, 0.000000000000000000, -1.000000000000000000 ) ) ;
#86083=ORIENTED_EDGE ( 'NONE', *, *, #65006, .T. ) ;
#86084=CARTESIAN_POINT ( 'NONE',  ( 195.4394726684814145, 39.61210057291198439, 13.99041345891462207 ) ) ;
#86095=AXIS2_PLACEMENT_3D ( 'NONE', #5505, #91648, #62324 ) ;
#86099=CARTESIAN_POINT ( 'NONE',  ( 196.2205576190423528, 72.73813141077837940, -11.64668355651677345 ) ) ;
#86133=VERTEX_POINT ( 'NONE', #7153 ) ;
#86134=ORIENTED_EDGE ( 'NONE', *, *, #13000, .T. ) ;
#86135=CARTESIAN_POINT ( 'NONE',  ( 175.2296996224750103, 154.6894116713782807, 0.000000000000000000 ) ) ;
#86149=CARTESIAN_POINT ( 'NONE',  ( 200.9021118020844199, 65.55478020308605380, -5.267193185415704804 ) ) ;
#86173=DIRECTION ( 'NONE',  ( 0.000000000000000000, 0.000000000000000000, 1.000000000000000000 ) ) ;
#86183=ADVANCED_FACE ( 'NONE', ( #65403 ), #29398, .T. ) ;
#86187=PLANE ( 'NONE',  #88211 ) ;
#86202=FACE_OUTER_BOUND ( 'NONE', #57292, .T. ) ;
#86223=ORIENTED_EDGE ( 'NONE', *, *, #16074, .F. ) ;
#86239=VERTEX_POINT ( 'NONE', #2378 ) ;
#86240=DIRECTION ( 'NONE',  ( 0.000000000000000000, 0.000000000000000000, 1.000000000000000000 ) ) ;
#86254=CARTESIAN_POINT ( 'NONE',  ( 185.8821869067168393, 215.0000000000000568, 23.16839473634431101 ) ) ;
#86260=ORIENTED_EDGE ( 'NONE', *, *, #47247, .F. ) ;
#86265=EDGE_CURVE ( 'NONE', #69489, #84890, #55180, .T. ) ;
#86268=CARTESIAN_POINT ( 'NONE',  ( 153.9133111279456045, 20.47222690886501439, 13.06183683676589524 ) ) ;
#86279=CARTESIAN_POINT ( 'NONE',  ( 151.4851178187871312, 21.00000000000000000, -3.492110388858667314 ) ) ;
#86296=ORIENTED_EDGE ( 'NONE', *, *, #53514, .T. ) ;
#86299=CIRCLE ( 'NONE', #3168, 1.500000000000001332 ) ;
#86306=VERTEX_POINT ( 'NONE', #53008 ) ;
#86312=CARTESIAN_POINT ( 'NONE',  ( 201.2104617360081704, 0.000000000000000000, 9.000000000000001776 ) ) ;
#86327=ORIENTED_EDGE ( 'NONE', *, *, #46324, .F. ) ;
#86330=ORIENTED_EDGE ( 'NONE', *, *, #10314, .F. ) ;
#86333=EDGE_CURVE ( 'NONE', #50317, #5104, #709, .T. ) ;
#86341=B_SPLINE_CURVE_WITH_KNOTS ( 'NONE', 3,
 ( #15728, #14354, #13877, #43214, #79669, #57438, #599, #44589, #73493, #37033, #21432, #73022, #65947, #57892, #1058, #37481 ),
 .UNSPECIFIED., .F., .F.,
 ( 4, 2, 2, 2, 2, 2, 2, 4 ),
 ( 0.000000000000000000, 0.001221894770150660538, 0.001832842155225994276, 0.002443789540301328448, 0.003054736925376662620, 0.003665684310451996358, 0.004276631695527330530, 0.004887579080602664702 ),
 .UNSPECIFIED. ) ;
#86350=ORIENTED_EDGE ( 'NONE', *, *, #54587, .F. ) ;
#86359=VERTEX_POINT ( 'NONE', #74324 ) ;
#86369=FACE_OUTER_BOUND ( 'NONE', #60535, .T. ) ;
#86380=CYLINDRICAL_SURFACE ( 'NONE', #51810, 24.00000000000001066 ) ;
#86384=DIRECTION ( 'NONE',  ( 0.5370370370370448621, 0.000000000000000000, -0.8435586647355782786 ) ) ;
#86387=LINE ( 'NONE', #50889, #52698 ) ;
#86391=CARTESIAN_POINT ( 'NONE',  ( 214.2238915819278589, 32.98517505407394168, 10.50000000000000000 ) ) ;
#86401=DIRECTION ( 'NONE',  ( 0.000000000000000000, 1.000000000000000000, 0.000000000000000000 ) ) ;
#86419=AXIS2_PLACEMENT_3D ( 'NONE', #59485, #39885, #31067 ) ;
#86421=VECTOR ( 'NONE', #61435, 1000.000000000000000 ) ;
#86440=PLANE ( 'NONE',  #71678 ) ;
#86444=ORIENTED_EDGE ( 'NONE', *, *, #27400, .F. ) ;
#86455=ORIENTED_EDGE ( 'NONE', *, *, #67723, .T. ) ;
#86459=CARTESIAN_POINT ( 'NONE',  ( 156.3051094419640492, 18.69637893470003220, 10.18000837680918913 ) ) ;
#86471=CARTESIAN_POINT ( 'NONE',  ( 156.8041522122653930, 275.0000000000000568, 16.89672165344857646 ) ) ;
#86480=AXIS2_PLACEMENT_3D ( 'NONE', #44682, #17215, #53179 ) ;
#86484=AXIS2_PLACEMENT_3D ( 'NONE', #1972, #81492, #30864 ) ;
#86487=CARTESIAN_POINT ( 'NONE',  ( 196.7737507933381949, 25.83989517275634995, 12.61380704606697023 ) ) ;
#86488=EDGE_CURVE ( 'NONE', #19459, #38465, #34023, .T. ) ;
#86489=EDGE_CURVE ( 'NONE', #17165, #90976, #32462, .T. ) ;
#86490=DIRECTION ( 'NONE',  ( 0.000000000000000000, 1.000000000000000000, 0.000000000000000000 ) ) ;
#86492=AXIS2_PLACEMENT_3D ( 'NONE', #20401, #90907, #4771 ) ;
#86504=CARTESIAN_POINT ( 'NONE',  ( 152.4536156746142410, 250.0000000000000568, 14.50000000000000000 ) ) ;
#86513=FACE_OUTER_BOUND ( 'NONE', #10426, .T. ) ;
#86518=CARTESIAN_POINT ( 'NONE',  ( 155.2961426000110805, 19.82592759221843792, -13.64628225442899456 ) ) ;
#86529=CARTESIAN_POINT ( 'NONE',  ( 197.2116943569230330, 250.5000000000000568, -12.92446933126074882 ) ) ;
#86531=FACE_OUTER_BOUND ( 'NONE', #52447, .T. ) ;
#86540=ORIENTED_EDGE ( 'NONE', *, *, #71165, .F. ) ;
#86541=CARTESIAN_POINT ( 'NONE',  ( 195.0325088190295162, 41.78303943026349998, 13.56014590831882671 ) ) ;
#86547=VERTEX_POINT ( 'NONE', #2830 ) ;
#86554=DIRECTION ( 'NONE',  ( 0.000000000000000000, 0.000000000000000000, 1.000000000000000000 ) ) ;
#86560=ORIENTED_EDGE ( 'NONE', *, *, #79269, .F. ) ;
#86565=CIRCLE ( 'NONE', #73000, 0.5000000000000004441 ) ;
#86577=CARTESIAN_POINT ( 'NONE',  ( 157.3402357740650075, 250.0000000000000568, 16.90039380915369094 ) ) ;
#86592=ORIENTED_EDGE ( 'NONE', *, *, #59069, .F. ) ;
#86598=EDGE_CURVE ( 'NONE', #23364, #85888, #79392, .T. ) ;
#86610=EDGE_CURVE ( 'NONE', #46837, #71459, #65755, .T. ) ;
#86611=CARTESIAN_POINT ( 'NONE',  ( 160.5350683151633291, 250.0000000000000568, 20.22542485937379908 ) ) ;
#86619=CIRCLE ( 'NONE', #17080, 1.000000000000000888 ) ;
#86622=CARTESIAN_POINT ( 'NONE',  ( 199.4392256788250677, 65.82574266882505754, 7.741079165001062634 ) ) ;
#86623=VECTOR ( 'NONE', #73129, 1000.000000000000000 ) ;
#86635=CARTESIAN_POINT ( 'NONE',  ( 208.6208076322478746, 32.98517505407394168, 14.49999999999999822 ) ) ;
#86638=CARTESIAN_POINT ( 'NONE',  ( 196.8803347170859865, 73.40565171261611965, -12.50000000000000355 ) ) ;
#86645=AXIS2_PLACEMENT_3D ( 'NONE', #89839, #25907, #9363 ) ;
#86649=FACE_OUTER_BOUND ( 'NONE', #18238, .T. ) ;
#86652=CARTESIAN_POINT ( 'NONE',  ( 165.2494399300530290, 8.542400036368780647, 9.000000000000001776 ) ) ;
#86665=LINE ( 'NONE', #8067, #21868 ) ;
#86677=ORIENTED_EDGE ( 'NONE', *, *, #90853, .F. ) ;
#86686=ORIENTED_EDGE ( 'NONE', *, *, #24497, .T. ) ;
#86687=ORIENTED_EDGE ( 'NONE', *, *, #66535, .T. ) ;
#86688=AXIS2_PLACEMENT_3D ( 'NONE', #76850, #11977, #62671 ) ;
#86690=AXIS2_PLACEMENT_3D ( 'NONE', #86135, #35024, #56349 ) ;
#86695=LINE ( 'NONE', #544, #92865 ) ;
#86707=ORIENTED_EDGE ( 'NONE', *, *, #91432, .T. ) ;
#86713=ADVANCED_FACE ( 'NONE', ( #8984 ), #52124, .T. ) ;
#86721=AXIS2_PLACEMENT_3D ( 'NONE', #68714, #75800, #25602 ) ;
#86737=CARTESIAN_POINT ( 'NONE',  ( 175.2296996224750103, 20.99999999999998934, 0.000000000000000000 ) ) ;
#86743=CARTESIAN_POINT ( 'NONE',  ( 209.4046159701566410, 38.09026110277402211, 12.05941621939746966 ) ) ;
#86745=CARTESIAN_POINT ( 'NONE',  ( 197.2116943569230330, 250.5000000000000568, -11.92446933126074882 ) ) ;
#86748=CARTESIAN_POINT ( 'NONE',  ( 199.6150009768959706, 250.5000000000000568, -2.367926910627514037 ) ) ;
#86749=CARTESIAN_POINT ( 'NONE',  ( 157.4471379844592036, 15.78783268421870645, -9.037979834338015550 ) ) ;
#86758=VERTEX_POINT ( 'NONE', #53488 ) ;
#86762=CARTESIAN_POINT ( 'NONE',  ( 193.9153122143737562, 215.0000000000000568, 17.21343741151142126 ) ) ;
#86764=ORIENTED_EDGE ( 'NONE', *, *, #34566, .T. ) ;
#86766=AXIS2_PLACEMENT_3D ( 'NONE', #62546, #75789, #12329 ) ;
#86774=ORIENTED_EDGE ( 'NONE', *, *, #73224, .F. ) ;
#86777=TOROIDAL_SURFACE ( 'NONE', #38378, 27.00000000000000355, 3.000000000000000000 ) ;
#86783=DIRECTION ( 'NONE',  ( 0.6573509547581669610, 0.1665889405894028785, -0.7349407099568147084 ) ) ;
#86796=VECTOR ( 'NONE', #89548, 1000.000000000000000 ) ;
#86830=ORIENTED_EDGE ( 'NONE', *, *, #86610, .T. ) ;
#86835=AXIS2_PLACEMENT_3D ( 'NONE', #68817, #25702, #76382 ) ;
#86841=CARTESIAN_POINT ( 'NONE',  ( 0.000000000000000000, 0.000000000000000000, 9.000000000000001776 ) ) ;
#86844=CIRCLE ( 'NONE', #46002, 0.4999999999999926170 ) ;
#86847=CARTESIAN_POINT ( 'NONE',  ( 209.5381921119887636, 36.46041812331149856, 14.69807322781370118 ) ) ;
#86856=CARTESIAN_POINT ( 'NONE',  ( 155.4162060973606287, 20.04122387618983936, 15.25295451849726902 ) ) ;
#86909=UNCERTAINTY_MEASURE_WITH_UNIT (LENGTH_MEASURE( 1.000000000000000082E-05 ), #60100, 'distance_accuracy_value', 'NONE');
#86914=AXIS2_PLACEMENT_3D ( 'NONE', #61515, #61966, #45876 ) ;
#86937=ORIENTED_EDGE ( 'NONE', *, *, #17248, .T. ) ;
#86939=CARTESIAN_POINT ( 'NONE',  ( 197.1933712184921603, 24.89666632552609826, 12.64285714285713169 ) ) ;
#86945=DIRECTION ( 'NONE',  ( 0.000000000000000000, 0.000000000000000000, -1.000000000000000000 ) ) ;
#86946=DIRECTION ( 'NONE',  ( 0.5729786897769378884, 0.000000000000000000, -0.8195702660916291959 ) ) ;
#86948=ORIENTED_EDGE ( 'NONE', *, *, #71792, .F. ) ;
#86964=CARTESIAN_POINT ( 'NONE',  ( 198.7945540180826072, 289.2625417210226146, -6.475712835924320565 ) ) ;
#86965=CARTESIAN_POINT ( 'NONE',  ( 207.0546088034498666, 35.99211966507625959, 14.99999999999999822 ) ) ;
#86981=CARTESIAN_POINT ( 'NONE',  ( 211.4629471475955427, 32.98517505407394168, 14.26380412667038655 ) ) ;
#86987=DIRECTION ( 'NONE',  ( 0.000000000000000000, 0.000000000000000000, 1.000000000000000000 ) ) ;
#86992=CIRCLE ( 'NONE', #82404, 2.000000000000001776 ) ;
#87004=ORIENTED_EDGE ( 'NONE', *, *, #57049, .T. ) ;
#87007=DIRECTION ( 'NONE',  ( -0.000000000000000000, -1.000000000000000000, -0.000000000000000000 ) ) ;
#87017=EDGE_LOOP ( 'NONE', ( #86223, #47655, #32566, #1634 ) ) ;
#87018=CARTESIAN_POINT ( 'NONE',  ( 196.8702642586142986, 40.96915988761479355, 12.42857142857142350 ) ) ;
#87028=CARTESIAN_POINT ( 'NONE',  ( 209.6287663260175975, 29.00782453271232697, 12.09245862095555601 ) ) ;
#87034=ADVANCED_FACE ( 'NONE', ( #47284 ), #19780, .T. ) ;
#87042=ORIENTED_EDGE ( 'NONE', *, *, #9842, .F. ) ;
#87049=LINE ( 'NONE', #52461, #80920 ) ;
#87066=ORIENTED_EDGE ( 'NONE', *, *, #36488, .F. ) ;
#87067=ORIENTED_EDGE ( 'NONE', *, *, #70399, .T. ) ;
#87068=DIRECTION ( 'NONE',  ( 1.000000000000000000, 0.000000000000000000, -0.000000000000000000 ) ) ;
#87084=DIRECTION ( 'NONE',  ( -0.5877852522924792433, 0.000000000000000000, -0.8090169943749430104 ) ) ;
#87097=CARTESIAN_POINT ( 'NONE',  ( 200.4892204403996345, 64.44609543878858915, 7.254661561168179951 ) ) ;
#87109=CARTESIAN_POINT ( 'NONE',  ( 196.8803347170859865, 73.40565171261611965, -12.50000000000000000 ) ) ;
#87110=DIRECTION ( 'NONE',  ( 0.000000000000000000, 0.000000000000000000, -1.000000000000000000 ) ) ;
#87118=CARTESIAN_POINT ( 'NONE',  ( 170.2305261370685798, 275.0000000000000568, -24.90909090909090295 ) ) ;
#87120=DIRECTION ( 'NONE',  ( 0.000000000000000000, 0.000000000000000000, 1.000000000000000000 ) ) ;
#87133=CARTESIAN_POINT ( 'NONE',  ( 202.8019728163925492, 61.40723988820082013, -6.999999999999999112 ) ) ;
#87146=ORIENTED_EDGE ( 'NONE', *, *, #22273, .T. ) ;
#87155=ORIENTED_EDGE ( 'NONE', *, *, #64747, .F. ) ;
#87161=CARTESIAN_POINT ( 'NONE',  ( 138.6539576904058606, 250.5000000000000568, -10.49999999999999822 ) ) ;
#87174=CARTESIAN_POINT ( 'NONE',  ( 195.2948010944529926, 25.74157531710192259, 13.17633069842077909 ) ) ;
#87198=CARTESIAN_POINT ( 'NONE',  ( 196.8803347170859865, 20.19615242270636557, -12.49999999999999289 ) ) ;
#87209=DIRECTION ( 'NONE',  ( 0.000000000000000000, 0.000000000000000000, 1.000000000000000000 ) ) ;
#87210=FACE_OUTER_BOUND ( 'NONE', #38262, .T. ) ;
#87221=DIRECTION ( 'NONE',  ( 1.000000000000000000, -0.000000000000000000, 5.880589007913310608E-16 ) ) ;
#87224=CARTESIAN_POINT ( 'NONE',  ( 197.2554367620029439, 24.42492926436516498, 11.92185234729253374 ) ) ;
#87233=ORIENTED_EDGE ( 'NONE', *, *, #22107, .T. ) ;
#87235=VECTOR ( 'NONE', #32658, 1000.000000000000000 ) ;
#87239=CARTESIAN_POINT ( 'NONE',  ( 154.7156223832783724, 19.57420759269780319, 12.98093464719297074 ) ) ;
#87240=ADVANCED_FACE ( 'NONE', ( #61993 ), #41595, .F. ) ;
#87243=DIRECTION ( 'NONE',  ( -0.000000000000000000, -0.000000000000000000, 1.000000000000000000 ) ) ;
#87257=ORIENTED_EDGE ( 'NONE', *, *, #30387, .F. ) ;
#87290=VERTEX_POINT ( 'NONE', #20317 ) ;
#87310=CYLINDRICAL_SURFACE ( 'NONE', #23165, 0.5000000000000004441 ) ;
#87313=CARTESIAN_POINT ( 'NONE',  ( 157.4851178187871312, 15.00000000000000000, -7.000000000000000888 ) ) ;
#87329=ORIENTED_EDGE ( 'NONE', *, *, #49529, .T. ) ;
#87334=CARTESIAN_POINT ( 'NONE',  ( 208.9735924857420741, 36.55662354001872671, 13.48907645363297547 ) ) ;
#87375=VECTOR ( 'NONE', #48341, 1000.000000000000000 ) ;
#87398=CARTESIAN_POINT ( 'NONE',  ( 209.5654368701818271, 27.96016292911928502, 12.08763307006249832 ) ) ;
#87399=LINE ( 'NONE', #59955, #54717 ) ;
#87403=EDGE_LOOP ( 'NONE', ( #60728, #57463, #70538, #75289 ) ) ;
#87404=CARTESIAN_POINT ( 'NONE',  ( 200.7568414405312751, 39.78480925505072463, 8.999999999999998224 ) ) ;
#87417=CARTESIAN_POINT ( 'NONE',  ( 210.6911063078042901, 0.9999999999999991118, -7.166232077703399206 ) ) ;
#87432=FACE_OUTER_BOUND ( 'NONE', #42339, .T. ) ;
#87434=CYLINDRICAL_SURFACE ( 'NONE', #56479, 3.000000000000000000 ) ;
#87435=CIRCLE ( 'NONE', #34545, 2.000000000000010658 ) ;
#87441=CARTESIAN_POINT ( 'NONE',  ( 207.4724402404594343, 29.73442829110639352, 14.90057469441957672 ) ) ;
#87444=DIRECTION ( 'NONE',  ( 0.9531768234071978929, -0.3024135303179465439, 0.000000000000000000 ) ) ;
#87456=EDGE_LOOP ( 'NONE', ( #1778, #5576, #45574 ) ) ;
#87459=DIRECTION ( 'NONE',  ( -0.000000000000000000, -1.000000000000000000, -0.000000000000000000 ) ) ;
#87468=VERTEX_POINT ( 'NONE', #55283 ) ;
#87480=CARTESIAN_POINT ( 'NONE',  ( 169.8384340989974532, 250.0000000000000568, -24.41176470588234437 ) ) ;
#87484=ORIENTED_EDGE ( 'NONE', *, *, #133, .F. ) ;
#87499=DIRECTION ( 'NONE',  ( 0.000000000000000000, 1.000000000000000000, 0.000000000000000000 ) ) ;
#87503=LINE ( 'NONE', #43956, #74555 ) ;
#87504=AXIS2_PLACEMENT_3D ( 'NONE', #73602, #82555, #31444 ) ;
#87513=CARTESIAN_POINT ( 'NONE',  ( 200.2349812190172713, 66.43136063442170780, -7.741079165001072404 ) ) ;
#87519=VERTEX_POINT ( 'NONE', #20226 ) ;
#87520=CARTESIAN_POINT ( 'NONE',  ( 196.0490226090805379, 41.97839894083266188, 13.84150264294241239 ) ) ;
#87522=( BOUNDED_CURVE ( )  B_SPLINE_CURVE ( 3, ( #72485, #56901, #7601, #516 ),
 .UNSPECIFIED., .F., .F. ) 
 B_SPLINE_CURVE_WITH_KNOTS ( ( 4, 4 ),
 ( 5.134959379131573520, 6.283185307179586232 ),
 .UNSPECIFIED. ) 
 CURVE ( )  GEOMETRIC_REPRESENTATION_ITEM ( )  RATIONAL_B_SPLINE_CURVE ( ( 1.000000000000000000, 0.8931162488198156613, 0.8931162488198156613, 1.000000000000000000 ) ) 
 REPRESENTATION_ITEM ( '' )  );
#87532=CARTESIAN_POINT ( 'NONE',  ( 175.2296996224750103, 20.99999999999998934, -25.00000000000000355 ) ) ;
#87533=CARTESIAN_POINT ( 'NONE',  ( 209.7513585654922679, 305.7026273589066818, -40.00000000000000711 ) ) ;
#87542=DIRECTION ( 'NONE',  ( -1.000000000000000000, -0.000000000000000000, 0.000000000000000000 ) ) ;
#87545=DIRECTION ( 'NONE',  ( 0.000000000000000000, 1.000000000000000000, 0.000000000000000000 ) ) ;
#87547=CARTESIAN_POINT ( 'NONE',  ( 152.4536156746142410, 130.6065089285656313, 11.50000000000000000 ) ) ;
#87554=EDGE_CURVE ( 'NONE', #5855, #2870, #53279, .T. ) ;
#87556=EDGE_CURVE ( 'NONE', #90952, #57748, #36356, .T. ) ;
#87561=DIRECTION ( 'NONE',  ( 1.000000000000000000, -0.000000000000000000, 0.000000000000000000 ) ) ;
#87571=ORIENTED_EDGE ( 'NONE', *, *, #69946, .F. ) ;
#87575=CARTESIAN_POINT ( 'NONE',  ( 175.2296996224750103, 133.0000000000000000, 0.000000000000000000 ) ) ;
#87587=LINE ( 'NONE', #71086, #83818 ) ;
#87588=DIRECTION ( 'NONE',  ( 0.000000000000000000, 0.000000000000000000, 1.000000000000000000 ) ) ;
#87591=DIRECTION ( 'NONE',  ( 0.000000000000000000, 0.000000000000000000, 1.000000000000000000 ) ) ;
#87609=VERTEX_POINT ( 'NONE', #93118 ) ;
#87615=FACE_OUTER_BOUND ( 'NONE', #12256, .T. ) ;
#87630=CARTESIAN_POINT ( 'NONE',  ( 175.2296996224750103, 20.00000000000000000, 0.000000000000000000 ) ) ;
#87635=AXIS2_PLACEMENT_3D ( 'NONE', #40273, #69189, #48325 ) ;
#87642=CIRCLE ( 'NONE', #58944, 2.500000000000000444 ) ;
#87654=DIRECTION ( 'NONE',  ( 0.000000000000000000, 1.000000000000000000, 0.000000000000000000 ) ) ;
#87659=EDGE_CURVE ( 'NONE', #37341, #55975, #14062, .T. ) ;
#87662=DIRECTION ( 'NONE',  ( -0.000000000000000000, -1.000000000000000000, -0.000000000000000000 ) ) ;
#87664=CARTESIAN_POINT ( 'NONE',  ( 198.1541494672131876, 25.06826132699710996, 11.52973355076513684 ) ) ;
#87667=CARTESIAN_POINT ( 'NONE',  ( 209.1990615267463056, 35.77166376090755762, 14.26711941829674579 ) ) ;
#87677=VERTEX_POINT ( 'NONE', #55747 ) ;
#87678=DIRECTION ( 'NONE',  ( 0.000000000000000000, 1.000000000000000000, 0.000000000000000000 ) ) ;
#87693=ADVANCED_FACE ( 'NONE', ( #5565 ), #34436, .T. ) ;
#87694=CARTESIAN_POINT ( 'NONE',  ( 198.7947541974662613, 298.6649591161120156, -6.475578415184554792 ) ) ;
#87698=CARTESIAN_POINT ( 'NONE',  ( 202.9738562182569694, 293.9636489450776367, -59.00000000000003553 ) ) ;
#87701=VECTOR ( 'NONE', #21268, 1000.000000000000000 ) ;
#87707=AXIS2_PLACEMENT_3D ( 'NONE', #42307, #4931, #76902 ) ;
#87713=ORIENTED_EDGE ( 'NONE', *, *, #68670, .F. ) ;
#87736=ORIENTED_EDGE ( 'NONE', *, *, #79684, .T. ) ;
#87743=ORIENTED_EDGE ( 'NONE', *, *, #84671, .T. ) ;
#87761=CARTESIAN_POINT ( 'NONE',  ( 209.0207885866473134, 36.54472185027779574, 14.72030241339632894 ) ) ;
#87769=CARTESIAN_POINT ( 'NONE',  ( 154.0637704119390321, 19.72112694978655867, 13.30738029212317564 ) ) ;
#87771=TOROIDAL_SURFACE ( 'NONE', #6165, 2.103083949679977582, 3.000000000000000000 ) ;
#87776=CARTESIAN_POINT ( 'NONE',  ( 153.5041831715920750, 19.57420759269873045, -11.76949543551211619 ) ) ;
#87778=CARTESIAN_POINT ( 'NONE',  ( 204.6539576904058606, 300.0210572133868823, -5.225551010890672643 ) ) ;
#87782=CARTESIAN_POINT ( 'NONE',  ( 164.6329196456214277, 249.5000000000000568, 23.09031830825855991 ) ) ;
#87789=B_SPLINE_CURVE_WITH_KNOTS ( 'NONE', 3,
 ( #68443, #82174, #24892, #54227 ),
 .UNSPECIFIED., .F., .F.,
 ( 4, 4 ),
 ( 0.0006709229447830969287, 0.0008458583158006164563 ),
 .UNSPECIFIED. ) ;
#87818=ADVANCED_FACE ( 'NONE', ( #78461 ), #12667, .T. ) ;
#87838=CIRCLE ( 'NONE', #15272, 0.4999999999999923395 ) ;
#87851=ORIENTED_EDGE ( 'NONE', *, *, #39617, .F. ) ;
#87858=CARTESIAN_POINT ( 'NONE',  ( 175.2296996224750103, 160.0000000000000568, 0.000000000000000000 ) ) ;
#87868=ADVANCED_FACE ( 'NONE', ( #42449 ), #18883, .T. ) ;
#87876=CARTESIAN_POINT ( 'NONE',  ( 151.4851178187871312, 20.00000000000000000, 3.492110388858666870 ) ) ;
#87884=CARTESIAN_POINT ( 'NONE',  ( 139.1539576904058606, 250.5000000000000568, -10.49999999999999822 ) ) ;
#87889=EDGE_CURVE ( 'NONE', #91480, #35022, #30986, .T. ) ;
#87891=DIRECTION ( 'NONE',  ( -0.000000000000000000, -1.000000000000000000, -0.000000000000000000 ) ) ;
#87893=CARTESIAN_POINT ( 'NONE',  ( 196.8803347170859865, 250.0000000000000568, -12.49999999999999289 ) ) ;
#87897=EDGE_CURVE ( 'NONE', #63820, #29329, #43084, .T. ) ;
#87900=DIRECTION ( 'NONE',  ( 0.000000000000000000, -1.000000000000000000, 0.000000000000000000 ) ) ;
#87905=AXIS2_PLACEMENT_3D ( 'NONE', #60913, #75115, #25834 ) ;
#87917=ORIENTED_EDGE ( 'NONE', *, *, #78116, .F. ) ;
#87918=CARTESIAN_POINT ( 'NONE',  ( 152.0194914954574870, 20.99319818809533089, 6.266237208439005890 ) ) ;
#87920=CARTESIAN_POINT ( 'NONE',  ( 209.6287663260176259, 29.00782453271233052, 12.90102856104451412 ) ) ;
#87929=ORIENTED_EDGE ( 'NONE', *, *, #29767, .T. ) ;
#87930=CARTESIAN_POINT ( 'NONE',  ( 196.0143093133015384, 42.36571313990104670, 11.99999999999999112 ) ) ;
#87940=CARTESIAN_POINT ( 'NONE',  ( 196.0143093133015384, 73.40565171261611965, -12.00000000000000355 ) ) ;
#87945=ORIENTED_EDGE ( 'NONE', *, *, #75074, .T. ) ;
#87961=ADVANCED_FACE ( 'NONE', ( #58086 ), #29478, .F. ) ;
#87965=CARTESIAN_POINT ( 'NONE',  ( 209.3463111024439343, 0.03396820302666800351, -7.457905934263069803 ) ) ;
#87978=VERTEX_POINT ( 'NONE', #19373 ) ;
#87979=ORIENTED_EDGE ( 'NONE', *, *, #15328, .F. ) ;
#87980=CARTESIAN_POINT ( 'NONE',  ( 199.0883366025630323, 17.54655016014115176, -10.45170682515238170 ) ) ;
#87985=ADVANCED_FACE ( 'NONE', ( #26484 ), #49161, .F. ) ;
#87995=LINE ( 'NONE', #23148, #39784 ) ;
#87996=FACE_OUTER_BOUND ( 'NONE', #57685, .T. ) ;
#88007=ADVANCED_FACE ( 'NONE', ( #4233 ), #52183, .T. ) ;
#88009=DIRECTION ( 'NONE',  ( 0.000000000000000000, 0.000000000000000000, 1.000000000000000000 ) ) ;
#88030=CIRCLE ( 'NONE', #18491, 4.499999999999990230 ) ;
#88033=FACE_OUTER_BOUND ( 'NONE', #13375, .T. ) ;
#88034=AXIS2_PLACEMENT_3D ( 'NONE', #5144, #49159, #14123 ) ;
#88040=STYLED_ITEM('',(#93738),#27724);
#88042=CIRCLE ( 'NONE', #66838, 4.999999999999993783 ) ;
#88048=EDGE_LOOP ( 'NONE', ( #63562, #57512, #26953, #6577 ) ) ;
#88066=( BOUNDED_SURFACE ( )  B_SPLINE_SURFACE ( 3, 2, ( 
 ( #59608, #81347, #2760 ),
 ( #16497, #24525, #31641 ),
 ( #45349, #67170, #2303 ),
 ( #60531, #89369, #17442 ) ),
 .UNSPECIFIED., .F., .F., .F. ) 
 B_SPLINE_SURFACE_WITH_KNOTS ( ( 4, 4 ),
 ( 3, 3 ),
 ( 0.000000000000000000, 0.0009404805950308383440 ),
 ( 0.000000000000000000, 1.000000000000000000 ),
 .UNSPECIFIED. ) 
 GEOMETRIC_REPRESENTATION_ITEM ( )  RATIONAL_B_SPLINE_SURFACE ( (
 ( 1.000000000000000000, 0.7071067811865475727, 1.000000000000000000),
 ( 1.000000000000000000, 0.6851250445827049562, 1.000000000000000000),
 ( 1.000000000000000000, 0.6575897825470939928, 1.000000000000000000),
 ( 1.000000000000000000, 0.6287211027133905450, 1.000000000000000000) ) ) 
 REPRESENTATION_ITEM ( '' )  SURFACE ( )  );
#88073=ORIENTED_EDGE ( 'NONE', *, *, #90062, .T. ) ;
#88092=FACE_OUTER_BOUND ( 'NONE', #23718, .T. ) ;
#88102=DIRECTION ( 'NONE',  ( 1.000000000000000000, 0.000000000000000000, -0.000000000000000000 ) ) ;
#88103=AXIS2_PLACEMENT_3D ( 'NONE', #70892, #64748, #80656 ) ;
#88112=EDGE_LOOP ( 'NONE', ( #77510, #73574, #33963, #68149, #47955 ) ) ;
#88119=CARTESIAN_POINT ( 'NONE',  ( 194.2870706637141609, 27.28231030510911381, 14.58823529411774089 ) ) ;
#88128=CARTESIAN_POINT ( 'NONE',  ( 203.5977283565847813, 62.01285785379744198, 7.000000000000000000 ) ) ;
#88131=DIRECTION ( 'NONE',  ( 1.000000000000000000, 0.000000000000000000, 0.000000000000000000 ) ) ;
#88132=CARTESIAN_POINT ( 'NONE',  ( 0.000000000000000000, 249.5000000000000568, -12.50000000000000000 ) ) ;
#88144=DIRECTION ( 'NONE',  ( -0.6056179655966479336, 0.7957555401921982963, 3.708340515370333519E-17 ) ) ;
#88147=CARTESIAN_POINT ( 'NONE',  ( 157.5411741086738004, 275.0000000000000568, 16.22085278731064761 ) ) ;
#88158=VECTOR ( 'NONE', #56850, 1000.000000000000000 ) ;
#88160=CARTESIAN_POINT ( 'NONE',  ( 165.6062301568830435, 2.982529536179759688, 9.000000000000001776 ) ) ;
#88163=CARTESIAN_POINT ( 'NONE',  ( 183.0442525570908288, 264.6571197653884155, -7.500000000000000000 ) ) ;
#88164=CIRCLE ( 'NONE', #68525, 1.499999999999998446 ) ;
#88174=AXIS2_PLACEMENT_3D ( 'NONE', #1273, #52846, #81723 ) ;
#88180=ORIENTED_EDGE ( 'NONE', *, *, #20867, .T. ) ;
#88185=TOROIDAL_SURFACE ( 'NONE', #70111, 4.500000000000002665, 0.5000000000000000000 ) ;
#88197=VECTOR ( 'NONE', #76145, 1000.000000000000000 ) ;
#88205=EDGE_CURVE ( 'NONE', #47327, #33195, #93023, .T. ) ;
#88207=ORIENTED_EDGE ( 'NONE', *, *, #28072, .T. ) ;
#88211=AXIS2_PLACEMENT_3D ( 'NONE', #21817, #8054, #15169 ) ;
#88216=CARTESIAN_POINT ( 'NONE',  ( 157.4851178187871312, 14.99999999999999645, 9.000000000000000000 ) ) ;
#88236=VECTOR ( 'NONE', #56619, 1000.000000000000000 ) ;
#88243=DIRECTION ( 'NONE',  ( -0.000000000000000000, -1.000000000000000000, -0.000000000000000000 ) ) ;
#88245=AXIS2_PLACEMENT_3D ( 'NONE', #59961, #23947, #45703 ) ;
#88247=CARTESIAN_POINT ( 'NONE',  ( 156.2461366866179731, 19.34073763602959772, -8.651974842892217410 ) ) ;
#88250=CARTESIAN_POINT ( 'NONE',  ( 154.0561329571298756, 19.33057573605838186, -12.42898486165725203 ) ) ;
#88252=PLANE ( 'NONE',  #49740 ) ;
#88256=CARTESIAN_POINT ( 'NONE',  ( 196.0143093133017658, 19.33012701892200624, -12.49999999999967315 ) ) ;
#88260=AXIS2_PLACEMENT_3D ( 'NONE', #80003, #29362, #49719 ) ;
#88273=DIRECTION ( 'NONE',  ( 0.000000000000000000, 0.000000000000000000, 1.000000000000000000 ) ) ;
#88277=TOROIDAL_SURFACE ( 'NONE', #38396, 24.50000000000000355, 0.5000000000000000000 ) ;
#88302=ORIENTED_EDGE ( 'NONE', *, *, #17026, .F. ) ;
#88318=EDGE_CURVE ( 'NONE', #74853, #49791, #36658, .T. ) ;
#88322=ORIENTED_EDGE ( 'NONE', *, *, #75906, .T. ) ;
#88328=EDGE_LOOP ( 'NONE', ( #83750, #35023, #79168, #42333 ) ) ;
#88329=DIRECTION ( 'NONE',  ( -0.000000000000000000, -1.000000000000000000, -0.000000000000000000 ) ) ;
#88330=AXIS2_PLACEMENT_3D ( 'NONE', #77277, #19507, #27556 ) ;
#88333=AXIS2_PLACEMENT_3D ( 'NONE', #84271, #42113, #18477 ) ;
#88337=DIRECTION ( 'NONE',  ( -0.000000000000000000, -0.000000000000000000, -1.000000000000000000 ) ) ;
#88341=AXIS2_PLACEMENT_3D ( 'NONE', #62342, #68504, #47162 ) ;
#88363=CARTESIAN_POINT ( 'NONE',  ( 152.4536156746142410, 275.5000000000000568, -14.50000000000000000 ) ) ;
#88367=CARTESIAN_POINT ( 'NONE',  ( 219.8344101925596021, 3.000000000000000000, 9.000000000000001776 ) ) ;
#88368=DIRECTION ( 'NONE',  ( -1.000000000000000000, 0.000000000000000000, -0.000000000000000000 ) ) ;
#88386=CARTESIAN_POINT ( 'NONE',  ( 175.2296996224750103, 154.6894116713782807, -20.15985230015483154 ) ) ;
#88402=CARTESIAN_POINT ( 'NONE',  ( 198.5952592410606314, 68.60901277742570414, 10.61452171551476198 ) ) ;
#88412=AXIS2_PLACEMENT_3D ( 'NONE', #62954, #34519, #90828 ) ;
#88427=CARTESIAN_POINT ( 'NONE',  ( 175.2296996224750103, 161.0000000000000853, 0.000000000000000000 ) ) ;
#88447=EDGE_CURVE ( 'NONE', #14856, #16112, #70047, .T. ) ;
#88449=DIRECTION ( 'NONE',  ( 0.000000000000000000, -0.000000000000000000, 1.000000000000000000 ) ) ;
#88463=ORIENTED_EDGE ( 'NONE', *, *, #70954, .F. ) ;
#88464=EDGE_CURVE ( 'NONE', #30954, #15639, #22813, .T. ) ;
#88465=CARTESIAN_POINT ( 'NONE',  ( 201.2104617360081704, 15.00000000000001421, -10.00000000000000178 ) ) ;
#88494=CARTESIAN_POINT ( 'NONE',  ( 140.6539576904058606, 275.0000000000000568, 10.50000000000000000 ) ) ;
#88504=FACE_OUTER_BOUND ( 'NONE', #92528, .T. ) ;
#88527=ORIENTED_EDGE ( 'NONE', *, *, #57879, .T. ) ;
#88531=CARTESIAN_POINT ( 'NONE',  ( 205.7381008070598227, 0.000000000000000000, 7.000000000000000000 ) ) ;
#88532=EDGE_CURVE ( 'NONE', #6460, #16264, #28020, .T. ) ;
#88535=FACE_OUTER_BOUND ( 'NONE', #79624, .T. ) ;
#88543=VECTOR ( 'NONE', #43839, 1000.000000000000000 ) ;
#88544=EDGE_LOOP ( 'NONE', ( #40272, #62020, #56075 ) ) ;
#88580=CARTESIAN_POINT ( 'NONE',  ( 199.0061125298537377, 250.5000000000000568, -7.725424859374024678 ) ) ;
#88590=CARTESIAN_POINT ( 'NONE',  ( 157.7277585059063938, 1.242640687119284992, 9.999999999999998224 ) ) ;
#88598=FACE_OUTER_BOUND ( 'NONE', #42517, .T. ) ;
#88601=CARTESIAN_POINT ( 'NONE',  ( 204.6539576904058606, 293.9636489450775230, 0.000000000000000000 ) ) ;
#88604=LINE ( 'NONE', #1978, #92581 ) ;
#88605=DIRECTION ( 'NONE',  ( 1.000000000000000000, 0.000000000000000000, -0.000000000000000000 ) ) ;
#88613=EDGE_CURVE ( 'NONE', #56036, #74598, #58302, .T. ) ;
#88615=ORIENTED_EDGE ( 'NONE', *, *, #57514, .F. ) ;
#88616=CARTESIAN_POINT ( 'NONE',  ( 165.7865175155837676, 3.000000000000000000, 10.00000000000000000 ) ) ;
#88619=CARTESIAN_POINT ( 'NONE',  ( 195.5192339169639979, 26.76774044649046758, 14.92136003405341249 ) ) ;
#88631=CARTESIAN_POINT ( 'NONE',  ( 156.4972887742121088, 15.41695093167224861, 9.987829044572988479 ) ) ;
#88634=CARTESIAN_POINT ( 'NONE',  ( 175.2296996224750103, 134.0000000000000284, -24.00000000000001066 ) ) ;
#88648=VERTEX_POINT ( 'NONE', #12764 ) ;
#88651=ORIENTED_EDGE ( 'NONE', *, *, #25921, .T. ) ;
#88661=ORIENTED_EDGE ( 'NONE', *, *, #31412, .F. ) ;
#88671=ORIENTED_EDGE ( 'NONE', *, *, #88447, .T. ) ;
#88682=EDGE_CURVE ( 'NONE', #62086, #54214, #32511, .T. ) ;
#88683=EDGE_LOOP ( 'NONE', ( #73349, #72571, #175, #20986 ) ) ;
#88694=DIRECTION ( 'NONE',  ( 0.9998346970812742596, 0.000000000000000000, 0.01818181818181330636 ) ) ;
#88697=DIRECTION ( 'NONE',  ( -0.000000000000000000, -1.000000000000000000, -0.000000000000000000 ) ) ;
#88700=DIRECTION ( 'NONE',  ( 0.000000000000000000, 0.000000000000000000, 1.000000000000000000 ) ) ;
#88707=CARTESIAN_POINT ( 'NONE',  ( 175.2296996224750103, 134.0000000000000284, -24.00000000000001066 ) ) ;
#88710=DIRECTION ( 'NONE',  ( -0.000000000000000000, -0.000000000000000000, 1.000000000000000000 ) ) ;
#88714=DIRECTION ( 'NONE',  ( -0.000000000000000000, -1.000000000000000000, -0.000000000000000000 ) ) ;
#88732=EDGE_CURVE ( 'NONE', #5311, #16264, #48711, .T. ) ;
#88735=CARTESIAN_POINT ( 'NONE',  ( 209.8616357346614905, 36.89613957940296274, 12.09245862095555601 ) ) ;
#88753=DIRECTION ( 'NONE',  ( 0.000000000000000000, -0.7071067811865584529, -0.7071067811865364705 ) ) ;
#88767=ORIENTED_EDGE ( 'NONE', *, *, #19699, .F. ) ;
#88786=ORIENTED_EDGE ( 'NONE', *, *, #57795, .T. ) ;
#88799=VERTEX_POINT ( 'NONE', #71934 ) ;
#88813=EDGE_CURVE ( 'NONE', #52100, #72640, #46314, .T. ) ;
#88823=PLANE ( 'NONE',  #50351 ) ;
#88828=CARTESIAN_POINT ( 'NONE',  ( 140.0681712527789671, 131.0000000000000568, 11.50000000000000000 ) ) ;
#88831=PLANE ( 'NONE',  #17108 ) ;
#88838=LINE ( 'NONE', #11181, #38320 ) ;
#88856=CARTESIAN_POINT ( 'NONE',  ( 199.8307606272909993, 66.96248882677818415, 8.111107179099439790 ) ) ;
#88880=VECTOR ( 'NONE', #80975, 1000.000000000000000 ) ;
#88883=VERTEX_POINT ( 'NONE', #44408 ) ;
#88900=CARTESIAN_POINT ( 'NONE',  ( 161.2494399300530290, 8.542400036368780647, 9.974999999999996092 ) ) ;
#88913=ORIENTED_EDGE ( 'NONE', *, *, #43587, .T. ) ;
#88914=EDGE_LOOP ( 'NONE', ( #71494, #8660, #81104, #49398 ) ) ;
#88915=CARTESIAN_POINT ( 'NONE',  ( 201.2104617360081704, 15.00000000000001421, -10.00000000000000178 ) ) ;
#88931=CARTESIAN_POINT ( 'NONE',  ( 156.1711927057158960, 19.99999999999999645, -14.66327707482027343 ) ) ;
#88939=CARTESIAN_POINT ( 'NONE',  ( 211.1232656141943949, 0.000000000000000000, -7.000000000000000000 ) ) ;
#88944=CARTESIAN_POINT ( 'NONE',  ( 0.000000000000000000, 0.000000000000000000, -7.500000000000000000 ) ) ;
#88946=CYLINDRICAL_SURFACE ( 'NONE', #92863, 4.999999999999993783 ) ;
#88967=VERTEX_POINT ( 'NONE', #28035 ) ;
#88968=CARTESIAN_POINT ( 'NONE',  ( 189.9243309297870610, 249.5000000000000568, 25.22542485937348644 ) ) ;
#88979=VERTEX_POINT ( 'NONE', #58657 ) ;
#88982=CARTESIAN_POINT ( 'NONE',  ( 210.3152560301384142, 38.32590481451376263, 10.50000000000000000 ) ) ;
#88984=CARTESIAN_POINT ( 'NONE',  ( 204.6539576904058606, 293.9636489450775230, 7.999911143031724237 ) ) ;
#89004=ORIENTED_EDGE ( 'NONE', *, *, #11508, .T. ) ;
#89022=ORIENTED_EDGE ( 'NONE', *, *, #81029, .T. ) ;
#89041=EDGE_CURVE ( 'NONE', #64853, #63422, #87049, .T. ) ;
#89046=CARTESIAN_POINT ( 'NONE',  ( 152.4536156746142410, 250.5000000000000568, 14.50000000000000000 ) ) ;
#89053=DIRECTION ( 'NONE',  ( 0.000000000000000000, 0.000000000000000000, 1.000000000000000000 ) ) ;
#89055=LINE ( 'NONE', #66840, #72528 ) ;
#89058=CARTESIAN_POINT ( 'NONE',  ( 160.5350683151633291, 275.0000000000000568, 20.22542485937379908 ) ) ;
#89067=EDGE_CURVE ( 'NONE', #88967, #31159, #8329, .T. ) ;
#89069=ORIENTED_EDGE ( 'NONE', *, *, #34302, .T. ) ;
#89073=DIRECTION ( 'NONE',  ( 0.000000000000000000, 1.000000000000000000, 0.000000000000000000 ) ) ;
#89085=FACE_BOUND ( 'NONE', #93090, .T. ) ;
#89086=FACE_OUTER_BOUND ( 'NONE', #19815, .T. ) ;
#89102=ORIENTED_EDGE ( 'NONE', *, *, #12755, .T. ) ;
#89105=ORIENTED_EDGE ( 'NONE', *, *, #48291, .T. ) ;
#89127=ORIENTED_EDGE ( 'NONE', *, *, #78996, .F. ) ;
#89134=ORIENTED_EDGE ( 'NONE', *, *, #36204, .T. ) ;
#89135=CARTESIAN_POINT ( 'NONE',  ( 157.4787282879766508, 15.38390992556648484, 9.006389530800610999 ) ) ;
#89138=EDGE_CURVE ( 'NONE', #93327, #2870, #43146, .T. ) ;
#89140=ORIENTED_EDGE ( 'NONE', *, *, #41260, .T. ) ;
#89141=VERTEX_POINT ( 'NONE', #81335 ) ;
#89143=B_SPLINE_CURVE_WITH_KNOTS ( 'NONE', 3,
 ( #74724, #31633, #87965, #900, #1814, #9365 ),
 .UNSPECIFIED., .F., .F.,
 ( 4, 2, 4 ),
 ( 0.002739916521960775175, 0.004109700271224535004, 0.005479484020488295699 ),
 .UNSPECIFIED. ) ;
#89153=DIRECTION ( 'NONE',  ( -0.000000000000000000, -1.000000000000000000, -0.000000000000000000 ) ) ;
#89158=DIRECTION ( 'NONE',  ( 0.000000000000000000, 1.000000000000000000, 0.000000000000000000 ) ) ;
#89163=FACE_OUTER_BOUND ( 'NONE', #64106, .T. ) ;
#89164=CARTESIAN_POINT ( 'NONE',  ( 160.5350683151633291, 275.0000000000000568, 15.22542485937381329 ) ) ;
#89170=DIRECTION ( 'NONE',  ( -0.000000000000000000, -0.000000000000000000, 1.000000000000000000 ) ) ;
#89187=LINE ( 'NONE', #38066, #27311 ) ;
#89197=EDGE_CURVE ( 'NONE', #55580, #64501, #20440, .T. ) ;
#89222=EDGE_LOOP ( 'NONE', ( #35187, #29901, #66247 ) ) ;
#89224=ORIENTED_EDGE ( 'NONE', *, *, #41709, .T. ) ;
#89251=AXIS2_PLACEMENT_3D ( 'NONE', #28671, #21555, #65612 ) ;
#89253=DIRECTION ( 'NONE',  ( 0.000000000000000000, 0.000000000000000000, 1.000000000000000000 ) ) ;
#89258=DIRECTION ( 'NONE',  ( -0.000000000000000000, -1.000000000000000000, -0.000000000000000000 ) ) ;
#89286=CARTESIAN_POINT ( 'NONE',  ( 139.6539576904058606, 131.4142135623731633, 11.08578643762690596 ) ) ;
#89310=ADVANCED_FACE ( 'NONE', ( #46739 ), #4606, .T. ) ;
#89313=ORIENTED_EDGE ( 'NONE', *, *, #57049, .F. ) ;
#89317=TOROIDAL_SURFACE ( 'NONE', #137, 24.50000000000000355, 0.5000000000000000000 ) ;
#89341=VERTEX_POINT ( 'NONE', #45811 ) ;
#89350=EDGE_LOOP ( 'NONE', ( #35911, #53883, #60868, #79741, #40856 ) ) ;
#89355=FACE_OUTER_BOUND ( 'NONE', #49464, .T. ) ;
#89358=CARTESIAN_POINT ( 'NONE',  ( 222.8344101925596306, 35.72494958537217968, 10.00000000000000000 ) ) ;
#89359=CARTESIAN_POINT ( 'NONE',  ( 200.4551663812866025, 64.49084098423909950, 2.633798379907748455 ) ) ;
#89368=EDGE_CURVE ( 'NONE', #50728, #20922, #5380, .T. ) ;
#89369=CARTESIAN_POINT ( 'NONE',  ( 207.8643778022844231, 35.72636131987244568, 15.02863188060211641 ) ) ;
#89373=ORIENTED_EDGE ( 'NONE', *, *, #85025, .F. ) ;
#89389=LINE ( 'NONE', #24543, #62481 ) ;
#89390=CARTESIAN_POINT ( 'NONE',  ( 155.2899061951603983, 19.82375796246930477, -13.63853015639874577 ) ) ;
#89399=CARTESIAN_POINT ( 'NONE',  ( 180.7149167944524493, 8.542400036368780647, 10.00000000000000178 ) ) ;
#89405=CARTESIAN_POINT ( 'NONE',  ( 193.9646936176702070, 21.00000000000000000, 15.00000000000000000 ) ) ;
#89425=ORIENTED_EDGE ( 'NONE', *, *, #41918, .F. ) ;
#89426=CARTESIAN_POINT ( 'NONE',  ( 205.4738562182569694, 293.9636489450776367, -54.00000000000000000 ) ) ;
#89443=CARTESIAN_POINT ( 'NONE',  ( 209.6287663260175975, 29.00782453271232697, 12.00000000000000000 ) ) ;
#89445=CIRCLE ( 'NONE', #30539, 25.00000000000001066 ) ;
#89448=AXIS2_PLACEMENT_3D ( 'NONE', #58364, #87662, #37028 ) ;
#89449=CARTESIAN_POINT ( 'NONE',  ( 195.7060440449982650, 26.13302583088762532, 14.67646719788673160 ) ) ;
#89457=ORIENTED_EDGE ( 'NONE', *, *, #66023, .F. ) ;
#89466=ORIENTED_EDGE ( 'NONE', *, *, #25669, .T. ) ;
#89472=CARTESIAN_POINT ( 'NONE',  ( 199.2172143179937223, 26.36928053068234590, 9.271110512036644380 ) ) ;
#89476=EDGE_CURVE ( 'NONE', #5341, #68064, #31054, .T. ) ;
#89494=CARTESIAN_POINT ( 'NONE',  ( 209.3679137592659742, 36.51444217272602089, 14.69807323122302023 ) ) ;
#89504=CARTESIAN_POINT ( 'NONE',  ( 207.4724402404594343, 29.73442829110639352, 14.90057469441957672 ) ) ;
#89506=CARTESIAN_POINT ( 'NONE',  ( 154.7659666677267580, 20.47222690886501795, 12.53936336329526036 ) ) ;
#89510=AXIS2_PLACEMENT_3D ( 'NONE', #18288, #25387, #40044 ) ;
#89514=VECTOR ( 'NONE', #26310, 1000.000000000000000 ) ;
#89516=CARTESIAN_POINT ( 'NONE',  ( 160.5350683151633291, 275.5000000000000568, 24.72542485937379197 ) ) ;
#89517=AXIS2_PLACEMENT_3D ( 'NONE', #6778, #64570, #50784 ) ;
#89519=DIRECTION ( 'NONE',  ( 0.000000000000000000, 0.000000000000000000, 1.000000000000000000 ) ) ;
#89522=DIRECTION ( 'NONE',  ( -0.000000000000000000, -0.000000000000000000, 1.000000000000000000 ) ) ;
#89523=CARTESIAN_POINT ( 'NONE',  ( 209.9972545312790544, 27.55378999303205845, 9.000000000000001776 ) ) ;
#89548=DIRECTION ( 'NONE',  ( -1.000000000000000000, 0.000000000000000000, 0.000000000000000000 ) ) ;
#89550=CARTESIAN_POINT ( 'NONE',  ( 175.2296996224750103, 249.5000000000000568, 0.000000000000000000 ) ) ;
#89565=ORIENTED_EDGE ( 'NONE', *, *, #51587, .F. ) ;
#89572=EDGE_CURVE ( 'NONE', #68312, #86758, #19419, .T. ) ;
#89577=ORIENTED_EDGE ( 'NONE', *, *, #68389, .F. ) ;
#89578=CIRCLE ( 'NONE', #74529, 9.550761578869391144 ) ;
#89590=VECTOR ( 'NONE', #12677, 1000.000000000000000 ) ;
#89596=EDGE_LOOP ( 'NONE', ( #30440, #69231, #7757, #43157, #8678, #60952 ) ) ;
#89597=CARTESIAN_POINT ( 'NONE',  ( 156.8097460173007391, 17.78059845260462879, 7.900495735314976287 ) ) ;
#89600=EDGE_CURVE ( 'NONE', #19714, #70200, #18949, .T. ) ;
#89602=ORIENTED_EDGE ( 'NONE', *, *, #87556, .T. ) ;
#89616=VECTOR ( 'NONE', #41113, 1000.000000000000000 ) ;
#89618=AXIS2_PLACEMENT_3D ( 'NONE', #41694, #82910, #4322 ) ;
#89619=CARTESIAN_POINT ( 'NONE',  ( 199.0061125298537377, 275.5000000000000568, -7.725424859374024678 ) ) ;
#89624=DIRECTION ( 'NONE',  ( -0.9693563597868445347, -0.2456588035076248955, 4.725301599749410243E-16 ) ) ;
#89628=DIRECTION ( 'NONE',  ( 0.000000000000000000, 1.000000000000000000, 0.000000000000000000 ) ) ;
#89630=CARTESIAN_POINT ( 'NONE',  ( 159.4851178187817879, 15.24064981607345892, -10.00000000000000178 ) ) ;
#89632=DIRECTION ( 'NONE',  ( -0.000000000000000000, -0.000000000000000000, -1.000000000000000000 ) ) ;
#89645=AXIS2_PLACEMENT_3D ( 'NONE', #81148, #36668, #51791 ) ;
#89650=DIRECTION ( 'NONE',  ( 0.000000000000000000, 1.000000000000000000, -0.000000000000000000 ) ) ;
#89654=CARTESIAN_POINT ( 'NONE',  ( 198.0449670149796475, 67.45552974974890503, 11.11895152694587274 ) ) ;
#89658=CIRCLE ( 'NONE', #56458, 24.50000000000000000 ) ;
#89669=CIRCLE ( 'NONE', #66993, 3.000000000000004885 ) ;
#89671=EDGE_CURVE ( 'NONE', #2063, #88883, #68832, .T. ) ;
#89676=CIRCLE ( 'NONE', #3524, 24.00000000000000355 ) ;
#89686=CIRCLE ( 'NONE', #35309, 4.025000000000000355 ) ;
#89690=ORIENTED_EDGE ( 'NONE', *, *, #31275, .T. ) ;
#89706=EDGE_LOOP ( 'NONE', ( #70069, #31400, #14060, #66514 ) ) ;
#89714=ADVANCED_FACE ( 'NONE', ( #4149 ), #75183, .T. ) ;
#89717=CIRCLE ( 'NONE', #82163, 7.910944475430059519 ) ;
#89723=VECTOR ( 'NONE', #27252, 1000.000000000000000 ) ;
#89728=CARTESIAN_POINT ( 'NONE',  ( 197.2550338912112409, 24.42483738579397823, 11.92230277053072562 ) ) ;
#89738=DIRECTION ( 'NONE',  ( -0.9531768234071978929, 0.3024135303179465439, -0.000000000000000000 ) ) ;
#89741=AXIS2_PLACEMENT_3D ( 'NONE', #47367, #40259, #73273 ) ;
#89745=CARTESIAN_POINT ( 'NONE',  ( 196.6005855419778641, 70.32660332368789113, 11.15032073793429568 ) ) ;
#89754=CARTESIAN_POINT ( 'NONE',  ( 202.8019728163925492, 61.40723988820079171, 7.000000000000000000 ) ) ;
#89759=DIRECTION ( 'NONE',  ( -0.2971780658744820891, 0.9548220761812652446, 0.000000000000000000 ) ) ;
#89787=ORIENTED_EDGE ( 'NONE', *, *, #80919, .T. ) ;
#89788=CARTESIAN_POINT ( 'NONE',  ( 200.2349812190172713, 66.43136063442170780, 7.741079165001067963 ) ) ;
#89791=DIRECTION ( 'NONE',  ( 0.5370370370370374236, 8.780046114482780452E-15, -0.8435586647355830525 ) ) ;
#89799=CIRCLE ( 'NONE', #80761, 1.000000000000000888 ) ;
#89803=ORIENTED_EDGE ( 'NONE', *, *, #78924, .F. ) ;
#89821=ORIENTED_EDGE ( 'NONE', *, *, #6894, .T. ) ;
#89829=TOROIDAL_SURFACE ( 'NONE', #2184, 4.499999999999986677, 0.5000000000000000000 ) ;
#89836=DIRECTION ( 'NONE',  ( 0.000000000000000000, 1.000000000000000000, 0.000000000000000000 ) ) ;
#89839=CARTESIAN_POINT ( 'NONE',  ( 193.9646936176697523, 21.00000000000000000, 15.00000000000057909 ) ) ;
#89848=CARTESIAN_POINT ( 'NONE',  ( 196.0143093133015384, 42.36571313990103249, 11.99999999999998757 ) ) ;
#89850=EDGE_CURVE ( 'NONE', #10831, #6353, #86992, .T. ) ;
#89851=ORIENTED_EDGE ( 'NONE', *, *, #29441, .T. ) ;
#89852=CARTESIAN_POINT ( 'NONE',  ( 201.2104617360081704, 15.00000000000000533, 10.00000000000000178 ) ) ;
#89868=CARTESIAN_POINT ( 'NONE',  ( 154.3120505024585327, 19.86534941647301977, -13.70129228612095673 ) ) ;
#89880=CARTESIAN_POINT ( 'NONE',  ( 139.6539576904058606, 275.0000000000000568, -10.49999999999999822 ) ) ;
#89882=CARTESIAN_POINT ( 'NONE',  ( 196.0143093133015384, 20.19615242270663913, 11.99999999999998757 ) ) ;
#89888=ADVANCED_FACE ( 'NONE', ( #89355 ), #24511, .F. ) ;
#89893=CARTESIAN_POINT ( 'NONE',  ( 196.3496553477289979, 250.5000000000000568, -12.41762739670150850 ) ) ;
#89903=VERTEX_POINT ( 'NONE', #57613 ) ;
#89904=DIRECTION ( 'NONE',  ( 0.000000000000000000, 1.000000000000000000, 0.000000000000000000 ) ) ;
#89910=ADVANCED_FACE ( 'NONE', ( #34896 ), #41021, .T. ) ;
#89920=DIRECTION ( 'NONE',  ( 0.000000000000000000, 1.000000000000000000, 0.000000000000000000 ) ) ;
#89922=CARTESIAN_POINT ( 'NONE',  ( 196.5878321470269157, 70.38283977259966662, 11.16596772118615988 ) ) ;
#89926=CARTESIAN_POINT ( 'NONE',  ( 165.2494399300530290, 8.542400036368780647, -9.000000000000001776 ) ) ;
#89935=ORIENTED_EDGE ( 'NONE', *, *, #71254, .T. ) ;
#89939=VECTOR ( 'NONE', #18002, 1000.000000000000000 ) ;
#89944=ORIENTED_EDGE ( 'NONE', *, *, #83917, .F. ) ;
#89945=VERTEX_POINT ( 'NONE', #5087 ) ;
#89946=EDGE_CURVE ( 'NONE', #91341, #37341, #20225, .T. ) ;
#89952=CARTESIAN_POINT ( 'NONE',  ( 200.5559520117673458, 215.0000000000000568, -2.971689740512053035 ) ) ;
#89964=VERTEX_POINT ( 'NONE', #57161 ) ;
#89965=DIRECTION ( 'NONE',  ( 0.000000000000000000, 0.000000000000000000, 1.000000000000000000 ) ) ;
#89973=FACE_OUTER_BOUND ( 'NONE', #57291, .T. ) ;
#89992=EDGE_CURVE ( 'NONE', #14615, #52785, #78914, .T. ) ;
#89993=CARTESIAN_POINT ( 'NONE',  ( 153.7504314680575987, 128.6410103095127226, -12.94315874461255689 ) ) ;
#89995=CARTESIAN_POINT ( 'NONE',  ( 197.4657836131030706, 215.0000000000000568, -12.48225014817974987 ) ) ;
#89997=CARTESIAN_POINT ( 'NONE',  ( 197.9510320457498551, 42.14527911255801484, 11.14415317764935587 ) ) ;
#89998=DIRECTION ( 'NONE',  ( 0.000000000000000000, -0.000000000000000000, 1.000000000000000000 ) ) ;
#90008=CARTESIAN_POINT ( 'NONE',  ( 208.3418117619747818, 38.42745601219718310, 12.00000000000000000 ) ) ;
#90011=LINE ( 'NONE', #51701, #3467 ) ;
#90014=EDGE_CURVE ( 'NONE', #60939, #87677, #56701, .T. ) ;
#90017=CIRCLE ( 'NONE', #74986, 0.5000000000000004441 ) ;
#90024=CARTESIAN_POINT ( 'NONE',  ( 156.5008572374906066, 15.54442400203491026, 9.984260581292296877 ) ) ;
#90026=ADVANCED_FACE ( 'NONE', ( #50021 ), #49565, .T. ) ;
#90028=CARTESIAN_POINT ( 'NONE',  ( 140.6539576904058606, 250.0000000000000568, -10.49999999999999822 ) ) ;
#90042=VERTEX_POINT ( 'NONE', #41977 ) ;
#90044=EDGE_LOOP ( 'NONE', ( #89069, #17389, #66652, #12307 ) ) ;
#90054=VERTEX_POINT ( 'NONE', #6021 ) ;
#90061=FACE_OUTER_BOUND ( 'NONE', #26744, .T. ) ;
#90062=EDGE_CURVE ( 'NONE', #56456, #14859, #14061, .T. ) ;
#90067=ORIENTED_EDGE ( 'NONE', *, *, #10809, .T. ) ;
#90074=ORIENTED_EDGE ( 'NONE', *, *, #73934, .T. ) ;
#90086=DIRECTION ( 'NONE',  ( 0.000000000000000000, 0.000000000000000000, 1.000000000000000000 ) ) ;
#90097=DIRECTION ( 'NONE',  ( 0.000000000000000000, -1.000000000000000000, 0.000000000000000000 ) ) ;
#90102=CARTESIAN_POINT ( 'NONE',  ( 208.8931598777758438, 1.060642095945600216, 7.489249145872055813 ) ) ;
#90103=DIRECTION ( 'NONE',  ( -1.000000000000000000, 0.000000000000000000, 0.000000000000000000 ) ) ;
#90106=DIRECTION ( 'NONE',  ( 0.000000000000000000, 0.000000000000000000, 1.000000000000000000 ) ) ;
#90109=CARTESIAN_POINT ( 'NONE',  ( 199.7648473163311849, 63.23516263141960536, 10.15923027032019021 ) ) ;
#90111=CARTESIAN_POINT ( 'NONE',  ( 207.1360844159087549, 30.54655824920636675, 14.49999999999999822 ) ) ;
#90122=EDGE_CURVE ( 'NONE', #13010, #48224, #27808, .T. ) ;
#90128=PLANE ( 'NONE',  #65125 ) ;
#90132=DIRECTION ( 'NONE',  ( -0.000000000000000000, -0.000000000000000000, -1.000000000000000000 ) ) ;
#90148=B_SPLINE_CURVE_WITH_KNOTS ( 'NONE', 3,
 ( #20362, #50639, #444, #6152, #28401, #27944 ),
 .UNSPECIFIED., .F., .F.,
 ( 4, 2, 4 ),
 ( 0.000000000000000000, 0.0004262108901887199383, 0.0008524217803774398767 ),
 .UNSPECIFIED. ) ;
#90150=CARTESIAN_POINT ( 'NONE',  ( 152.4536156746142410, 275.5000000000000568, 14.50000000000000000 ) ) ;
#90163=ORIENTED_EDGE ( 'NONE', *, *, #29603, .F. ) ;
#90182=ORIENTED_EDGE ( 'NONE', *, *, #92757, .F. ) ;
#90193=CARTESIAN_POINT ( 'NONE',  ( 151.4851178187871312, 20.00000000000000000, -3.492110388858667314 ) ) ;
#90198=DIRECTION ( 'NONE',  ( 0.000000000000000000, 0.000000000000000000, 1.000000000000000000 ) ) ;
#90206=CARTESIAN_POINT ( 'NONE',  ( 153.6987871352710613, 19.48326534539920019, -11.45812909362551757 ) ) ;
#90224=DIRECTION ( 'NONE',  ( -0.000000000000000000, -1.000000000000000000, -9.656854691831248164E-17 ) ) ;
#90238=CYLINDRICAL_SURFACE ( 'NONE', #89510, 0.5000000000000004441 ) ;
#90252=ORIENTED_EDGE ( 'NONE', *, *, #73796, .T. ) ;
#90255=CYLINDRICAL_SURFACE ( 'NONE', #27822, 0.5000000000000004441 ) ;
#90266=VERTEX_POINT ( 'NONE', #1695 ) ;
#90280=VERTEX_POINT ( 'NONE', #22090 ) ;
#90294=DIRECTION ( 'NONE',  ( -0.3994899938747922263, 0.000000000000000000, 0.9167375550253837879 ) ) ;
#90297=CARTESIAN_POINT ( 'NONE',  ( 189.9243309297870610, 275.5000000000000568, 24.72542485937349710 ) ) ;
#90298=CARTESIAN_POINT ( 'NONE',  ( 197.8536156918358131, 70.38469146216345962, 8.282373351508748982 ) ) ;
#90308=CARTESIAN_POINT ( 'NONE',  ( 198.8856906601484980, 17.32477107587147458, 10.54429824094339097 ) ) ;
#90310=EDGE_CURVE ( 'NONE', #10071, #4825, #68901, .T. ) ;
#90324=CARTESIAN_POINT ( 'NONE',  ( 196.6930115205277616, 40.98292740024594849, 12.61309341605360856 ) ) ;
#90338=DIRECTION ( 'NONE',  ( 0.000000000000000000, 0.000000000000000000, 1.000000000000000000 ) ) ;
#90344=DIRECTION ( 'NONE',  ( -0.000000000000000000, -1.000000000000000000, -0.000000000000000000 ) ) ;
#90356=CARTESIAN_POINT ( 'NONE',  ( 197.2116943569230330, 275.0000000000000568, -12.92446933126074882 ) ) ;
#90358=DIRECTION ( 'NONE',  ( -1.000000000000000000, 0.000000000000000000, 0.000000000000000000 ) ) ;
#90368=ORIENTED_EDGE ( 'NONE', *, *, #26658, .F. ) ;
#90373=EDGE_CURVE ( 'NONE', #20997, #71446, #44685, .T. ) ;
#90379=CARTESIAN_POINT ( 'NONE',  ( 200.1145890159574492, 64.93834475843401322, -5.212391550061756362 ) ) ;
#90380=CARTESIAN_POINT ( 'NONE',  ( 195.8444066023239714, 25.85623389517961002, 14.49918517833957132 ) ) ;
#90395=ORIENTED_EDGE ( 'NONE', *, *, #51306, .F. ) ;
#90397=FACE_OUTER_BOUND ( 'NONE', #15109, .T. ) ;
#90402=CARTESIAN_POINT ( 'NONE',  ( 201.2104617360081704, 25.32700003806617772, 9.000000000000000000 ) ) ;
#90421=DIRECTION ( 'NONE',  ( -0.000000000000000000, 1.000000000000000000, 0.000000000000000000 ) ) ;
#90425=ADVANCED_FACE ( 'NONE', ( #50960 ), #30120, .T. ) ;
#90435=DIRECTION ( 'NONE',  ( 0.000000000000000000, -1.000000000000000000, 0.000000000000000000 ) ) ;
#90443=FACE_OUTER_BOUND ( 'NONE', #40658, .T. ) ;
#90445=CARTESIAN_POINT ( 'NONE',  ( 150.6539576904058606, 293.9636489450775230, -9.103929867429224387 ) ) ;
#90448=CARTESIAN_POINT ( 'NONE',  ( 140.6539576904058606, 250.0000000000000568, -12.50000000000000000 ) ) ;
#90457=AXIS2_PLACEMENT_3D ( 'NONE', #980, #58745, #87588 ) ;
#90463=DIRECTION ( 'NONE',  ( 0.000000000000000000, -1.000000000000000000, 0.000000000000000000 ) ) ;
#90474=CARTESIAN_POINT ( 'NONE',  ( 208.6208076322478746, 32.98517505407394168, 10.50000000000000000 ) ) ;
#90475=DIRECTION ( 'NONE',  ( 0.000000000000000000, 1.000000000000000000, 0.000000000000000000 ) ) ;
#90490=ORIENTED_EDGE ( 'NONE', *, *, #26879, .T. ) ;
#90495=CARTESIAN_POINT ( 'NONE',  ( 196.1243318874861927, 19.88069242108673507, -13.74009414728758216 ) ) ;
#90519=FACE_OUTER_BOUND ( 'NONE', #83632, .T. ) ;
#90525=CIRCLE ( 'NONE', #87504, 0.5000000000000004441 ) ;
#90537=EDGE_CURVE ( 'NONE', #43024, #25984, #93087, .T. ) ;
#90539=ADVANCED_FACE ( 'NONE', ( #79843 ), #22064, .T. ) ;
#90541=( BOUNDED_CURVE ( )  B_SPLINE_CURVE ( 3, ( #12804, #62038, #18954, #70085 ),
 .UNSPECIFIED., .F., .F. ) 
 B_SPLINE_CURVE_WITH_KNOTS ( ( 4, 4 ),
 ( 3.141592653589793116, 4.289818581638156658 ),
 .UNSPECIFIED. ) 
 CURVE ( )  GEOMETRIC_REPRESENTATION_ITEM ( )  RATIONAL_B_SPLINE_CURVE ( ( 1.000000000000000000, 0.8931162488197521565, 0.8931162488197521565, 1.000000000000000000 ) ) 
 REPRESENTATION_ITEM ( '' )  );
#90544=CARTESIAN_POINT ( 'NONE',  ( 205.7381008070597943, 1.000000000000000000, -6.999999999999991118 ) ) ;
#90549=DIRECTION ( 'NONE',  ( 0.000000000000000000, 0.000000000000000000, 1.000000000000000000 ) ) ;
#90552=CARTESIAN_POINT ( 'NONE',  ( 175.2296996224750103, 133.0000000000000000, 24.00000000000001066 ) ) ;
#90557=CARTESIAN_POINT ( 'NONE',  ( 216.5288609127277084, 293.9636489450776935, -40.00000000000000711 ) ) ;
#90560=CARTESIAN_POINT ( 'NONE',  ( 155.4148940283161835, 19.61091623264263362, -11.07022379048152239 ) ) ;
#90572=CARTESIAN_POINT ( 'NONE',  ( 175.2296996224750103, 20.00000000000000000, 0.000000000000000000 ) ) ;
#90574=ORIENTED_EDGE ( 'NONE', *, *, #3741, .T. ) ;
#90576=CARTESIAN_POINT ( 'NONE',  ( 196.9830544186642953, 72.65363667333228648, 12.32798201617853984 ) ) ;
#90590=AXIS2_PLACEMENT_3D ( 'NONE', #93061, #91164, #57105 ) ;
#90605=ORIENTED_EDGE ( 'NONE', *, *, #7600, .T. ) ;
#90608=ORIENTED_EDGE ( 'NONE', *, *, #21310, .T. ) ;
#90630=VERTEX_POINT ( 'NONE', #59474 ) ;
#90633=ORIENTED_EDGE ( 'NONE', *, *, #53671, .F. ) ;
#90640=PLANE ( 'NONE',  #7884 ) ;
#90645=CARTESIAN_POINT ( 'NONE',  ( 196.8803347170859865, 20.19615242270636557, -12.49999999999999289 ) ) ;
#90660=CARTESIAN_POINT ( 'NONE',  ( 198.6806486734898272, 66.92004278903957015, 8.362876768746247080 ) ) ;
#90674=CARTESIAN_POINT ( 'NONE',  ( 151.4851178187871312, 21.00000000000000000, -3.492110388858666870 ) ) ;
#90682=CARTESIAN_POINT ( 'NONE',  ( 164.2231345125756263, 264.6571197653884155, -7.500000000000000000 ) ) ;
#90683=DIRECTION ( 'NONE',  ( 1.110223024625155531E-13, 0.000000000000000000, 1.000000000000000000 ) ) ;
#90699=ORIENTED_EDGE ( 'NONE', *, *, #32642, .T. ) ;
#90700=DIRECTION ( 'NONE',  ( 1.000000000000000000, 0.000000000000000000, 0.000000000000000000 ) ) ;
#90702=DIRECTION ( 'NONE',  ( 0.000000000000000000, 0.000000000000000000, 1.000000000000000000 ) ) ;
#90713=ORIENTED_EDGE ( 'NONE', *, *, #75906, .F. ) ;
#90722=CIRCLE ( 'NONE', #43907, 25.00000000000000355 ) ;
#90731=ORIENTED_EDGE ( 'NONE', *, *, #77442, .F. ) ;
#90736=CIRCLE ( 'NONE', #6170, 2.000000000000000000 ) ;
#90748=EDGE_CURVE ( 'NONE', #9431, #4576, #90017, .T. ) ;
#90757=DIRECTION ( 'NONE',  ( 1.000000000000000000, 0.000000000000000000, 0.000000000000000000 ) ) ;
#90761=ORIENTED_EDGE ( 'NONE', *, *, #49105, .T. ) ;
#90763=CARTESIAN_POINT ( 'NONE',  ( 201.2104617360081704, 15.00000000000000711, 10.00000000000000178 ) ) ;
#90775=EDGE_CURVE ( 'NONE', #87609, #1443, #15921, .T. ) ;
#90778=CARTESIAN_POINT ( 'NONE',  ( 196.7806748523260012, 275.0000000000000568, -12.67104836398113044 ) ) ;
#90779=CARTESIAN_POINT ( 'NONE',  ( 156.4851178187871312, 16.95599219719193229, -7.000000000000000000 ) ) ;
#90793=VECTOR ( 'NONE', #41827, 1000.000000000000000 ) ;
#90803=CARTESIAN_POINT ( 'NONE',  ( 196.6777378159611089, 42.34889665583091301, 12.85090812620430789 ) ) ;
#90814=CARTESIAN_POINT ( 'NONE',  ( 200.3359402460285139, 61.72811464988816255, 8.999999999999998224 ) ) ;
#90828=DIRECTION ( 'NONE',  ( 0.000000000000000000, 0.000000000000000000, -1.000000000000000000 ) ) ;
#90829=ADVANCED_FACE ( 'NONE', ( #37665 ), #52350, .T. ) ;
#90835=CARTESIAN_POINT ( 'NONE',  ( 194.2870706637141325, 250.0000000000000568, 14.58823529411763431 ) ) ;
#90836=CARTESIAN_POINT ( 'NONE',  ( 195.2729366661233144, 26.72345838548328345, 14.94480962496910159 ) ) ;
#90845=ORIENTED_EDGE ( 'NONE', *, *, #60850, .F. ) ;
#90853=EDGE_CURVE ( 'NONE', #443, #31059, #45223, .T. ) ;
#90855=ORIENTED_EDGE ( 'NONE', *, *, #89476, .F. ) ;
#90861=CARTESIAN_POINT ( 'NONE',  ( 165.4284657918965991, 2.965303559109565334, -9.000000000000001776 ) ) ;
#90871=ORIENTED_EDGE ( 'NONE', *, *, #25372, .F. ) ;
#90872=CARTESIAN_POINT ( 'NONE',  ( 140.6539576904058606, 250.5000000000000568, -12.00000000000000000 ) ) ;
#90876=EDGE_CURVE ( 'NONE', #35594, #38261, #67421, .T. ) ;
#90895=CARTESIAN_POINT ( 'NONE',  ( 208.4306832106271088, -74.55766379199613425, 0.000000000000000000 ) ) ;
#90903=CARTESIAN_POINT ( 'NONE',  ( 199.6150009768959990, 276.0000000000000568, -2.367926910627516257 ) ) ;
#90905=CARTESIAN_POINT ( 'NONE',  ( 201.9220344434848755, 287.7612796304733251, -5.053264882194825169 ) ) ;
#90907=DIRECTION ( 'NONE',  ( 0.000000000000000000, 0.000000000000000000, 1.000000000000000000 ) ) ;
#90919=ORIENTED_EDGE ( 'NONE', *, *, #84689, .T. ) ;
#90923=DIRECTION ( 'NONE',  ( 0.000000000000000000, 0.000000000000000000, -1.000000000000000000 ) ) ;
#90927=AXIS2_PLACEMENT_3D ( 'NONE', #31102, #81269, #15026 ) ;
#90938=B_SPLINE_CURVE_WITH_KNOTS ( 'NONE', 3,
 ( #80227, #52724, #67434, #1616, #16756, #1160, #36671, #30043 ),
 .UNSPECIFIED., .F., .F.,
 ( 4, 2, 2, 4 ),
 ( 0.000000000000000000, 0.0008414166960586483236, 0.001682833392117296647, 0.003365666784234650107 ),
 .UNSPECIFIED. ) ;
#90952=VERTEX_POINT ( 'NONE', #38124 ) ;
#90959=CARTESIAN_POINT ( 'NONE',  ( 0.000000000000000000, 0.000000000000000000, 0.000000000000000000 ) ) ;
#90976=VERTEX_POINT ( 'NONE', #31060 ) ;
#90983=ORIENTED_EDGE ( 'NONE', *, *, #69967, .T. ) ;
#90988=EDGE_LOOP ( 'NONE', ( #56296, #85674, #45945, #2147 ) ) ;
#90993=CIRCLE ( 'NONE', #41046, 0.5000000000000068834 ) ;
#90996=CARTESIAN_POINT ( 'NONE',  ( 221.8344101925596306, 0.000000000000000000, 7.000000000000000000 ) ) ;
#90998=CIRCLE ( 'NONE', #72856, 0.5000000000000004441 ) ;
#91005=CIRCLE ( 'NONE', #80485, 4.003189038634634045 ) ;
#91019=VERTEX_POINT ( 'NONE', #45691 ) ;
#91020=CARTESIAN_POINT ( 'NONE',  ( 201.2849759805918382, 65.05171340438522520, 7.254661561168179951 ) ) ;
#91034=EDGE_LOOP ( 'NONE', ( #71937, #27824, #66460, #82524 ) ) ;
#91039=ORIENTED_EDGE ( 'NONE', *, *, #2612, .F. ) ;
#91041=CARTESIAN_POINT ( 'NONE',  ( 183.0442525570908288, 264.6571197653884155, 7.500000000000000000 ) ) ;
#91056=TOROIDAL_SURFACE ( 'NONE', #36623, 5.603083949679977138, 0.5000000000000000000 ) ;
#91063=EDGE_CURVE ( 'NONE', #70513, #87609, #45206, .T. ) ;
#91066=CARTESIAN_POINT ( 'NONE',  ( 200.4816938276917995, 61.72811464988816965, 9.999999999999998224 ) ) ;
#91068=EDGE_CURVE ( 'NONE', #54877, #26035, #41640, .T. ) ;
#91071=CIRCLE ( 'NONE', #77529, 4.999999999999986677 ) ;
#91096=( BOUNDED_SURFACE ( )  B_SPLINE_SURFACE ( 3, 2, ( 
 ( #72588, #7710, #87239 ),
 ( #22386, #51258, #41938 ),
 ( #84557, #37064, #29964 ),
 ( #70850, #92131, #12618 ),
 ( #41464, #5523, #34393 ),
 ( #63300, #27286, #45068 ),
 ( #38897, #39821, #53111 ),
 ( #1535, #61187, #30420 ),
 ( #25177, #53598, #73968 ),
 ( #82470, #30899, #16670 ),
 ( #18075, #32281, #37962 ),
 ( #2005, #90024, #17617 ),
 ( #59790, #88631, #45525 ),
 ( #81990, #66869, #54051 ),
 ( #59311, #9082, #74427 ),
 ( #31815, #23778, #31359 ) ),
 .UNSPECIFIED., .F., .F., .F. ) 
 B_SPLINE_SURFACE_WITH_KNOTS ( ( 4, 2, 2, 2, 2, 2, 2, 4 ),
 ( 3, 3 ),
 ( 5.128070023563283009, 5.416848844467358148, 5.561238254919396162, 5.705627665371434176, 5.850017075823472190, 5.994406486275510204, 6.138795896727548218, 6.283185307179586232 ),
 ( 0.000000000000000000, 1.000000000000000000 ),
 .UNSPECIFIED. ) 
 GEOMETRIC_REPRESENTATION_ITEM ( )  RATIONAL_B_SPLINE_SURFACE ( (
 ( 1.000000000000000000, 0.9583671019092242505, 1.000000000000000000),
 ( 1.000000000000000000, 0.9398658125638100769, 1.000000000000000000),
 ( 1.000000000000000000, 0.9157002655843566874, 1.000000000000000000),
 ( 1.000000000000000000, 0.8756259400453313413, 1.000000000000000000),
 ( 1.000000000000000000, 0.8616433317033089789, 1.000000000000000000),
 ( 1.000000000000000000, 0.8334785261034494130, 1.000000000000000000),
 ( 1.000000000000000000, 0.8192978668688222221, 1.000000000000000000),
 ( 1.000000000000000000, 0.7919708659745230417, 1.000000000000000000),
 ( 1.000000000000000000, 0.7788285231915303974, 1.000000000000000000),
 ( 1.000000000000000000, 0.7549177526733705790, 1.000000000000000000),
 ( 1.000000000000000000, 0.7441566529437987354, 1.000000000000000000),
 ( 1.000000000000000000, 0.7262859251462959742, 1.000000000000000000),
 ( 1.000000000000000000, 0.7191857644035468677, 1.000000000000000000),
 ( 1.000000000000000000, 0.7095926089624788879, 1.000000000000000000),
 ( 1.000000000000000000, 0.7070960980132534601, 1.000000000000000000),
 ( 1.000000000000000000, 0.7071067811865473507, 1.000000000000000000) ) ) 
 REPRESENTATION_ITEM ( '' )  SURFACE ( )  );
#91098=AXIS2_PLACEMENT_3D ( 'NONE', #52178, #81060, #24700 ) ;
#91102=ORIENTED_EDGE ( 'NONE', *, *, #9083, .T. ) ;
#91105=ORIENTED_EDGE ( 'NONE', *, *, #34233, .T. ) ;
#91117=DIRECTION ( 'NONE',  ( -5.551115123125777653E-14, 0.000000000000000000, 1.000000000000000000 ) ) ;
#91118=AXIS2_PLACEMENT_3D ( 'NONE', #12820, #41660, #34578 ) ;
#91126=LINE ( 'NONE', #76959, #62450 ) ;
#91133=CIRCLE ( 'NONE', #53378, 2.000000000000001776 ) ;
#91134=AXIS2_PLACEMENT_3D ( 'NONE', #16010, #36851, #81779 ) ;
#91137=CIRCLE ( 'NONE', #60980, 1.000000000000000888 ) ;
#91143=CARTESIAN_POINT ( 'NONE',  ( 195.6782526186922269, 40.73232731989658362, 14.69414600581795050 ) ) ;
#91144=CARTESIAN_POINT ( 'NONE',  ( 197.8477145984406889, 64.61450673763175701, 7.741079165001056417 ) ) ;
#91148=CIRCLE ( 'NONE', #86645, 0.9999999999999998890 ) ;
#91150=CARTESIAN_POINT ( 'NONE',  ( 154.1415209985679269, 20.37991841447901820, -11.45812909362559040 ) ) ;
#91155=AXIS2_PLACEMENT_3D ( 'NONE', #37710, #51455, #23980 ) ;
#91164=DIRECTION ( 'NONE',  ( 0.9764705882352960886, 0.000000000000000000, -0.2156506209390900708 ) ) ;
#91168=CIRCLE ( 'NONE', #14098, 23.00000000000000711 ) ;
#91180=ORIENTED_EDGE ( 'NONE', *, *, #62216, .F. ) ;
#91186=ADVANCED_FACE ( 'NONE', ( #49196 ), #27909, .T. ) ;
#91194=ORIENTED_EDGE ( 'NONE', *, *, #78924, .T. ) ;
#91203=AXIS2_PLACEMENT_3D ( 'NONE', #40361, #33286, #33760 ) ;
#91206=CIRCLE ( 'NONE', #59480, 2.500000000000002220 ) ;
#91211=ORIENTED_EDGE ( 'NONE', *, *, #19481, .F. ) ;
#91217=AXIS2_PLACEMENT_3D ( 'NONE', #74384, #2891, #60668 ) ;
#91230=CARTESIAN_POINT ( 'NONE',  ( 208.6208076322478746, 32.98517505407394168, 15.00000000000000000 ) ) ;
#91239=CARTESIAN_POINT ( 'NONE',  ( 183.0442525570908288, 300.2961574867697436, -7.500000000000000000 ) ) ;
#91241=CARTESIAN_POINT ( 'NONE',  ( 194.3451372756567537, 40.15325844710437053, 14.51211662731439844 ) ) ;
#91243=CIRCLE ( 'NONE', #50382, 1.500000000000001332 ) ;
#91244=ORIENTED_EDGE ( 'NONE', *, *, #90537, .T. ) ;
#91245=CARTESIAN_POINT ( 'NONE',  ( 197.9834613664959591, 18.87240044341487533, 11.15593255764673408 ) ) ;
#91259=CYLINDRICAL_SURFACE ( 'NONE', #6660, 5.000000000000000888 ) ;
#91260=CARTESIAN_POINT ( 'NONE',  ( 155.4526335419795373, 18.61728136335800343, -8.651974842892215634 ) ) ;
#91274=CARTESIAN_POINT ( 'NONE',  ( 189.9243309297870610, 275.0000000000000568, 15.22542485937351664 ) ) ;
#91277=CIRCLE ( 'NONE', #50480, 0.5000000000000009992 ) ;
#91283=AXIS2_PLACEMENT_3D ( 'NONE', #84284, #54945, #48298 ) ;
#91292=AXIS2_PLACEMENT_3D ( 'NONE', #81212, #66110, #2155 ) ;
#91293=ADVANCED_FACE ( 'NONE', ( #70984 ), #19372, .F. ) ;
#91296=ORIENTED_EDGE ( 'NONE', *, *, #4934, .T. ) ;
#91297=CARTESIAN_POINT ( 'NONE',  ( 201.2509219215140206, 65.09645894978946501, -2.617322427804798401 ) ) ;
#91308=CIRCLE ( 'NONE', #50511, 0.4999999999999929501 ) ;
#91310=ORIENTED_EDGE ( 'NONE', *, *, #9906, .T. ) ;
#91321=CYLINDRICAL_SURFACE ( 'NONE', #7989, 4.999999999999990230 ) ;
#91322=CARTESIAN_POINT ( 'NONE',  ( 208.6208076322478746, 32.98517505407394168, 12.09245862095555601 ) ) ;
#91332=VERTEX_POINT ( 'NONE', #92264 ) ;
#91341=VERTEX_POINT ( 'NONE', #64843 ) ;
#91342=B_SPLINE_CURVE_WITH_KNOTS ( 'NONE', 3,
 ( #78962, #51002, #42493, #14579, #93617, #50066, #42020, #64337 ),
 .UNSPECIFIED., .F., .F.,
 ( 4, 2, 2, 4 ),
 ( 0.000000000000000000, 0.001936817825059323562, 0.002905226737588965501, 0.003873635650118607658 ),
 .UNSPECIFIED. ) ;
#91343=AXIS2_PLACEMENT_3D ( 'NONE', #85459, #56605, #28183 ) ;
#91344=CARTESIAN_POINT ( 'NONE',  ( 175.2296996224750103, 134.0000000000000284, 0.000000000000000000 ) ) ;
#91360=ORIENTED_EDGE ( 'NONE', *, *, #26082, .F. ) ;
#91361=DIRECTION ( 'NONE',  ( 0.000000000000000000, 0.000000000000000000, -1.000000000000000000 ) ) ;
#91363=VECTOR ( 'NONE', #36798, 1000.000000000000000 ) ;
#91365=AXIS2_PLACEMENT_3D ( 'NONE', #47908, #76811, #11936 ) ;
#91378=B_SPLINE_CURVE_WITH_KNOTS ( 'NONE', 3,
 ( #66522, #38069, #1641, #30521, #23429, #88735 ),
 .UNSPECIFIED., .F., .F.,
 ( 4, 2, 4 ),
 ( 0.000000000000000000, 0.0009572278725339521555, 0.001914455745067904311 ),
 .UNSPECIFIED. ) ;
#91387=AXIS2_PLACEMENT_3D ( 'NONE', #34986, #21724, #6115 ) ;
#91389=DIRECTION ( 'NONE',  ( 1.000000000000000000, 0.000000000000000000, 0.000000000000000000 ) ) ;
#91399=CARTESIAN_POINT ( 'NONE',  ( 197.4836817735085219, 42.27872732282707346, 11.66666666666666785 ) ) ;
#91401=CARTESIAN_POINT ( 'NONE',  ( 197.3748232817349049, 275.5000000000000568, -12.45182892472559821 ) ) ;
#91403=DIRECTION ( 'NONE',  ( 0.000000000000000000, -1.000000000000000000, 0.000000000000000000 ) ) ;
#91412=EDGE_CURVE ( 'NONE', #27913, #14834, #77140, .T. ) ;
#91415=LINE ( 'NONE', #75356, #63496 ) ;
#91418=CARTESIAN_POINT ( 'NONE',  ( 207.2842799582832356, 30.47689859374760957, 11.99999999999999822 ) ) ;
#91430=AXIS2_PLACEMENT_3D ( 'NONE', #46396, #17066, #25559 ) ;
#91432=EDGE_CURVE ( 'NONE', #51603, #72522, #16043, .T. ) ;
#91433=CARTESIAN_POINT ( 'NONE',  ( 151.4851178187871312, 20.00000000000000000, -3.492110388858666870 ) ) ;
#91480=VERTEX_POINT ( 'NONE', #20786 ) ;
#91481=CARTESIAN_POINT ( 'NONE',  ( 160.6539576904058606, 293.9636489450775230, 0.000000000000000000 ) ) ;
#91502=ADVANCED_FACE ( 'NONE', ( #6591 ), #6116, .T. ) ;
#91505=CARTESIAN_POINT ( 'NONE',  ( 209.6287663260175975, 29.00782453271232697, 10.50000000000000000 ) ) ;
#91513=ORIENTED_EDGE ( 'NONE', *, *, #250, .T. ) ;
#91519=CARTESIAN_POINT ( 'NONE',  ( 157.7670607448636702, 18.75975317436435574, -10.28854280544447697 ) ) ;
#91529=ORIENTED_EDGE ( 'NONE', *, *, #93048, .T. ) ;
#91532=DIRECTION ( 'NONE',  ( 0.000000000000000000, 1.000000000000000000, 0.000000000000000000 ) ) ;
#91534=ORIENTED_EDGE ( 'NONE', *, *, #48886, .F. ) ;
#91536=DIRECTION ( 'NONE',  ( 0.000000000000000000, 1.000000000000000000, 0.000000000000000000 ) ) ;
#91551=DIRECTION ( 'NONE',  ( 0.000000000000000000, 0.000000000000000000, 1.000000000000000000 ) ) ;
#91558=CARTESIAN_POINT ( 'NONE',  ( 197.2116943569230330, 250.5000000000000568, -12.42446933126074882 ) ) ;
#91565=EDGE_CURVE ( 'NONE', #36764, #16269, #21726, .T. ) ;
#91567=ORIENTED_EDGE ( 'NONE', *, *, #56930, .F. ) ;
#91595=ORIENTED_EDGE ( 'NONE', *, *, #81578, .F. ) ;
#91597=ORIENTED_EDGE ( 'NONE', *, *, #48446, .T. ) ;
#91604=CARTESIAN_POINT ( 'NONE',  ( 219.8344101925596021, 3.000000000000000000, 9.000000000000001776 ) ) ;
#91617=CARTESIAN_POINT ( 'NONE',  ( 153.8045260737213482, 20.39559083867290568, 12.88430403588788842 ) ) ;
#91623=ADVANCED_FACE ( 'NONE', ( #51502 ), #8457, .T. ) ;
#91624=CARTESIAN_POINT ( 'NONE',  ( 196.8320172978770870, 70.49480016127409954, 10.86682040754346090 ) ) ;
#91628=CARTESIAN_POINT ( 'NONE',  ( 208.1728644033713636, 30.17484991538838912, 14.33122224313838800 ) ) ;
#91631=CARTESIAN_POINT ( 'NONE',  ( 197.7051530045995094, 41.80213891112347113, 12.00000000000000888 ) ) ;
#91636=DIRECTION ( 'NONE',  ( -1.000000000000000000, 0.000000000000000000, 0.000000000000000000 ) ) ;
#91648=DIRECTION ( 'NONE',  ( -0.000000000000000000, -1.000000000000000000, -0.000000000000000000 ) ) ;
#91651=AXIS2_PLACEMENT_3D ( 'NONE', #55263, #26839, #49084 ) ;
#91666=DIRECTION ( 'NONE',  ( -0.000000000000000000, -0.000000000000000000, 1.000000000000000000 ) ) ;
#91675=( BOUNDED_CURVE ( )  B_SPLINE_CURVE ( 3, ( #814, #16862, #51906, #15946 ),
 .UNSPECIFIED., .F., .F. ) 
 B_SPLINE_CURVE_WITH_KNOTS ( ( 4, 4 ),
 ( 4.712388980384689674, 5.553457650952617008 ),
 .UNSPECIFIED. ) 
 CURVE ( )  GEOMETRIC_REPRESENTATION_ITEM ( )  RATIONAL_B_SPLINE_CURVE ( ( 1.000000000000000000, 0.9419139527835183046, 0.9419139527835183046, 1.000000000000000000 ) ) 
 REPRESENTATION_ITEM ( '' )  );
#91679=( BOUNDED_CURVE ( )  B_SPLINE_CURVE ( 3, ( #88256, #59402, #45156, #7793 ),
 .UNSPECIFIED., .F., .F. ) 
 B_SPLINE_CURVE_WITH_KNOTS ( ( 4, 4 ),
 ( 3.665191429188167760, 4.712388980384689674 ),
 .UNSPECIFIED. ) 
 CURVE ( )  GEOMETRIC_REPRESENTATION_ITEM ( )  RATIONAL_B_SPLINE_CURVE ( ( 1.000000000000000000, 0.9106836025229716469, 0.9106836025229716469, 1.000000000000000000 ) ) 
 REPRESENTATION_ITEM ( '' )  );
#91687=CARTESIAN_POINT ( 'NONE',  ( 197.6805213618982009, 68.84011358609819808, 9.477520602874013989 ) ) ;
#91704=ORIENTED_EDGE ( 'NONE', *, *, #43329, .F. ) ;
#91708=CARTESIAN_POINT ( 'NONE',  ( 154.8793480878393041, 20.01712742760162200, 11.60576973085460040 ) ) ;
#91715=LINE ( 'NONE', #41519, #10997 ) ;
#91717=CARTESIAN_POINT ( 'NONE',  ( 195.3024354219830911, 42.05395879699454298, 13.15751923266871870 ) ) ;
#91719=ORIENTED_EDGE ( 'NONE', *, *, #55843, .T. ) ;
#91723=EDGE_CURVE ( 'NONE', #69962, #25512, #14629, .T. ) ;
#91738=DIRECTION ( 'NONE',  ( 0.000000000000000000, 0.000000000000000000, 1.000000000000000000 ) ) ;
#91760=CARTESIAN_POINT ( 'NONE',  ( 0.000000000000000000, 0.000000000000000000, -12.50000000000000000 ) ) ;
#91763=CARTESIAN_POINT ( 'NONE',  ( 195.2279938257249228, 39.55206589069444334, 15.00421968542118911 ) ) ;
#91772=CARTESIAN_POINT ( 'NONE',  ( 152.4883615486727990, 19.90193753872963711, 8.271207965229679715 ) ) ;
#91784=ORIENTED_EDGE ( 'NONE', *, *, #54006, .T. ) ;
#91797=LINE ( 'NONE', #19371, #77551 ) ;
#91798=CARTESIAN_POINT ( 'NONE',  ( 196.1155190967640465, 73.07272925554217124, -11.82469951281970566 ) ) ;
#91799=CARTESIAN_POINT ( 'NONE',  ( 195.0811277904324754, 250.0000000000000568, 15.19607843137254477 ) ) ;
#91832=ORIENTED_EDGE ( 'NONE', *, *, #89671, .F. ) ;
#91833=CYLINDRICAL_SURFACE ( 'NONE', #79150, 25.00000000000000000 ) ;
#91848=EDGE_CURVE ( 'NONE', #5104, #45831, #36385, .T. ) ;
#91854=ADVANCED_FACE ( 'NONE', ( #28828 ), #50601, .T. ) ;
#91880=ORIENTED_EDGE ( 'NONE', *, *, #66944, .T. ) ;
#91881=CARTESIAN_POINT ( 'NONE',  ( 186.6539576904058890, 293.9636489450775230, 11.60392986742922439 ) ) ;
#91883=DIRECTION ( 'NONE',  ( 0.000000000000000000, 0.000000000000000000, 1.000000000000000000 ) ) ;
#91895=CARTESIAN_POINT ( 'NONE',  ( 165.2494399300530290, 8.542400036368780647, 9.000000000000001776 ) ) ;
#91897=CIRCLE ( 'NONE', #73809, 4.000000000000003553 ) ;
#91910=ORIENTED_EDGE ( 'NONE', *, *, #28072, .F. ) ;
#91912=ORIENTED_EDGE ( 'NONE', *, *, #38745, .F. ) ;
#91921=ORIENTED_EDGE ( 'NONE', *, *, #59069, .T. ) ;
#91934=ORIENTED_EDGE ( 'NONE', *, *, #74810, .F. ) ;
#91941=ORIENTED_EDGE ( 'NONE', *, *, #52236, .F. ) ;
#91942=PLANE ( 'NONE',  #18566 ) ;
#91947=EDGE_CURVE ( 'NONE', #8082, #18551, #85577, .T. ) ;
#91954=CARTESIAN_POINT ( 'NONE',  ( 200.8419735307467420, 26.78103457774642138, 10.49999999999999822 ) ) ;
#91960=CARTESIAN_POINT ( 'NONE',  ( 208.8044539878574426, 30.13468703429182227, 15.11452430534868618 ) ) ;
#91971=CARTESIAN_POINT ( 'NONE',  ( 175.2296996224750103, 20.99999999999998934, 0.000000000000000000 ) ) ;
#91972=CIRCLE ( 'NONE', #46612, 1.000000000000000888 ) ;
#91979=CARTESIAN_POINT ( 'NONE',  ( 193.1191634708854110, 250.0000000000000000, 16.90039380915348843 ) ) ;
#91983=CARTESIAN_POINT ( 'NONE',  ( 207.6175730408114930, 30.32598770090644180, 14.41714557868295898 ) ) ;
#91986=CARTESIAN_POINT ( 'NONE',  ( 158.9078607026220595, 17.25638377771136334, -9.432942837125283475 ) ) ;
#91996=EDGE_LOOP ( 'NONE', ( #15269, #44787, #37744, #7698 ) ) ;
#91999=CARTESIAN_POINT ( 'NONE',  ( 209.5646630284975629, 29.26077267968336315, 13.08022668053246740 ) ) ;
#92003=CARTESIAN_POINT ( 'NONE',  ( 196.8803347170859865, 73.40565171261609123, 12.49999999999999289 ) ) ;
#92039=ADVANCED_FACE ( 'NONE', ( #15074 ), #3945, .T. ) ;
#92043=TOROIDAL_SURFACE ( 'NONE', #61845, 1.000000000000000000, 0.5000000000000000000 ) ;
#92055=ORIENTED_EDGE ( 'NONE', *, *, #24425, .F. ) ;
#92071=CARTESIAN_POINT ( 'NONE',  ( 208.6208076322478746, 32.98517505407394168, 10.50000000000000000 ) ) ;
#92083=CARTESIAN_POINT ( 'NONE',  ( 175.2296996224750103, 215.0000000000000568, 0.000000000000000000 ) ) ;
#92092=CARTESIAN_POINT ( 'NONE',  ( 193.5659903145831038, 249.5000000000000568, 16.24901362097127233 ) ) ;
#92096=FACE_OUTER_BOUND ( 'NONE', #35918, .T. ) ;
#92101=EDGE_CURVE ( 'NONE', #28861, #53738, #10278, .T. ) ;
#92111=CARTESIAN_POINT ( 'NONE',  ( 0.000000000000000000, 131.0000000000000568, 11.50000000000000000 ) ) ;
#92131=CARTESIAN_POINT ( 'NONE',  ( 155.6265766802846713, 17.98195150565417322, 10.85854113850158953 ) ) ;
#92141=ORIENTED_EDGE ( 'NONE', *, *, #19203, .T. ) ;
#92142=EDGE_LOOP ( 'NONE', ( #13678, #41989, #67012, #27215 ) ) ;
#92153=CARTESIAN_POINT ( 'NONE',  ( 150.6539576904058606, 293.9636489450775230, 0.000000000000000000 ) ) ;
#92157=ORIENTED_EDGE ( 'NONE', *, *, #56521, .T. ) ;
#92166=ORIENTED_EDGE ( 'NONE', *, *, #26705, .F. ) ;
#92175=DIRECTION ( 'NONE',  ( 0.000000000000000000, 0.000000000000000000, -1.000000000000000000 ) ) ;
#92182=CARTESIAN_POINT ( 'NONE',  ( 208.0212563688061209, 27.56882951438707607, 12.00000000000000000 ) ) ;
#92185=EDGE_LOOP ( 'NONE', ( #90490, #89313, #83368, #49780 ) ) ;
#92186=ORIENTED_EDGE ( 'NONE', *, *, #42456, .F. ) ;
#92187=CARTESIAN_POINT ( 'NONE',  ( 201.2104617360081704, 25.32700003806615641, 10.50000000000000000 ) ) ;
#92201=CARTESIAN_POINT ( 'NONE',  ( 196.0602364706492153, 26.06347922710755327, 13.31833675859200916 ) ) ;
#92216=FACE_OUTER_BOUND ( 'NONE', #54105, .T. ) ;
#92218=DIRECTION ( 'NONE',  ( -5.551115123125793746E-15, 0.000000000000000000, 1.000000000000000000 ) ) ;
#92229=CARTESIAN_POINT ( 'NONE',  ( 199.0061125298537377, 249.5000000000000568, -7.725424859374024678 ) ) ;
#92235=CIRCLE ( 'NONE', #75548, 0.5000000000000004441 ) ;
#92238=ORIENTED_EDGE ( 'NONE', *, *, #35647, .T. ) ;
#92240=DIRECTION ( 'NONE',  ( 0.000000000000000000, 0.000000000000000000, -1.000000000000000000 ) ) ;
#92252=CARTESIAN_POINT ( 'NONE',  ( 195.5098343408735957, 40.18270620362346079, 13.84004740867598393 ) ) ;
#92255=CARTESIAN_POINT ( 'NONE',  ( 200.4551663813218170, 64.49084098419280053, -5.329070518200752656E-14 ) ) ;
#92257=ORIENTED_EDGE ( 'NONE', *, *, #61720, .T. ) ;
#92263=CARTESIAN_POINT ( 'NONE',  ( 197.0949311480472659, 69.78325229578651090, -10.59408097397595405 ) ) ;
#92264=CARTESIAN_POINT ( 'NONE',  ( 140.6539576904058606, 275.5000000000000568, 12.50000000000000000 ) ) ;
#92265=DIRECTION ( 'NONE',  ( 1.000000000000000000, 0.000000000000000000, 0.000000000000000000 ) ) ;
#92268=EDGE_CURVE ( 'NONE', #28384, #75749, #30980, .T. ) ;
#92275=ORIENTED_EDGE ( 'NONE', *, *, #6687, .F. ) ;
#92298=ORIENTED_EDGE ( 'NONE', *, *, #17686, .F. ) ;
#92299=ORIENTED_EDGE ( 'NONE', *, *, #84612, .T. ) ;
#92313=CIRCLE ( 'NONE', #40852, 24.00000000000000355 ) ;
#92317=CARTESIAN_POINT ( 'NONE',  ( 196.8409580319986674, 73.46773880466290052, -12.56795567929779445 ) ) ;
#92318=CARTESIAN_POINT ( 'NONE',  ( 180.6209651459523968, 275.5000000000000568, -24.41176470588238345 ) ) ;
#92327=DIRECTION ( 'NONE',  ( 1.000000000000000000, 0.000000000000000000, 0.000000000000000000 ) ) ;
#92348=ORIENTED_EDGE ( 'NONE', *, *, #84321, .T. ) ;
#92349=DIRECTION ( 'NONE',  ( -0.000000000000000000, 1.000000000000000000, -9.656854691831248164E-17 ) ) ;
#92363=DIRECTION ( 'NONE',  ( 0.000000000000000000, 0.000000000000000000, 1.000000000000000000 ) ) ;
#92364=CARTESIAN_POINT ( 'NONE',  ( 151.9232213214486649, 19.99481389066561121, -6.233836834234008251 ) ) ;
#92370=EDGE_CURVE ( 'NONE', #3752, #15791, #8003, .T. ) ;
#92379=ORIENTED_EDGE ( 'NONE', *, *, #53825, .F. ) ;
#92408=ORIENTED_EDGE ( 'NONE', *, *, #28179, .T. ) ;
#92409=CARTESIAN_POINT ( 'NONE',  ( 208.4306832106271088, -74.55766379199613425, -7.500000000000013323 ) ) ;
#92419=DIRECTION ( 'NONE',  ( -1.000000000000000000, 0.000000000000000000, 0.000000000000000000 ) ) ;
#92439=VECTOR ( 'NONE', #74049, 1000.000000000000000 ) ;
#92447=DIRECTION ( 'NONE',  ( 0.000000000000000000, 1.000000000000000000, 0.000000000000000000 ) ) ;
#92464=ORIENTED_EDGE ( 'NONE', *, *, #5711, .T. ) ;
#92480=CARTESIAN_POINT ( 'NONE',  ( 154.6618932926284913, 20.39585521906777643, -12.36951983184901493 ) ) ;
#92496=EDGE_LOOP ( 'NONE', ( #66437, #43230, #74966, #36154 ) ) ;
#92508=CIRCLE ( 'NONE', #75887, 1.000000000000000888 ) ;
#92511=TOROIDAL_SURFACE ( 'NONE', #35072, 5.603083949679977138, 1.500000000000000000 ) ;
#92519=ORIENTED_EDGE ( 'NONE', *, *, #35848, .T. ) ;
#92526=EDGE_LOOP ( 'NONE', ( #5788, #28170, #18824, #89565 ) ) ;
#92528=EDGE_LOOP ( 'NONE', ( #32109, #21138, #25734, #6830 ) ) ;
#92535=CARTESIAN_POINT ( 'NONE',  ( 152.8567950062365242, 19.85971597382232190, -11.17893457255801337 ) ) ;
#92540=DIRECTION ( 'NONE',  ( 1.000000000000000000, 0.000000000000000000, -0.000000000000000000 ) ) ;
#92555=CARTESIAN_POINT ( 'NONE',  ( 207.7524637998687638, 30.27509731313811869, 14.39153753875996244 ) ) ;
#92569=AXIS2_PLACEMENT_3D ( 'NONE', #23055, #51933, #80823 ) ;
#92573=DIRECTION ( 'NONE',  ( -0.000000000000000000, -0.000000000000000000, 1.000000000000000000 ) ) ;
#92578=CARTESIAN_POINT ( 'NONE',  ( 175.2296996224750103, 154.6894116713782807, -24.16304133878946558 ) ) ;
#92581=VECTOR ( 'NONE', #2905, 1000.000000000000000 ) ;
#92606=ORIENTED_EDGE ( 'NONE', *, *, #68122, .F. ) ;
#92618=DIRECTION ( 'NONE',  ( -0.9531768234071978929, 0.3024135303179465439, 0.000000000000000000 ) ) ;
#92619=FACE_OUTER_BOUND ( 'NONE', #8916, .T. ) ;
#92636=DIRECTION ( 'NONE',  ( -0.6056179655966478226, 0.7957555401921982963, 0.000000000000000000 ) ) ;
#92637=CARTESIAN_POINT ( 'NONE',  ( 197.2558782386354892, 42.34377483820648536, 11.92135876141209394 ) ) ;
#92641=AXIS2_PLACEMENT_3D ( 'NONE', #63114, #19520, #20476 ) ;
#92647=VECTOR ( 'NONE', #36568, 1000.000000000000000 ) ;
#92648=DIRECTION ( 'NONE',  ( 0.000000000000000000, -1.000000000000000000, -0.000000000000000000 ) ) ;
#92649=DIRECTION ( 'NONE',  ( 0.000000000000000000, 0.000000000000000000, -1.000000000000000000 ) ) ;
#92653=ORIENTED_EDGE ( 'NONE', *, *, #54065, .F. ) ;
#92654=CYLINDRICAL_SURFACE ( 'NONE', #3565, 4.000000000000003553 ) ;
#92668=DIRECTION ( 'NONE',  ( 0.2916739763039743472, 0.000000000000000000, 0.9565177946839404921 ) ) ;
#92669=CARTESIAN_POINT ( 'NONE',  ( 175.2296996224750103, 275.0000000000000568, 24.00000000000000355 ) ) ;
#92671=CIRCLE ( 'NONE', #6524, 3.842139515347647638 ) ;
#92683=ADVANCED_FACE ( 'NONE', ( #75165 ), #46721, .F. ) ;
#92687=CARTESIAN_POINT ( 'NONE',  ( 219.8344101925596021, 35.72494958537217968, -10.00000000000000000 ) ) ;
#92696=PLANE ( 'NONE',  #60832 ) ;
#92700=CARTESIAN_POINT ( 'NONE',  ( 195.0937532148314233, 39.77461757279066035, 15.17963093583605705 ) ) ;
#92708=ADVANCED_FACE ( 'NONE', ( #11229 ), #69000, .F. ) ;
#92709=AXIS2_PLACEMENT_3D ( 'NONE', #41783, #59160, #8019 ) ;
#92711=VERTEX_POINT ( 'NONE', #24978 ) ;
#92712=CARTESIAN_POINT ( 'NONE',  ( 153.4245301327627828, 19.61868323047014329, 10.85241966622267462 ) ) ;
#92715=CARTESIAN_POINT ( 'NONE',  ( 208.9486937585552937, 28.83547737520457588, 12.90287354992395130 ) ) ;
#92724=VERTEX_POINT ( 'NONE', #82259 ) ;
#92728=AXIS2_PLACEMENT_3D ( 'NONE', #17696, #74995, #24314 ) ;
#92730=EDGE_LOOP ( 'NONE', ( #13007, #13694, #93221, #6741, #55252, #37792, #88671, #84151, #63232, #50830, #25401, #24696, #30771, #150, #83305, #882, #82552, #56914, #42894, #80491, #60297, #78430, #12915, #68093, #78229 ) ) ;
#92736=CARTESIAN_POINT ( 'NONE',  ( 198.3166830480494411, 65.26573560487175030, -9.728010558291394716 ) ) ;
#92737=AXIS2_PLACEMENT_3D ( 'NONE', #459, #28416, #63486 ) ;
#92738=DIRECTION ( 'NONE',  ( 0.000000000000000000, 0.000000000000000000, -1.000000000000000000 ) ) ;
#92742=ORIENTED_EDGE ( 'NONE', *, *, #71254, .F. ) ;
#92757=EDGE_CURVE ( 'NONE', #77857, #16264, #84081, .T. ) ;
#92775=ORIENTED_EDGE ( 'NONE', *, *, #28532, .F. ) ;
#92776=CARTESIAN_POINT ( 'NONE',  ( 186.2362647323748206, 250.0000000000000568, 22.80382896336985965 ) ) ;
#92785=CIRCLE ( 'NONE', #80683, 25.00000000000000355 ) ;
#92792=CARTESIAN_POINT ( 'NONE',  ( 189.9243309297870610, 215.0000000000000568, 20.22542485937349355 ) ) ;
#92800=AXIS2_PLACEMENT_3D ( 'NONE', #35642, #7220, #64559 ) ;
#92801=VECTOR ( 'NONE', #55262, 1000.000000000000000 ) ;
#92803=CARTESIAN_POINT ( 'NONE',  ( 197.1933712184921603, 24.89666632552609826, 12.64285714285712992 ) ) ;
#92805=DIRECTION ( 'NONE',  ( 0.9531768234071978929, -0.3024135303179465439, 0.000000000000000000 ) ) ;
#92808=VECTOR ( 'NONE', #44363, 1000.000000000000000 ) ;
#92815=EDGE_CURVE ( 'NONE', #65891, #31, #18880, .T. ) ;
#92817=CARTESIAN_POINT ( 'NONE',  ( 205.2296996224750103, 68.12454877777268791, 0.000000000000000000 ) ) ;
#92819=CARTESIAN_POINT ( 'NONE',  ( 197.1181226030119262, 72.74206317236959762, -12.08813930015187488 ) ) ;
#92829=VERTEX_POINT ( 'NONE', #69456 ) ;
#92830=CYLINDRICAL_SURFACE ( 'NONE', #58939, 7.500000000000013323 ) ;
#92844=FACE_OUTER_BOUND ( 'NONE', #88328, .T. ) ;
#92848=VECTOR ( 'NONE', #29580, 1000.000000000000000 ) ;
#92853=AXIS2_PLACEMENT_3D ( 'NONE', #88944, #15599, #59163 ) ;
#92859=VERTEX_POINT ( 'NONE', #27309 ) ;
#92861=ORIENTED_EDGE ( 'NONE', *, *, #27400, .T. ) ;
#92863=AXIS2_PLACEMENT_3D ( 'NONE', #67667, #52971, #2793 ) ;
#92865=VECTOR ( 'NONE', #23236, 1000.000000000000000 ) ;
#92870=EDGE_LOOP ( 'NONE', ( #80852, #20107, #57715, #8161 ) ) ;
#92878=CARTESIAN_POINT ( 'NONE',  ( 158.6539576904058606, 293.9636489450775230, 0.000000000000000000 ) ) ;
#92890=ADVANCED_FACE ( 'NONE', ( #92619 ), #13123, .T. ) ;
#92894=CARTESIAN_POINT ( 'NONE',  ( 194.4923472626465752, 26.08759934769913258, 14.31634348551539659 ) ) ;
#92920=DIRECTION ( 'NONE',  ( 0.000000000000000000, 0.000000000000000000, 1.000000000000000000 ) ) ;
#92926=ADVANCED_FACE ( 'NONE', ( #27790 ), #56196, .F. ) ;
#92927=CARTESIAN_POINT ( 'NONE',  ( 185.2519943799831879, 3.000000000000000000, 10.00000000000000000 ) ) ;
#92929=DIRECTION ( 'NONE',  ( -0.000000000000000000, -0.000000000000000000, -1.000000000000000000 ) ) ;
#92931=CARTESIAN_POINT ( 'NONE',  ( 157.7238125175282732, 19.47471017779399105, -10.32097897594415592 ) ) ;
#92934=CARTESIAN_POINT ( 'NONE',  ( 164.2231345125756263, 249.5000000000000568, 22.80382896337008702 ) ) ;
#92941=AXIS2_PLACEMENT_3D ( 'NONE', #44015, #79566, #43562 ) ;
#92945=ORIENTED_EDGE ( 'NONE', *, *, #10705, .F. ) ;
#92948=DIRECTION ( 'NONE',  ( 0.000000000000000000, 1.000000000000000000, 0.000000000000000000 ) ) ;
#92950=ORIENTED_EDGE ( 'NONE', *, *, #75324, .F. ) ;
#92967=DIRECTION ( 'NONE',  ( 0.000000000000000000, 0.000000000000000000, 1.000000000000000000 ) ) ;
#92975=CARTESIAN_POINT ( 'NONE',  ( 157.5411741086738004, 275.0000000000000568, 16.22085278731064761 ) ) ;
#92985=ORIENTED_EDGE ( 'NONE', *, *, #36695, .F. ) ;
#93003=ORIENTED_EDGE ( 'NONE', *, *, #59598, .F. ) ;
#93009=ORIENTED_EDGE ( 'NONE', *, *, #57561, .F. ) ;
#93010=CIRCLE ( 'NONE', #52169, 5.568361562975243650 ) ;
#93018=CIRCLE ( 'NONE', #38529, 0.5000000000000004441 ) ;
#93023=CIRCLE ( 'NONE', #24964, 25.00000000000000355 ) ;
#93040=CARTESIAN_POINT ( 'NONE',  ( 165.2494399300530290, 8.542400036368780647, 9.974999999999996092 ) ) ;
#93044=CARTESIAN_POINT ( 'NONE',  ( 199.1087447750284980, 64.61450673763175701, -10.46317447812566570 ) ) ;
#93048=EDGE_CURVE ( 'NONE', #4223, #27414, #37191, .T. ) ;
#93058=CARTESIAN_POINT ( 'NONE',  ( 209.3354045562396379, 36.47363971095035140, 13.48243931971275167 ) ) ;
#93061=CARTESIAN_POINT ( 'NONE',  ( 169.9462594094670180, 275.5000000000000568, -23.92352941176469727 ) ) ;
#93067=EDGE_CURVE ( 'NONE', #91019, #26459, #61407, .T. ) ;
#93087=CIRCLE ( 'NONE', #3867, 0.5000000000000003331 ) ;
#93090=EDGE_LOOP ( 'NONE', ( #72130, #89577 ) ) ;
#93099=DIRECTION ( 'NONE',  ( 0.9764705882352963107, -0.000000000000000000, 0.2156506209390885997 ) ) ;
#93100=DIRECTION ( 'NONE',  ( 0.000000000000000000, 0.000000000000000000, 1.000000000000000000 ) ) ;
#93104=VERTEX_POINT ( 'NONE', #33461 ) ;
#93112=VERTEX_POINT ( 'NONE', #19268 ) ;
#93116=ORIENTED_EDGE ( 'NONE', *, *, #68258, .F. ) ;
#93117=DIRECTION ( 'NONE',  ( 0.000000000000000000, 0.000000000000000000, -1.000000000000000000 ) ) ;
#93118=CARTESIAN_POINT ( 'NONE',  ( 196.0143093133015384, 73.40565171261609123, -11.99999999999998046 ) ) ;
#93125=CARTESIAN_POINT ( 'NONE',  ( 202.4316997032785537, 63.54496854667812755, -6.999999999999996447 ) ) ;
#93127=ORIENTED_EDGE ( 'NONE', *, *, #51125, .T. ) ;
#93128=ORIENTED_EDGE ( 'NONE', *, *, #78174, .T. ) ;
#93129=CARTESIAN_POINT ( 'NONE',  ( 208.3305877567938751, 27.64722171545246709, 11.99999999999999822 ) ) ;
#93144=CARTESIAN_POINT ( 'NONE',  ( 195.4479150618181791, 27.22655798642326985, 13.98918657931467635 ) ) ;
#93147=AXIS2_PLACEMENT_3D ( 'NONE', #41114, #43031, #70046 ) ;
#93160=EDGE_CURVE ( 'NONE', #12543, #27549, #93018, .T. ) ;
#93163=B_SPLINE_CURVE_WITH_KNOTS ( 'NONE', 3,
 ( #10571, #25258, #83004, #92927 ),
 .UNSPECIFIED., .F., .F.,
 ( 4, 4 ),
 ( 0.000000000000000000, 1.000000000000000000 ),
 .UNSPECIFIED. ) ;
#93171=CARTESIAN_POINT ( 'NONE',  ( 209.2568086740256206, 34.98978593258855341, 14.00000000000000000 ) ) ;
#93178=CARTESIAN_POINT ( 'NONE',  ( 164.2231345125756263, 264.6571197653884155, -7.500000000000000000 ) ) ;
#93187=ORIENTED_EDGE ( 'NONE', *, *, #48476, .F. ) ;
#93188=CARTESIAN_POINT ( 'NONE',  ( 151.6573119020196145, 20.00000000000000000, 4.897109440894215737 ) ) ;
#93200=CARTESIAN_POINT ( 'NONE',  ( 175.2296996224750103, 250.0000000000000568, 0.000000000000000000 ) ) ;
#93205=ORIENTED_EDGE ( 'NONE', *, *, #82436, .F. ) ;
#93213=CARTESIAN_POINT ( 'NONE',  ( 199.9311642430735105, 312.1715086799357550, -9.103929867429124911 ) ) ;
#93221=ORIENTED_EDGE ( 'NONE', *, *, #5681, .T. ) ;
#93228=EDGE_CURVE ( 'NONE', #15791, #57748, #24956, .T. ) ;
#93246=ORIENTED_EDGE ( 'NONE', *, *, #49257, .T. ) ;
#93248=DIRECTION ( 'NONE',  ( 0.000000000000000000, 1.000000000000000000, 0.000000000000000000 ) ) ;
#93262=DIRECTION ( 'NONE',  ( 0.000000000000000000, 1.000000000000000000, 0.000000000000000000 ) ) ;
#93263=CARTESIAN_POINT ( 'NONE',  ( 197.2116943569230330, 275.5000000000000568, -12.92446933126074882 ) ) ;
#93273=FACE_OUTER_BOUND ( 'NONE', #87403, .T. ) ;
#93275=FACE_OUTER_BOUND ( 'NONE', #12412, .T. ) ;
#93284=DIRECTION ( 'NONE',  ( -0.000000000000000000, -1.000000000000000000, -0.000000000000000000 ) ) ;
#93286=EDGE_CURVE ( 'NONE', #1451, #20790, #32825, .T. ) ;
#93287=CARTESIAN_POINT ( 'NONE',  ( 198.6673011211816515, 69.03676313268820763, -9.597248819411134946 ) ) ;
#93302=DIRECTION ( 'NONE',  ( 0.000000000000000000, 0.000000000000000000, 1.000000000000000000 ) ) ;
#93314=CARTESIAN_POINT ( 'NONE',  ( 201.6445761222588544, 62.92800856396105047, -6.999999999998341771 ) ) ;
#93327=VERTEX_POINT ( 'NONE', #71341 ) ;
#93332=B_SPLINE_CURVE_WITH_KNOTS ( 'NONE', 3,
 ( #83698, #90324, #55316, #18860, #47717, #46771, #19778, #84167, #76617, #40593, #69507, #82768, #4638, #33998, #33512, #47235 ),
 .UNSPECIFIED., .F., .F.,
 ( 4, 2, 2, 2, 2, 2, 2, 4 ),
 ( 0.000000000000000000, 0.0007636009008559850987, 0.001145401351284006108, 0.001527201801712027227, 0.001909002252140048128, 0.002290802702568069029, 0.002672603152996090147, 0.003054403603424111265 ),
 .UNSPECIFIED. ) ;
#93335=ORIENTED_EDGE ( 'NONE', *, *, #34144, .T. ) ;
#93342=CARTESIAN_POINT ( 'NONE',  ( 196.8803347170859865, 42.36571313990103249, 12.49999999999999289 ) ) ;
#93355=CARTESIAN_POINT ( 'NONE',  ( 194.7518928364593478, 26.86155445384702034, 13.97733162193927114 ) ) ;
#93383=CARTESIAN_POINT ( 'NONE',  ( 169.2494399300530290, 8.542400036368780647, 9.000000000000001776 ) ) ;
#93389=FACE_OUTER_BOUND ( 'NONE', #77177, .T. ) ;
#93390=FACE_OUTER_BOUND ( 'NONE', #14139, .T. ) ;
#93392=LINE ( 'NONE', #56978, #63363 ) ;
#93395=FACE_OUTER_BOUND ( 'NONE', #19491, .T. ) ;
#93396=CARTESIAN_POINT ( 'NONE',  ( 159.0442047513579951, 16.98551211945800432, -9.330684800570146820 ) ) ;
#93406=ORIENTED_EDGE ( 'NONE', *, *, #73224, .T. ) ;
#93409=CARTESIAN_POINT ( 'NONE',  ( 183.0442525570908288, 300.2961574867697436, 4.888549259831427740 ) ) ;
#93427=FACE_OUTER_BOUND ( 'NONE', #3090, .T. ) ;
#93441=ORIENTED_EDGE ( 'NONE', *, *, #41040, .T. ) ;
#93444=ORIENTED_EDGE ( 'NONE', *, *, #19910, .F. ) ;
#93470=EDGE_LOOP ( 'NONE', ( #68909, #4601, #3435 ) ) ;
#93482=CARTESIAN_POINT ( 'NONE',  ( 209.7513585654922679, 305.7026273589066818, -40.00000000000000711 ) ) ;
#93493=DIRECTION ( 'NONE',  ( 1.000000000000000000, 0.000000000000000000, -0.000000000000000000 ) ) ;
#93497=LINE ( 'NONE', #64207, #42897 ) ;
#93503=CARTESIAN_POINT ( 'NONE',  ( 197.8479349096537874, 68.18631839859101262, -11.29146348611214812 ) ) ;
#93529=CIRCLE ( 'NONE', #90457, 4.999999999999993783 ) ;
#93547=EDGE_CURVE ( 'NONE', #21018, #4210, #10647, .T. ) ;
#93553=DIRECTION ( 'NONE',  ( -0.000000000000000000, 1.000000000000000000, -0.000000000000000000 ) ) ;
#93562=EDGE_CURVE ( 'NONE', #71446, #26935, #69226, .T. ) ;
#93571=DIRECTION ( 'NONE',  ( 0.000000000000000000, 0.000000000000000000, -1.000000000000000000 ) ) ;
#93572=DIRECTION ( 'NONE',  ( 0.000000000000000000, 1.000000000000000000, 0.000000000000000000 ) ) ;
#93580=CARTESIAN_POINT ( 'NONE',  ( 208.6515845757822092, 29.54020560868483614, 14.79569954156320755 ) ) ;
#93581=DIRECTION ( 'NONE',  ( 0.000000000000000000, 0.000000000000000000, -1.000000000000000000 ) ) ;
#93586=LINE ( 'NONE', #86471, #15669 ) ;
#93593=CIRCLE ( 'NONE', #72467, 0.4999999999999989453 ) ;
#93601=CARTESIAN_POINT ( 'NONE',  ( 201.2104617360081704, 41.21457449016151031, 10.50000000000000000 ) ) ;
#93602=DIRECTION ( 'NONE',  ( -0.000000000000000000, -1.000000000000000000, -0.000000000000000000 ) ) ;
#93615=CARTESIAN_POINT ( 'NONE',  ( 152.2746432211103809, 129.8137309627706202, -12.50000000000000178 ) ) ;
#93617=CARTESIAN_POINT ( 'NONE',  ( 196.2438553357862077, 20.66497315817206015, 13.54628071421389102 ) ) ;
#93624=CARTESIAN_POINT ( 'NONE',  ( 140.6539576904058606, 250.0000000000000568, 10.50000000000000000 ) ) ;
#93627=CARTESIAN_POINT ( 'NONE',  ( 205.7381008070598227, 1.000000000000000888, 7.000000000000000000 ) ) ;
#93631=CARTESIAN_POINT ( 'NONE',  ( 152.4536156746142410, 130.6065089285656313, -11.50000000000000000 ) ) ;
#93642=DIRECTION ( 'NONE',  ( 0.000000000000000000, 1.000000000000000000, 0.000000000000000000 ) ) ;
#93644=CARTESIAN_POINT ( 'NONE',  ( 189.9243309297870610, 275.0000000000000568, 20.22542485937349355 ) ) ;
#93653=ORIENTED_EDGE ( 'NONE', *, *, #66553, .T. ) ;
#93654=CARTESIAN_POINT ( 'NONE',  ( 195.4548275740021666, 39.96818058921539318, 13.92024756609993119 ) ) ;
#93660=ADVANCED_FACE ( 'NONE', ( #69691 ), #20356, .T. ) ;
#93665=CIRCLE ( 'NONE', #52826, 4.499999999999986677 ) ;
#93669=DIRECTION ( 'NONE',  ( 8.659560562355067211E-17, -0.7071067811865364705, 0.7071067811865584529 ) ) ;
#93670=CARTESIAN_POINT ( 'NONE',  ( 138.6539576904058606, 132.0000000000000568, -10.49999999999999822 ) ) ;
#93690=ORIENTED_EDGE ( 'NONE', *, *, #92757, .T. ) ;
#93691=CARTESIAN_POINT ( 'NONE',  ( 157.4851178187871312, 69.18068689461284748, 7.000000000000000000 ) ) ;
#93704=VERTEX_POINT ( 'NONE', #68296 ) ;
#93706=FACE_OUTER_BOUND ( 'NONE', #11452, .T. ) ;
#93732=COLOUR_RGB('Light Blue',0.38,0.62,0.78);
#93733=FILL_AREA_STYLE_COLOUR('',#93732);
#93734=FILL_AREA_STYLE('',(#93733));
#93735=SURFACE_STYLE_FILL_AREA(#93734);
#93736=SURFACE_SIDE_STYLE('',(#93735));
#93737=SURFACE_STYLE_USAGE(.BOTH.,#93736);
#93738=PRESENTATION_STYLE_ASSIGNMENT((#93737));
ENDSEC;
END-ISO-10303-21;
